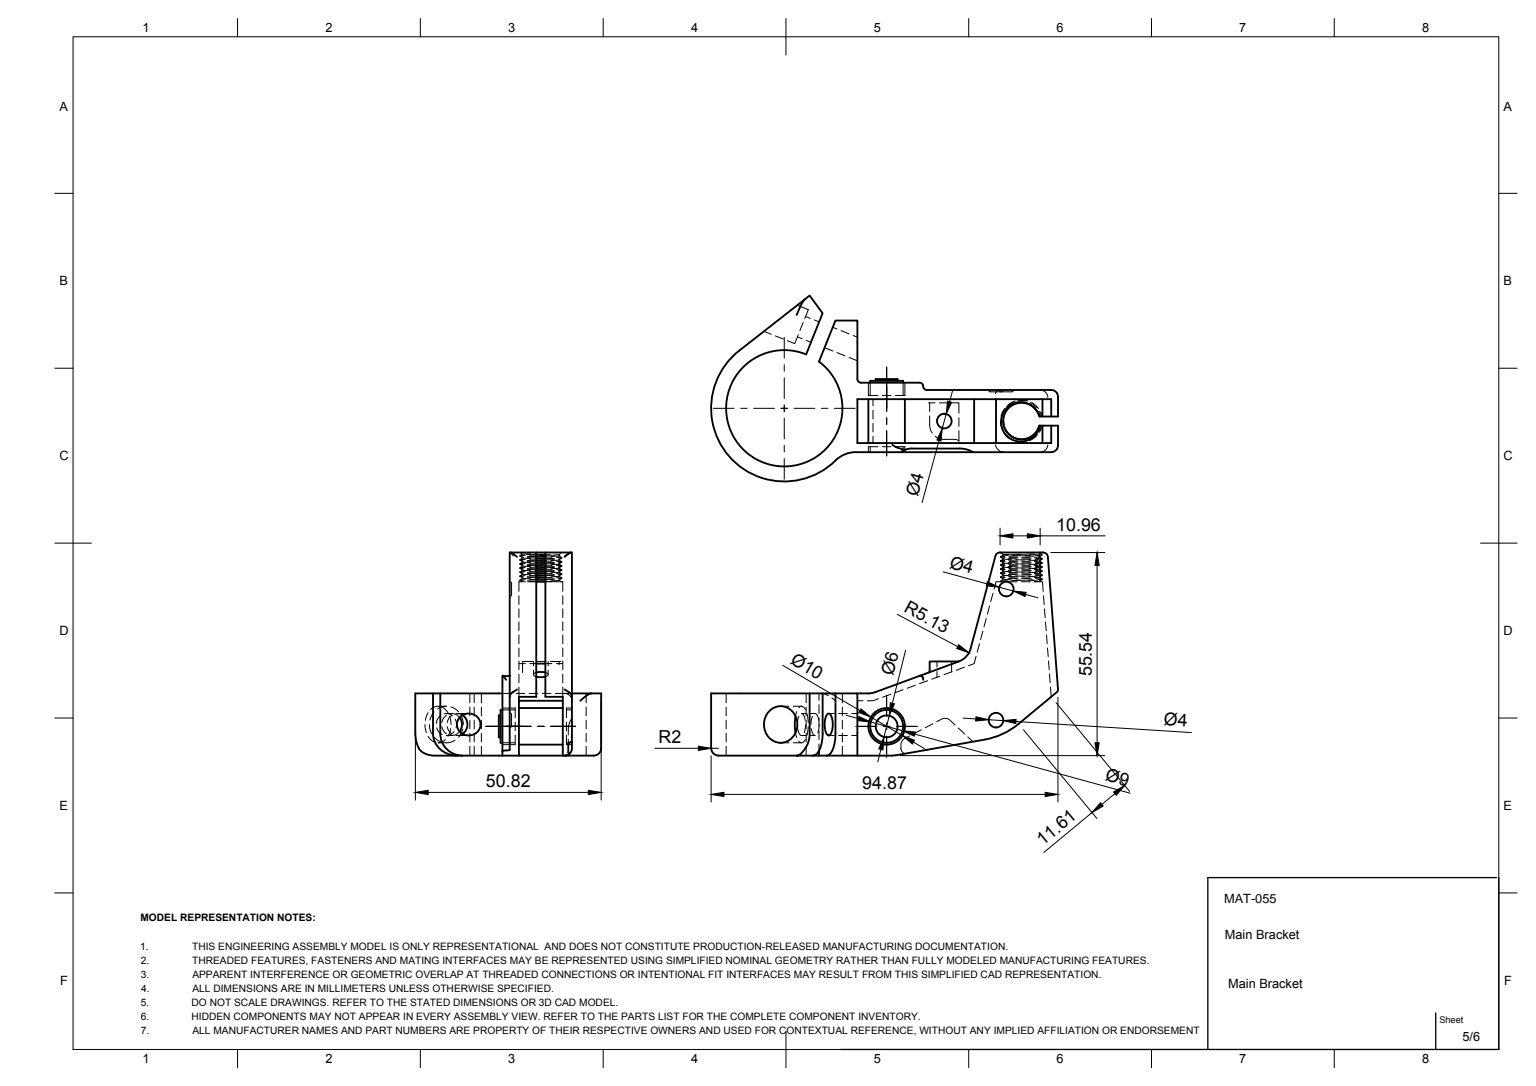
ISO-10303-21;
HEADER;
FILE_DESCRIPTION (('STEP AP214'),
    '1' );
FILE_NAME ('Main Bracket.step',
    '2026-10-30T09:41:00',
    ( '' ),
    ( '' ),
    'SwSTEP 2.0',
    'SolidWorks 2020',
    '' );
FILE_SCHEMA (( 'AUTOMOTIVE_DESIGN' ));
ENDSEC;

DATA;
#1=CARTESIAN_POINT ( 'NONE',  ( 110.9687390045248350, -9.868328341294098749, -11.32035403202665869 ) ) ;
#13=CARTESIAN_POINT ( 'NONE',  ( 69.69189222814998175, -41.76310523276723785, -24.39321520033831447 ) ) ;
#21=CARTESIAN_POINT ( 'NONE',  ( 106.2459265045248173, -7.250697342233347165, -19.15521520033831138 ) ) ;
#24=ORIENTED_EDGE ( 'NONE', *, *, #31128, .T. ) ;
#26=CYLINDRICAL_SURFACE ( 'NONE', #29939, 3.000000000000002665 ) ;
#41=CARTESIAN_POINT ( 'NONE',  ( 116.0834518517486771, -0.01906416985213849058, -12.14321520033831625 ) ) ;
#42=CARTESIAN_POINT ( 'NONE',  ( 106.5237390045248418, 0.8980012041604421569, -15.77991374673208469 ) ) ;
#43=CARTESIAN_POINT ( 'NONE',  ( 107.8433483795247838, -8.402594152722688392, -16.93181055722141792 ) ) ;
#44=CARTESIAN_POINT ( 'NONE',  ( 105.4819421295248247, 0.8980012041604618078, -13.39321520033831447 ) ) ;
#47=ORIENTED_EDGE ( 'NONE', *, *, #34668, .T. ) ;
#49=CARTESIAN_POINT ( 'NONE',  ( 111.3854577545248645, -7.250697342233347165, -7.631215200338321125 ) ) ;
#50=DIRECTION ( 'NONE',  ( 0.000000000000000000, 0.000000000000000000, -1.000000000000000000 ) ) ;
#55=CARTESIAN_POINT ( 'NONE',  ( 116.0388171295248014, -10.62599879583958540, -13.39321520033831447 ) ) ;
#56=CARTESIAN_POINT ( 'NONE',  ( 106.8710046295248759, -4.863998795839590272, -7.631215200338315796 ) ) ;
#57=ORIENTED_EDGE ( 'NONE', *, *, #39925, .T. ) ;
#62=CARTESIAN_POINT ( 'NONE',  ( 115.7610046295247912, -4.863998795839590272, -7.631215200338315796 ) ) ;
#63=CARTESIAN_POINT ( 'NONE',  ( 108.3295202545248657, 0.1403307496149616695, -11.32035403202665336 ) ) ;
#74=CARTESIAN_POINT ( 'NONE',  ( 112.6356140045247827, 0.1403307496149616695, -15.46607636864997204 ) ) ;
#85=CARTESIAN_POINT ( 'NONE',  ( 106.4542858795248179, -8.402594152722688392, -9.854619843455216355 ) ) ;
#88=AXIS2_PLACEMENT_3D ( 'NONE', #42203, #35787, #10965 ) ;
#91=CARTESIAN_POINT ( 'NONE',  ( 78.69189222814998175, -49.76310523276723785, -23.89321520033831803 ) ) ;
#92=ORIENTED_EDGE ( 'NONE', *, *, #23975, .F. ) ;
#96=CARTESIAN_POINT ( 'NONE',  ( 85.28386362106600416, -27.88924328735366132, -8.828750294274950505 ) ) ;
#98=EDGE_CURVE ( 'NONE', #12720, #5950, #1643, .T. ) ;
#100=ORIENTED_EDGE ( 'NONE', *, *, #14497, .T. ) ;
#103=CARTESIAN_POINT ( 'NONE',  ( 111.6632702545248605, -10.62599879583958717, -15.77991374673208469 ) ) ;
#108=CARTESIAN_POINT ( 'NONE',  ( 108.5378796295247810, -4.863998795839590272, -8.388885654883775800 ) ) ;
#109=DIRECTION ( 'NONE',  ( -1.000000000000000000, 0.000000000000000000, 0.000000000000000000 ) ) ;
#110=CARTESIAN_POINT ( 'NONE',  ( 109.2294422165998071, -3.102175910333654585, -18.18453611788106983 ) ) ;
#113=CARTESIAN_POINT ( 'NONE',  ( 107.0099108795247815, -8.938348069036489818, -9.318865927141430916 ) ) ;
#114=CARTESIAN_POINT ( 'NONE',  ( 115.2748327545248657, -6.936859964151250502, -8.388885654883777576 ) ) ;
#115=CARTESIAN_POINT ( 'NONE',  ( 111.3854577545248645, -7.250697342233347165, -7.631215200338321125 ) ) ;
#126=EDGE_CURVE ( 'NONE', #5046, #36034, #30866, .T. ) ;
#132=CARTESIAN_POINT ( 'NONE',  ( 114.7192077545248594, -7.250697342233347165, -7.631215200338321125 ) ) ;
#141=CARTESIAN_POINT ( 'NONE',  ( 111.1767004682428848, 0.5115630086001619059, -14.64321520033833757 ) ) ;
#142=CARTESIAN_POINT ( 'NONE',  ( 115.6915515045247531, -6.936859964151250502, -18.39754474579286025 ) ) ;
#148=ORIENTED_EDGE ( 'NONE', *, *, #1596, .T. ) ;
#155=CARTESIAN_POINT ( 'NONE',  ( 112.5661608795247872, -8.938348069036489818, -9.318865927141430916 ) ) ;
#158=CARTESIAN_POINT ( 'NONE',  ( 109.2294420414169451, -0.008529726858385754465, -11.21375788622608560 ) ) ;
#160=CARTESIAN_POINT ( 'NONE',  ( 107.0793640045248196, 0.1403307496149616695, -15.46607636864997204 ) ) ;
#164=CARTESIAN_POINT ( 'NONE',  ( 108.8851452545248151, 0.8980012041604421569, -11.00651665394454071 ) ) ;
#165=DIRECTION ( 'NONE',  ( -0.9970811988817434024, 0.07634843047859724008, 0.000000000000000000 ) ) ;
#174=CARTESIAN_POINT ( 'NONE',  ( 108.1906140045248037, 0.1403307496149616695, -15.46607636864997204 ) ) ;
#177=EDGE_LOOP ( 'NONE', ( #36537, #100, #20372, #6347 ) ) ;
#182=EDGE_LOOP ( 'NONE', ( #10317, #8710, #12538, #23742 ) ) ;
#183=CARTESIAN_POINT ( 'NONE',  ( 107.3571765045248299, -2.791137627527939813, -8.388885654883777576 ) ) ;
#202=CARTESIAN_POINT ( 'NONE',  ( 106.8015515045248378, -2.477300249445798297, -7.631215200338321125 ) ) ;
#212=EDGE_CURVE ( 'NONE', #32579, #21740, #16699, .T. ) ;
#213=CARTESIAN_POINT ( 'NONE',  ( 74.69189222814998175, -41.76310523276723785, -7.393215200338315363 ) ) ;
#217=CARTESIAN_POINT ( 'NONE',  ( 110.5520202545248054, 0.1403307496149616695, -11.32035403202665336 ) ) ;
#227=CYLINDRICAL_SURFACE ( 'NONE', #9190, 4.000000000000000000 ) ;
#229=ORIENTED_EDGE ( 'NONE', *, *, #20701, .T. ) ;
#231=CARTESIAN_POINT ( 'NONE',  ( 70.19189222814998175, -75.31442247550839397, -37.94335727672635983 ) ) ;
#235=ORIENTED_EDGE ( 'NONE', *, *, #33948, .T. ) ;
#236=ADVANCED_FACE ( 'NONE', ( #2543, #19428 ), #16245, .T. ) ;
#241=CARTESIAN_POINT ( 'NONE',  ( 77.77634386988368931, 3.254514819260763581, -19.39321520033831447 ) ) ;
#242=CARTESIAN_POINT ( 'NONE',  ( 110.1353015045248469, -2.477300249445798297, -7.631215200338321125 ) ) ;
#261=DIRECTION ( 'NONE',  ( 1.000000000000000000, 0.000000000000000000, 0.000000000000000000 ) ) ;
#262=CARTESIAN_POINT ( 'NONE',  ( 113.1217858795247935, -8.402594152722688392, -9.854619843455216355 ) ) ;
#264=CARTESIAN_POINT ( 'NONE',  ( 108.3989733795247759, -1.325403438956436419, -9.854619843455211026 ) ) ;
#265=CARTESIAN_POINT ( 'NONE',  ( 113.7468640045248236, 0.1403307496149616695, -15.46607636864997204 ) ) ;
#268=EDGE_LOOP ( 'NONE', ( #6034, #39667, #9832, #29930 ) ) ;
#270=CARTESIAN_POINT ( 'NONE',  ( 110.9687390045248350, 0.8980012041604421569, -15.77991374673208469 ) ) ;
#277=CARTESIAN_POINT ( 'NONE',  ( 115.2748327545248657, -2.477300249445798297, -19.15521520033831138 ) ) ;
#278=CARTESIAN_POINT ( 'NONE',  ( 114.7886608795247696, -1.325403438956436419, -16.93181055722141792 ) ) ;
#284=CARTESIAN_POINT ( 'NONE',  ( 113.3995983795247895, -0.7896495226426338832, -9.318865927141430916 ) ) ;
#285=CARTESIAN_POINT ( 'NONE',  ( 107.4960827545248350, -6.936859964151250502, -8.388885654883777576 ) ) ;
#289=ORIENTED_EDGE ( 'NONE', *, *, #44643, .F. ) ;
#295=EDGE_CURVE ( 'NONE', #33939, #11904, #44743, .T. ) ;
#296=CARTESIAN_POINT ( 'NONE',  ( 106.5931921295248372, 0.8980012041604618078, -13.39321520033831447 ) ) ;
#297=CARTESIAN_POINT ( 'NONE',  ( 110.9687390045248350, -9.868328341294098749, -11.32035403202665869 ) ) ;
#306=DIRECTION ( 'NONE',  ( 0.000000000000000000, 0.7876185884367599144, -0.6161630946014909904 ) ) ;
#307=CARTESIAN_POINT ( 'NONE',  ( 106.5931921295248372, -9.868328341294093420, -13.39321520033831447 ) ) ;
#316=LINE ( 'NONE', #14010, #39137 ) ;
#321=LINE ( 'NONE', #35409, #15967 ) ;
#322=CARTESIAN_POINT ( 'NONE',  ( 112.8439733795247832, -8.938348069036489818, -17.46756447353520159 ) ) ;
#327=CARTESIAN_POINT ( 'NONE',  ( 111.7327233795247849, -1.325403438956533675, -9.854619843455175499 ) ) ;
#328=CARTESIAN_POINT ( 'NONE',  ( 110.2047546295247855, -4.863998795839590272, -18.39754474579285315 ) ) ;
#331=CARTESIAN_POINT ( 'NONE',  ( 109.2294421564239713, -3.315832619059893460, -18.27430022661860676 ) ) ;
#333=CARTESIAN_POINT ( 'NONE',  ( 106.0375671295248310, -10.62599879583958540, -13.39321520033831447 ) ) ;
#334=CARTESIAN_POINT ( 'NONE',  ( 114.4413952545248350, -9.868328341294098749, -15.46607636864997204 ) ) ;
#335=CARTESIAN_POINT ( 'NONE',  ( 108.1906140045248463, -10.62599879583958717, -11.00651665394454604 ) ) ;
#336=CARTESIAN_POINT ( 'NONE',  ( 66.06194382436763135, -14.97931106434683635, -7.393215200338315363 ) ) ;
#338=CARTESIAN_POINT ( 'NONE',  ( 71.37572422742091760, -11.86958442233774313, -21.89321520033831447 ) ) ;
#341=EDGE_CURVE ( 'NONE', #2225, #6245, #14383, .T. ) ;
#351=EDGE_CURVE ( 'NONE', #29699, #30236, #16925, .T. ) ;
#353=CARTESIAN_POINT ( 'NONE',  ( 107.9128015045248219, -2.477300249445798297, -7.631215200338321125 ) ) ;
#354=B_SPLINE_CURVE_WITH_KNOTS ( 'NONE', 3,
 ( #21953, #36072, #29691, #15790, #25607, #25823, #22401, #36296, #1419, #40183 ),
 .UNSPECIFIED., .F., .F.,
 ( 4, 2, 2, 2, 4 ),
 ( 0.000000000000000000, 0.2500000000000000000, 0.5000000000000000000, 0.7500000000000000000, 1.000000000000000000 ),
 .UNSPECIFIED. ) ;
#356=FACE_OUTER_BOUND ( 'NONE', #44787, .T. ) ;
#360=CARTESIAN_POINT ( 'NONE',  ( 90.93679655599923706, -18.80572346544368756, -20.89321520033831447 ) ) ;
#363=CARTESIAN_POINT ( 'NONE',  ( 112.3324666496844912, 0.5600166689815611054, -12.14321520033829849 ) ) ;
#364=CARTESIAN_POINT ( 'NONE',  ( 114.4413952545248350, -9.868328341294098749, -15.46607636864997204 ) ) ;
#376=CARTESIAN_POINT ( 'NONE',  ( 116.3860827545247787, -6.936859964151250502, -8.388885654883777576 ) ) ;
#380=CARTESIAN_POINT ( 'NONE',  ( 114.3024890045248156, 0.8980012041604421569, -15.77991374673208469 ) ) ;
#386=CARTESIAN_POINT ( 'NONE',  ( 108.3295202545248657, 0.1403307496149616695, -11.32035403202665336 ) ) ;
#387=CARTESIAN_POINT ( 'NONE',  ( 117.1746850318387203, 1.411517391187495640, -21.51583517613059016 ) ) ;
#390=CARTESIAN_POINT ( 'NONE',  ( 112.4272546295247821, -4.863998795839590272, -7.631215200338315796 ) ) ;
#393=CARTESIAN_POINT ( 'NONE',  ( 117.2294421295247844, 1.035107641088057973, -21.89321520033831447 ) ) ;
#400=CARTESIAN_POINT ( 'NONE',  ( 106.7320983795247855, -8.402594152722688392, -16.93181055722141792 ) ) ;
#408=VERTEX_POINT ( 'NONE', #41764 ) ;
#409=CARTESIAN_POINT ( 'NONE',  ( 107.1488171295247867, 0.1403307496149613920, -13.39321520033831447 ) ) ;
#424=VERTEX_POINT ( 'NONE', #34228 ) ;
#426=CARTESIAN_POINT ( 'NONE',  ( 113.6079577545248043, -2.791137627527939813, -18.39754474579286025 ) ) ;
#428=DIRECTION ( 'NONE',  ( 8.673617379884029556E-16, 1.000000000000000000, 0.000000000000000000 ) ) ;
#438=CARTESIAN_POINT ( 'NONE',  ( 110.2742077545248094, -2.791137627527939813, -18.39754474579286025 ) ) ;
#449=CARTESIAN_POINT ( 'NONE',  ( 66.82415148905926117, -40.21211973637273474, -4.893215200338314474 ) ) ;
#450=CARTESIAN_POINT ( 'NONE',  ( 109.9649712410415816, 0.7607806665038616689, -12.14321520033831625 ) ) ;
#461=CARTESIAN_POINT ( 'NONE',  ( 108.8851452545248151, 0.8980012041604421569, -11.00651665394454071 ) ) ;
#465=AXIS2_PLACEMENT_3D ( 'NONE', #17179, #9891, #34693 ) ;
#466=CARTESIAN_POINT ( 'NONE',  ( 69.69189222814998175, -41.76310523276723785, -4.893215200338314474 ) ) ;
#484=CARTESIAN_POINT ( 'NONE',  ( 113.2606921295247702, -9.868328341294093420, -13.39321520033831447 ) ) ;
#485=CARTESIAN_POINT ( 'NONE',  ( 110.1353015045248469, -6.936859964151250502, -18.39754474579286025 ) ) ;
#486=CARTESIAN_POINT ( 'NONE',  ( 115.6915515045247531, -6.936859964151250502, -18.39754474579286025 ) ) ;
#492=CARTESIAN_POINT ( 'NONE',  ( 112.7745202545247878, -10.62599879583958717, -15.77991374673208469 ) ) ;
#499=CARTESIAN_POINT ( 'NONE',  ( 115.6915515045247531, -2.477300249445798297, -7.631215200338321125 ) ) ;
#500=CARTESIAN_POINT ( 'NONE',  ( 112.9134265045247645, -2.791137627527939813, -8.388885654883777576 ) ) ;
#506=CARTESIAN_POINT ( 'NONE',  ( 114.9970202545248412, -10.62599879583958717, -15.77991374673208469 ) ) ;
#507=CARTESIAN_POINT ( 'NONE',  ( 105.2041296295248287, -4.863998795839590272, -8.388885654883775800 ) ) ;
#520=CARTESIAN_POINT ( 'NONE',  ( 111.5938171295247940, 0.1403307496149613920, -13.39321520033831447 ) ) ;
#526=DIRECTION ( 'NONE',  ( 1.000000000000000000, 0.000000000000000000, 0.000000000000000000 ) ) ;
#527=EDGE_CURVE ( 'NONE', #24697, #26785, #16321, .T. ) ;
#529=VERTEX_POINT ( 'NONE', #27409 ) ;
#533=CARTESIAN_POINT ( 'NONE',  ( 112.4967077545247633, -7.250697342233347165, -7.631215200338321125 ) ) ;
#534=CIRCLE ( 'NONE', #35440, 3.000000000000002665 ) ;
#541=CARTESIAN_POINT ( 'NONE',  ( 115.4137390045248566, 0.8980012041604421569, -15.77991374673208469 ) ) ;
#542=CARTESIAN_POINT ( 'NONE',  ( 85.65290454163996969, -26.88367880166602220, -8.452090709015315895 ) ) ;
#548=CARTESIAN_POINT ( 'NONE',  ( 113.1912390045248031, 0.8980012041604421569, -15.77991374673208469 ) ) ;
#552=CIRCLE ( 'NONE', #2726, 2.000000000000001776 ) ;
#555=CARTESIAN_POINT ( 'NONE',  ( 110.3436608795247764, -1.325403438956436419, -16.93181055722141792 ) ) ;
#558=CARTESIAN_POINT ( 'NONE',  ( 109.2294414898113217, -8.099164058012600975, -17.65094077544404882 ) ) ;
#562=CARTESIAN_POINT ( 'NONE',  ( 111.2465515045248168, -2.477300249445798297, -7.631215200338321125 ) ) ;
#574=VERTEX_POINT ( 'NONE', #3001 ) ;
#579=CARTESIAN_POINT ( 'NONE',  ( 108.2600671295247992, -10.62599879583958540, -13.39321520033831447 ) ) ;
#582=CARTESIAN_POINT ( 'NONE',  ( 116.4555358795247884, -8.402594152722688392, -9.854619843455216355 ) ) ;
#588=CARTESIAN_POINT ( 'NONE',  ( 112.4290776191212871, 0.4261359969231631739, -12.14321520033833046 ) ) ;
#589=CARTESIAN_POINT ( 'NONE',  ( 114.8581140045248361, 0.1403307496149616695, -15.46607636864997204 ) ) ;
#598=ORIENTED_EDGE ( 'NONE', *, *, #44306, .T. ) ;
#601=CARTESIAN_POINT ( 'NONE',  ( 113.1912390045248031, -9.868328341294098749, -11.32035403202665869 ) ) ;
#605=CARTESIAN_POINT ( 'NONE',  ( 114.8581140045248361, -10.62599879583958717, -11.00651665394454604 ) ) ;
#609=CARTESIAN_POINT ( 'NONE',  ( 109.2293317483792805, -6.895714903177337263, -8.103635009265300226 ) ) ;
#611=CARTESIAN_POINT ( 'NONE',  ( 114.7192077545248594, -7.250697342233347165, -7.631215200338321125 ) ) ;
#612=CARTESIAN_POINT ( 'NONE',  ( 116.4741944465760213, 2.215541826465470709, -20.45829475731958169 ) ) ;
#615=CARTESIAN_POINT ( 'NONE',  ( 111.5243640045248412, -10.62599879583958717, -11.00651665394454604 ) ) ;
#625=CARTESIAN_POINT ( 'NONE',  ( 113.1217858795247935, -0.7896495226426338832, -17.46756447353520159 ) ) ;
#633=CARTESIAN_POINT ( 'NONE',  ( 116.1777233795247781, -8.938348069036489818, -17.46756447353520159 ) ) ;
#639=CARTESIAN_POINT ( 'NONE',  ( 143.3676850761856940, -63.77884951796256274, -31.62409037935697143 ) ) ;
#646=CARTESIAN_POINT ( 'NONE',  ( 111.6379010812576809, -0.01829820670803256055, -12.14321520033831625 ) ) ;
#648=ORIENTED_EDGE ( 'NONE', *, *, #42605, .T. ) ;
#650=CARTESIAN_POINT ( 'NONE',  ( 111.8716296295247901, -4.863998795839590272, -8.388885654883775800 ) ) ;
#654=CARTESIAN_POINT ( 'NONE',  ( 82.42994493343583429, -31.76310523276723430, -22.89321520033831803 ) ) ;
#656=ORIENTED_EDGE ( 'NONE', *, *, #15376, .T. ) ;
#658=VECTOR ( 'NONE', #32222, 1000.000000000000000 ) ;
#662=CARTESIAN_POINT ( 'NONE',  ( 112.7050671295247923, 0.1403307496149613920, -13.39321520033831447 ) ) ;
#666=DIRECTION ( 'NONE',  ( 0.000000000000000000, 0.000000000000000000, 1.000000000000000000 ) ) ;
#675=CARTESIAN_POINT ( 'NONE',  ( 114.9970202545248412, 0.1403307496149616695, -11.32035403202665336 ) ) ;
#678=ORIENTED_EDGE ( 'NONE', *, *, #1567, .T. ) ;
#686=AXIS2_PLACEMENT_3D ( 'NONE', #16548, #16776, #44363 ) ;
#699=ORIENTED_EDGE ( 'NONE', *, *, #22024, .F. ) ;
#700=CARTESIAN_POINT ( 'NONE',  ( 112.0109337908067886, 0.5115630086001619059, -12.14321520033831625 ) ) ;
#701=CARTESIAN_POINT ( 'NONE',  ( 115.9693640045247776, -10.62599879583958717, -11.00651665394454604 ) ) ;
#702=CARTESIAN_POINT ( 'NONE',  ( 114.3719421295247827, -9.868328341294093420, -13.39321520033831447 ) ) ;
#703=CARTESIAN_POINT ( 'NONE',  ( 110.4131140045248287, 0.1403307496149616695, -15.46607636864997204 ) ) ;
#704=CARTESIAN_POINT ( 'NONE',  ( 113.6079577545248043, -2.791137627527939813, -18.39754474579286025 ) ) ;
#707=EDGE_LOOP ( 'NONE', ( #22175, #39798, #28141, #15557 ) ) ;
#709=CARTESIAN_POINT ( 'NONE',  ( 109.2324108795247923, -8.938348069036489818, -9.318865927141430916 ) ) ;
#710=FACE_OUTER_BOUND ( 'NONE', #10794, .T. ) ;
#714=CARTESIAN_POINT ( 'NONE',  ( 115.3442858795247759, -0.7896495226426338832, -17.46756447353520159 ) ) ;
#715=CARTESIAN_POINT ( 'NONE',  ( 110.0658483795247804, -8.402594152722688392, -16.93181055722141792 ) ) ;
#721=CARTESIAN_POINT ( 'NONE',  ( 83.84865386347668448, -25.99489077589588604, -15.39321520033831625 ) ) ;
#727=AXIS2_PLACEMENT_3D ( 'NONE', #17094, #41489, #30986 ) ;
#733=CARTESIAN_POINT ( 'NONE',  ( 110.2047546295247855, -4.863998795839590272, -18.39754474579285315 ) ) ;
#740=ADVANCED_FACE ( 'NONE', ( #42651 ), #25772, .F. ) ;
#745=CARTESIAN_POINT ( 'NONE',  ( 112.4272546295247821, -4.863998795839590272, -7.631215200338315796 ) ) ;
#755=CARTESIAN_POINT ( 'NONE',  ( 116.5249890045247980, 0.8980012041604421569, -15.77991374673208469 ) ) ;
#758=TOROIDAL_SURFACE ( 'NONE', #8032, 1.500000000000000000, 0.5000000000000000000 ) ;
#760=DIRECTION ( 'NONE',  ( 1.000000000000000000, 0.000000000000000000, 0.000000000000000000 ) ) ;
#761=CARTESIAN_POINT ( 'NONE',  ( 111.7327233795247849, -8.938348069036489818, -17.46756447353520159 ) ) ;
#765=CARTESIAN_POINT ( 'NONE',  ( 71.37572422742091760, -11.86958442233774313, -21.39321520033831447 ) ) ;
#766=CARTESIAN_POINT ( 'NONE',  ( 106.3848327545248651, -6.936859964151250502, -8.388885654883777576 ) ) ;
#770=CARTESIAN_POINT ( 'NONE',  ( 109.2294595382483777, -2.917851662749194386, -18.10281666216439689 ) ) ;
#774=CARTESIAN_POINT ( 'NONE',  ( 114.1635827545248389, -6.936859964151250502, -8.388885654883777576 ) ) ;
#781=EDGE_LOOP ( 'NONE', ( #39157, #35315, #35728, #29011 ) ) ;
#794=CARTESIAN_POINT ( 'NONE',  ( 111.3854577545248645, -7.250697342233347165, -7.631215200338321125 ) ) ;
#801=CARTESIAN_POINT ( 'NONE',  ( 113.3301452545248083, -9.868328341294098749, -15.46607636864997204 ) ) ;
#805=CARTESIAN_POINT ( 'NONE',  ( 111.4567791257774729, 0.2334052082820642360, -12.14321520033830026 ) ) ;
#806=DIRECTION ( 'NONE',  ( 1.000000000000000000, 0.000000000000000000, 0.000000000000000000 ) ) ;
#807=CARTESIAN_POINT ( 'NONE',  ( 112.7050671295247923, 0.1403307496149613920, -13.39321520033831447 ) ) ;
#811=DIRECTION ( 'NONE',  ( 0.000000000000000000, 0.000000000000000000, 1.000000000000000000 ) ) ;
#816=VERTEX_POINT ( 'NONE', #43550 ) ;
#819=CARTESIAN_POINT ( 'NONE',  ( 114.0246765045248196, -2.791137627527939813, -8.388885654883777576 ) ) ;
#822=CARTESIAN_POINT ( 'NONE',  ( 85.43848064358274996, -28.59459646149706913, -9.352541679919285755 ) ) ;
#823=CARTESIAN_POINT ( 'NONE',  ( 113.3301452545248083, 0.8980012041604421569, -11.00651665394454071 ) ) ;
#828=CARTESIAN_POINT ( 'NONE',  ( 109.2293785907020407, -6.437107504569898886, -7.971344053030498422 ) ) ;
#830=CARTESIAN_POINT ( 'NONE',  ( 106.8710046295248759, -4.863998795839590272, -18.39754474579285315 ) ) ;
#832=CARTESIAN_POINT ( 'NONE',  ( 62.57015527438819191, -24.33598972801448923, -6.893215200338315363 ) ) ;
#835=CARTESIAN_POINT ( 'NONE',  ( 110.1353015045248469, -2.477300249445798297, -7.631215200338321125 ) ) ;
#845=CARTESIAN_POINT ( 'NONE',  ( 114.1635827545248389, -2.477300249445798297, -19.15521520033831138 ) ) ;
#862=CARTESIAN_POINT ( 'NONE',  ( 64.12124478315966769, -35.39759648474613840, -5.871463680831255694 ) ) ;
#875=CARTESIAN_POINT ( 'NONE',  ( 111.4549108795247747, -1.325403438956436419, -16.93181055722141792 ) ) ;
#878=CIRCLE ( 'NONE', #26376, 20.00000000000000355 ) ;
#879=CARTESIAN_POINT ( 'NONE',  ( 85.07488655036617331, -28.45866502056250980, -7.893215200338303816 ) ) ;
#886=CARTESIAN_POINT ( 'NONE',  ( 109.2294421295247844, -49.76310523276723785, -7.393215200338315363 ) ) ;
#887=CARTESIAN_POINT ( 'NONE',  ( 112.6356140045247827, 0.1403307496149616695, -15.46607636864997204 ) ) ;
#892=DIRECTION ( 'NONE',  ( 0.9659258262890689783, 0.2588190451025185190, 0.000000000000000000 ) ) ;
#899=CARTESIAN_POINT ( 'NONE',  ( 72.75524511225664526, -29.99489077589588959, -18.39321520033831803 ) ) ;
#901=EDGE_LOOP ( 'NONE', ( #39869, #4969 ) ) ;
#903=CARTESIAN_POINT ( 'NONE',  ( 116.3166296295247832, -4.863998795839590272, -8.388885654883775800 ) ) ;
#906=EDGE_LOOP ( 'NONE', ( #19691, #14880 ) ) ;
#921=PLANE ( 'NONE',  #20121 ) ;
#925=CARTESIAN_POINT ( 'NONE',  ( 116.7068493634037480, -7.245760568235874999, -17.91803073691438897 ) ) ;
#930=VERTEX_POINT ( 'NONE', #30764 ) ;
#931=CARTESIAN_POINT ( 'NONE',  ( 111.8277378519202756, 0.2518737723193609224, -12.14321520033831625 ) ) ;
#933=CARTESIAN_POINT ( 'NONE',  ( 112.9134265045247645, -2.791137627527939813, -8.388885654883777576 ) ) ;
#934=CARTESIAN_POINT ( 'NONE',  ( 114.0246765045248196, -2.791137627527939813, -8.388885654883777576 ) ) ;
#940=CARTESIAN_POINT ( 'NONE',  ( 107.7044421295247929, 0.8980012041604618078, -13.39321520033831447 ) ) ;
#942=CARTESIAN_POINT ( 'NONE',  ( 69.69189222814998175, -41.76310523276723785, -4.893215200338314474 ) ) ;
#943=CARTESIAN_POINT ( 'NONE',  ( 109.2294421295247560, 0.08637466845215115152, -14.75790253999268131 ) ) ;
#947=CARTESIAN_POINT ( 'NONE',  ( 116.4555358795247884, -0.7896495226426338832, -17.46756447353520159 ) ) ;
#948=CARTESIAN_POINT ( 'NONE',  ( 113.8163171295247764, 0.1403307496149613920, -13.39321520033831447 ) ) ;
#959=EDGE_LOOP ( 'NONE', ( #4440, #25894, #33864, #38580, #39938 ) ) ;
#967=CARTESIAN_POINT ( 'NONE',  ( 115.2748327545248657, -2.477300249445798297, -19.15521520033831138 ) ) ;
#970=VERTEX_POINT ( 'NONE', #23714 ) ;
#980=CARTESIAN_POINT ( 'NONE',  ( 111.9410827545248708, -2.477300249445798297, -19.15521520033831138 ) ) ;
#981=CIRCLE ( 'NONE', #8996, 1.500000000000001332 ) ;
#988=CARTESIAN_POINT ( 'NONE',  ( 115.9693640045247776, -10.62599879583958717, -11.00651665394454604 ) ) ;
#990=CARTESIAN_POINT ( 'NONE',  ( 117.1500671295247713, 0.1403307496149613920, -13.39321520033831447 ) ) ;
#991=FACE_OUTER_BOUND ( 'NONE', #6590, .T. ) ;
#996=CARTESIAN_POINT ( 'NONE',  ( 113.5385046295247804, -4.863998795839590272, -7.631215200338315796 ) ) ;
#1001=CARTESIAN_POINT ( 'NONE',  ( 90.93679655599923706, -18.80572346544368756, -4.893215200338314474 ) ) ;
#1004=CARTESIAN_POINT ( 'NONE',  ( 109.2294436890326779, -7.171314547180734245, -18.16325295140885387 ) ) ;
#1007=CARTESIAN_POINT ( 'NONE',  ( 115.6915515045247531, -6.936859964151250502, -18.39754474579286025 ) ) ;
#1008=CARTESIAN_POINT ( 'NONE',  ( 113.8857702545248003, 0.1403307496149616695, -11.32035403202665336 ) ) ;
#1014=ORIENTED_EDGE ( 'NONE', *, *, #2177, .F. ) ;
#1023=CARTESIAN_POINT ( 'NONE',  ( 110.6909265045248247, -7.250697342233347165, -19.15521520033831138 ) ) ;
#1025=CARTESIAN_POINT ( 'NONE',  ( 116.6447457829843870, 0.6362173239733635022, -14.64321520033831447 ) ) ;
#1026=EDGE_CURVE ( 'NONE', #25605, #31523, #7613, .T. ) ;
#1027=CARTESIAN_POINT ( 'NONE',  ( 113.5385046295247804, -4.863998795839590272, -18.39754474579285315 ) ) ;
#1033=CARTESIAN_POINT ( 'NONE',  ( 108.8156921295247912, -9.868328341294093420, -13.39321520033831447 ) ) ;
#1045=CARTESIAN_POINT ( 'NONE',  ( 116.5249890045247980, -9.868328341294098749, -11.32035403202665869 ) ) ;
#1049=CARTESIAN_POINT ( 'NONE',  ( 85.01908738548678457, -29.61018707541026629, -10.68033442898624941 ) ) ;
#1050=CARTESIAN_POINT ( 'NONE',  ( 107.9128015045248219, -2.477300249445798297, -7.631215200338321125 ) ) ;
#1054=CARTESIAN_POINT ( 'NONE',  ( 109.2294962932281095, -5.361490969279928187, -7.816834419629333119 ) ) ;
#1056=CARTESIAN_POINT ( 'NONE',  ( 106.1070202545248407, 0.1403307496149616695, -11.32035403202665336 ) ) ;
#1057=ADVANCED_FACE ( 'NONE', ( #37605 ), #20955, .T. ) ;
#1058=CARTESIAN_POINT ( 'NONE',  ( 116.8894182543351405, 1.911972990205162981, -21.02721497854282973 ) ) ;
#1059=CARTESIAN_POINT ( 'NONE',  ( 83.41361896732357195, -32.98529496753769052, -22.17982263453885494 ) ) ;
#1062=CARTESIAN_POINT ( 'NONE',  ( 110.9687390045248350, 0.8980012041604421569, -15.77991374673208469 ) ) ;
#1074=AXIS2_PLACEMENT_3D ( 'NONE', #18198, #11365, #39169 ) ;
#1075=CARTESIAN_POINT ( 'NONE',  ( 113.6079577545248043, -7.250697342233347165, -7.631215200338321125 ) ) ;
#1082=ORIENTED_EDGE ( 'NONE', *, *, #17680, .F. ) ;
#1088=CARTESIAN_POINT ( 'NONE',  ( 64.98570645825515157, -35.85007757536534001, -5.722960826911935861 ) ) ;
#1090=LINE ( 'NONE', #639, #17142 ) ;
#1092=AXIS2_PLACEMENT_3D ( 'NONE', #41329, #44293, #41546 ) ;
#1099=VECTOR ( 'NONE', #43138, 1000.000000000000114 ) ;
#1103=CARTESIAN_POINT ( 'NONE',  ( 115.4137390045248566, -9.868328341294098749, -11.32035403202665869 ) ) ;
#1104=CARTESIAN_POINT ( 'NONE',  ( 86.84453910206313765, -17.83168818462593919, -7.393215200338315363 ) ) ;
#1107=CARTESIAN_POINT ( 'NONE',  ( 117.1500671295247713, 0.1403307496149613920, -13.39321520033831447 ) ) ;
#1114=CARTESIAN_POINT ( 'NONE',  ( 106.8710046295248759, -4.863998795839590272, -18.39754474579285315 ) ) ;
#1115=ORIENTED_EDGE ( 'NONE', *, *, #34492, .T. ) ;
#1117=DIRECTION ( 'NONE',  ( -0.3445294493088594256, -0.9387755102040817867, 2.988316619407199162E-16 ) ) ;
#1124=VERTEX_POINT ( 'NONE', #38050 ) ;
#1130=EDGE_LOOP ( 'NONE', ( #25260, #4271, #38542, #14867, #38250, #1878, #17115, #2078 ) ) ;
#1131=CARTESIAN_POINT ( 'NONE',  ( 61.69084222814998242, 7.836001204160461420, -12.14321520033831625 ) ) ;
#1133=AXIS2_PLACEMENT_3D ( 'NONE', #30931, #41654, #44854 ) ;
#1140=CARTESIAN_POINT ( 'NONE',  ( 79.13619734047924226, 4.894407596166499452, -20.89842468304581047 ) ) ;
#1148=CARTESIAN_POINT ( 'NONE',  ( 116.6385761563547447, -9.481945103229687533, -15.42247872983044665 ) ) ;
#1154=CARTESIAN_POINT ( 'NONE',  ( 114.5066521944298756, 0.6269505268395592079, -12.14321520033831625 ) ) ;
#1155=CARTESIAN_POINT ( 'NONE',  ( 116.1777233795247781, -8.938348069036489818, -17.46756447353520159 ) ) ;
#1157=CARTESIAN_POINT ( 'NONE',  ( 115.0664733795247798, -1.325403438956436419, -9.854619843455211026 ) ) ;
#1158=CARTESIAN_POINT ( 'NONE',  ( 114.4413952545248350, -9.868328341294098749, -15.46607636864997204 ) ) ;
#1163=CARTESIAN_POINT ( 'NONE',  ( 107.0099108795247815, -8.938348069036489818, -9.318865927141430916 ) ) ;
#1171=CARTESIAN_POINT ( 'NONE',  ( 111.3854577545248645, -7.250697342233347165, -7.631215200338321125 ) ) ;
#1172=CARTESIAN_POINT ( 'NONE',  ( 110.2047546295247855, -4.863998795839590272, -18.39754474579285315 ) ) ;
#1185=B_SPLINE_CURVE_WITH_KNOTS ( 'NONE', 3,
 ( #39404, #4514, #28248, #24600 ),
 .UNSPECIFIED., .F., .F.,
 ( 4, 4 ),
 ( 0.005279168639414119624, 0.005761668442105720260 ),
 .UNSPECIFIED. ) ;
#1193=CARTESIAN_POINT ( 'NONE',  ( 114.7192077545248594, -7.250697342233347165, -7.631215200338321125 ) ) ;
#1196=ORIENTED_EDGE ( 'NONE', *, *, #31166, .F. ) ;
#1204=CARTESIAN_POINT ( 'NONE',  ( 62.03132163408040611, -65.45885774859658568, -44.53126419185489482 ) ) ;
#1205=CARTESIAN_POINT ( 'NONE',  ( 111.3854577545248645, -7.250697342233347165, -7.631215200338321125 ) ) ;
#1206=( BOUNDED_CURVE ( )  B_SPLINE_CURVE ( 3, ( #13133, #12913, #34310, #37964 ),
 .UNSPECIFIED., .F., .T. ) 
 B_SPLINE_CURVE_WITH_KNOTS ( ( 4, 4 ),
 ( 3.141592653589795336, 4.712388980384689674 ),
 .UNSPECIFIED. ) 
 CURVE ( )  GEOMETRIC_REPRESENTATION_ITEM ( )  RATIONAL_B_SPLINE_CURVE ( ( 1.000000000000000000, 0.8047378541243649375, 0.8047378541243649375, 1.000000000000000000 ) ) 
 REPRESENTATION_ITEM ( '' )  );
#1215=CARTESIAN_POINT ( 'NONE',  ( 114.7886608795247696, -8.938348069036489818, -9.318865927141430916 ) ) ;
#1218=ORIENTED_EDGE ( 'NONE', *, *, #5520, .T. ) ;
#1221=CARTESIAN_POINT ( 'NONE',  ( 106.3848327545248651, -2.477300249445798297, -19.15521520033831138 ) ) ;
#1225=CARTESIAN_POINT ( 'NONE',  ( 116.6426534889645552, -11.85006152547368430, -6.385399117676209713 ) ) ;
#1226=CARTESIAN_POINT ( 'NONE',  ( 107.4960827545248350, -6.936859964151250502, -8.388885654883777576 ) ) ;
#1229=CARTESIAN_POINT ( 'NONE',  ( 115.5212212410415873, 0.7607806665037644134, -12.14321520033829493 ) ) ;
#1230=CARTESIAN_POINT ( 'NONE',  ( 109.2294382629313958, -10.31656828667767734, -14.31165057277949870 ) ) ;
#1233=CARTESIAN_POINT ( 'NONE',  ( 114.2330358795247776, -8.402594152722688392, -9.854619843455216355 ) ) ;
#1234=CARTESIAN_POINT ( 'NONE',  ( 113.5385046295247804, -4.863998795839590272, -18.39754474579285315 ) ) ;
#1237=DIRECTION ( 'NONE',  ( 0.000000000000000000, 0.000000000000000000, 1.000000000000000000 ) ) ;
#1240=ORIENTED_EDGE ( 'NONE', *, *, #25111, .F. ) ;
#1251=DIRECTION ( 'NONE',  ( 0.2588190451025126904, -0.9659258262890705327, 0.000000000000000000 ) ) ;
#1253=CARTESIAN_POINT ( 'NONE',  ( 114.9970202545248412, 0.1403307496149616695, -11.32035403202665336 ) ) ;
#1258=DIRECTION ( 'NONE',  ( 0.000000000000000000, 0.000000000000000000, 1.000000000000000000 ) ) ;
#1260=CARTESIAN_POINT ( 'NONE',  ( 111.6632702545248605, 0.1403307496149616695, -11.32035403202665336 ) ) ;
#1272=CARTESIAN_POINT ( 'NONE',  ( 112.6356140045247827, 0.1403307496149616695, -15.46607636864997204 ) ) ;
#1276=CARTESIAN_POINT ( 'NONE',  ( 85.90654841308125356, -27.46059110997621033, -8.671423226218806235 ) ) ;
#1277=CARTESIAN_POINT ( 'NONE',  ( 109.5796765045248122, -7.250697342233347165, -19.15521520033831138 ) ) ;
#1284=CARTESIAN_POINT ( 'NONE',  ( 114.3024890045248156, 0.8980012041604421569, -15.77991374673208469 ) ) ;
#1286=CARTESIAN_POINT ( 'NONE',  ( 82.57348731610973402, -31.56754274340543986, -22.29195438618578606 ) ) ;
#1289=CARTESIAN_POINT ( 'NONE',  ( 105.6208483795248299, -0.7896495226426338832, -9.318865927141430916 ) ) ;
#1299=CARTESIAN_POINT ( 'NONE',  ( 113.3301452545248083, 0.8980012041604421569, -11.00651665394454071 ) ) ;
#1301=CARTESIAN_POINT ( 'NONE',  ( 116.7898211891027671, -3.191637679206685618, -18.31208751218940733 ) ) ;
#1322=DIRECTION ( 'NONE',  ( 0.000000000000000000, 0.000000000000000000, -1.000000000000000000 ) ) ;
#1324=ORIENTED_EDGE ( 'NONE', *, *, #3945, .T. ) ;
#1326=CARTESIAN_POINT ( 'NONE',  ( 114.9970202545248412, 0.1403307496149616695, -11.32035403202665336 ) ) ;
#1327=DIRECTION ( 'NONE',  ( 0.000000000000000000, -0.3713878862591642460, 0.9284778069183722282 ) ) ;
#1333=DIRECTION ( 'NONE',  ( 1.000000000000000000, 0.000000000000000000, 0.000000000000000000 ) ) ;
#1336=CARTESIAN_POINT ( 'NONE',  ( 107.0099108795247815, -1.325403438956436419, -16.93181055722141792 ) ) ;
#1337=EDGE_CURVE ( 'NONE', #35799, #17886, #22886, .T. ) ;
#1338=ORIENTED_EDGE ( 'NONE', *, *, #7480, .F. ) ;
#1350=CARTESIAN_POINT ( 'NONE',  ( 114.7192077545248594, -2.791137627527939813, -18.39754474579286025 ) ) ;
#1354=DIRECTION ( 'NONE',  ( -3.317300593186674996E-33, 1.195183497228115774E-16, 1.000000000000000000 ) ) ;
#1357=CARTESIAN_POINT ( 'NONE',  ( 111.0381921295247878, -9.868328341294093420, -13.39321520033836599 ) ) ;
#1361=CYLINDRICAL_SURFACE ( 'NONE', #27421, 5.000000000000004441 ) ;
#1362=CARTESIAN_POINT ( 'NONE',  ( 64.61935771200890599, -37.86087448816891765, -4.893215200338314474 ) ) ;
#1366=EDGE_CURVE ( 'NONE', #32579, #11479, #1090, .T. ) ;
#1377=CARTESIAN_POINT ( 'NONE',  ( 114.9275671295247889, -10.62599879583958540, -13.39321520033831447 ) ) ;
#1378=CARTESIAN_POINT ( 'NONE',  ( 112.0105358795248804, -8.402594152722688392, -9.854619843455216355 ) ) ;
#1379=CARTESIAN_POINT ( 'NONE',  ( 109.7185827545247889, -6.936859964151250502, -8.388885654883777576 ) ) ;
#1384=CARTESIAN_POINT ( 'NONE',  ( 108.8851452545248151, 0.8980012041604421569, -11.00651665394454071 ) ) ;
#1391=CARTESIAN_POINT ( 'NONE',  ( 109.2324108795247923, -8.938348069036489818, -9.318865927141430916 ) ) ;
#1392=CARTESIAN_POINT ( 'NONE',  ( 112.5661608795247872, -1.325403438956436419, -16.93181055722141792 ) ) ;
#1403=CARTESIAN_POINT ( 'NONE',  ( 113.5823964071292806, 0.2518737723193609224, -14.64321520033831447 ) ) ;
#1409=CARTESIAN_POINT ( 'NONE',  ( 106.5931921295248372, -9.868328341294093420, -13.39321520033831447 ) ) ;
#1419=CARTESIAN_POINT ( 'NONE',  ( 71.50489436060276205, -24.57757939319463958, -4.893215200338314474 ) ) ;
#1420=CARTESIAN_POINT ( 'NONE',  ( 112.3578015045248861, -2.477300249445798297, -7.631215200338321125 ) ) ;
#1424=ADVANCED_FACE ( 'NONE', ( #42377 ), #25497, .T. ) ;
#1430=CARTESIAN_POINT ( 'NONE',  ( 111.5243640045248412, -10.62599879583958717, -11.00651665394454604 ) ) ;
#1431=CARTESIAN_POINT ( 'NONE',  ( 116.2471765045247594, -2.791137627527939813, -8.388885654883777576 ) ) ;
#1432=CARTESIAN_POINT ( 'NONE',  ( 115.5526452545247622, 0.8980012041604421569, -11.00651665394454071 ) ) ;
#1438=CARTESIAN_POINT ( 'NONE',  ( 105.9681140045248355, -10.62599879583958717, -11.00651665394454604 ) ) ;
#1442=CARTESIAN_POINT ( 'NONE',  ( 117.1639140680481148, -11.17155048450423571, -5.478470727163857745 ) ) ;
#1443=CARTESIAN_POINT ( 'NONE',  ( 107.0793640045248196, 0.1403307496149616695, -15.46607636864997204 ) ) ;
#1445=CARTESIAN_POINT ( 'NONE',  ( 115.6915515045247531, -2.477300249445798297, -7.631215200338321125 ) ) ;
#1449=CARTESIAN_POINT ( 'NONE',  ( 113.3995983795247895, -8.402594152722688392, -16.93181055722141792 ) ) ;
#1450=CARTESIAN_POINT ( 'NONE',  ( 105.6208483795248299, -0.7896495226426338832, -9.318865927141430916 ) ) ;
#1456=ORIENTED_EDGE ( 'NONE', *, *, #21137, .F. ) ;
#1461=ORIENTED_EDGE ( 'NONE', *, *, #33249, .T. ) ;
#1466=DIRECTION ( 'NONE',  ( 0.000000000000000000, 0.5905882410490338463, 0.8069730661766898461 ) ) ;
#1468=CARTESIAN_POINT ( 'NONE',  ( 114.9275671295247889, 0.1403307496149613920, -13.39321520033831447 ) ) ;
#1476=DIRECTION ( 'NONE',  ( 0.000000000000000000, 1.000000000000000000, 0.000000000000000000 ) ) ;
#1477=B_SPLINE_CURVE_WITH_KNOTS ( 'NONE', 3,
 ( #15560, #4843, #19211, #1859, #4618, #1638, #18762, #32652, #8949, #33090, #22850, #11923, #36741, #18539, #8718, #8274, #32430, #1204, #15118, #32869, #39954, #39730, #29465, #43380, #26051, #8499, #42936, #11697, #22177, #5064, #18979, #36522, #5295, #14589, #10732, #25081, #39436, #14818, #38973 ),
 .UNSPECIFIED., .F., .F.,
 ( 4, 2, 2, 2, 1, 1, 1, 2, 2, 2, 2, 1, 1, 1, 2, 2, 2, 2, 1, 1, 1, 2, 2, 4 ),
 ( 0.000000000000000000, 0.1250000000001450784, 0.1875000000002177425, 0.2187500000002557954, 0.2343750000002725598, 0.2421875000002784162, 0.2460937500002818301, 0.2480468750002813305, 0.2500000000002808309, 0.3750000000002225997, 0.4375000000001940115, 0.4687500000001821321, 0.4843750000001779132, 0.4921875000001740275, 0.4960937500001719735, 0.5000000000001699751, 0.6250000000001478817, 0.6875000000001361133, 0.7187500000001322276, 0.7343750000001287859, 0.7421875000001285638, 0.7460937500001243450, 0.7500000000001200151, 1.000000000000000000 ),
 .UNSPECIFIED. ) ;
#1478=CARTESIAN_POINT ( 'NONE',  ( 116.1808983795247769, -1.328464889906837199, -9.857681294405580275 ) ) ;
#1479=CARTESIAN_POINT ( 'NONE',  ( 109.9269421295247753, -9.868328341294093420, -13.39321520033831447 ) ) ;
#1481=CARTESIAN_POINT ( 'NONE',  ( 92.26512299712632625, -23.76310523276723785, -4.893215200338314474 ) ) ;
#1489=CARTESIAN_POINT ( 'NONE',  ( 108.1211608795247798, -1.325403438956436419, -16.93181055722141792 ) ) ;
#1494=CARTESIAN_POINT ( 'NONE',  ( 110.2742077545248094, -7.250697342233347165, -7.631215200338321125 ) ) ;
#1502=CARTESIAN_POINT ( 'NONE',  ( 106.1764733795248219, -1.325403438956436419, -9.854619843455211026 ) ) ;
#1504=CARTESIAN_POINT ( 'NONE',  ( 83.65649369947882974, -32.32350872240788675, -21.29440707590126536 ) ) ;
#1507=CARTESIAN_POINT ( 'NONE',  ( 108.2600671295247992, -10.62599879583958540, -13.39321520033831447 ) ) ;
#1518=CARTESIAN_POINT ( 'NONE',  ( 110.8298327545248299, -2.477300249445798297, -19.15521520033831138 ) ) ;
#1520=CARTESIAN_POINT ( 'NONE',  ( 111.0001630180080809, 0.7607806665038616689, -14.64321520033831447 ) ) ;
#1525=ORIENTED_EDGE ( 'NONE', *, *, #11406, .T. ) ;
#1531=CARTESIAN_POINT ( 'NONE',  ( 64.01282776924008999, -34.86145050234441811, -5.893215200338315363 ) ) ;
#1539=CIRCLE ( 'NONE', #5799, 2.000000000000000000 ) ;
#1542=CARTESIAN_POINT ( 'NONE',  ( 113.8857702545248003, 0.1403307496149616695, -11.32035403202665336 ) ) ;
#1546=CARTESIAN_POINT ( 'NONE',  ( 106.4542858795248179, -8.402594152722688392, -9.854619843455216355 ) ) ;
#1547=CARTESIAN_POINT ( 'NONE',  ( 111.3160046295247838, -4.863998795839590272, -18.39754474579285315 ) ) ;
#1556=DIRECTION ( 'NONE',  ( 0.000000000000000000, 0.000000000000000000, -1.000000000000000000 ) ) ;
#1557=CARTESIAN_POINT ( 'NONE',  ( 109.3713171295247832, 0.1403307496149613920, -13.39321520033831447 ) ) ;
#1564=CARTESIAN_POINT ( 'NONE',  ( 143.3676850761856940, -60.26310523276723785, -29.64311716074571379 ) ) ;
#1565=DIRECTION ( 'NONE',  ( 0.000000000000000000, 0.000000000000000000, -1.000000000000000000 ) ) ;
#1567=EDGE_CURVE ( 'NONE', #31450, #27343, #1756, .T. ) ;
#1568=CARTESIAN_POINT ( 'NONE',  ( 114.9275671295247889, 0.1403307496149613920, -13.39321520033831447 ) ) ;
#1569=AXIS2_PLACEMENT_3D ( 'NONE', #40150, #39699, #32835 ) ;
#1572=EDGE_LOOP ( 'NONE', ( #5834, #26562, #648, #6802 ) ) ;
#1575=CARTESIAN_POINT ( 'NONE',  ( 111.2465515045248168, -6.936859964151197211, -18.39754474579287447 ) ) ;
#1579=CARTESIAN_POINT ( 'NONE',  ( 109.5102233795247884, -1.325403438956533675, -9.854619843455186157 ) ) ;
#1595=CARTESIAN_POINT ( 'NONE',  ( 114.8811338361194743, 0.1075849324168598464, -12.14321520033831625 ) ) ;
#1596=EDGE_CURVE ( 'NONE', #42526, #38298, #5731, .T. ) ;
#1597=CARTESIAN_POINT ( 'NONE',  ( 116.2471765045247594, -7.250697342233347165, -19.15521520033831138 ) ) ;
#1598=CARTESIAN_POINT ( 'NONE',  ( 111.8716296295247901, -4.863998795839590272, -8.388885654883775800 ) ) ;
#1599=CARTESIAN_POINT ( 'NONE',  ( 109.3713171295247832, 0.1403307496149613920, -13.39321520033831447 ) ) ;
#1602=EDGE_LOOP ( 'NONE', ( #39178, #37336, #34760, #27849 ) ) ;
#1603=CARTESIAN_POINT ( 'NONE',  ( 107.7738952545248310, 0.8980012041604421569, -11.00651665394454071 ) ) ;
#1604=CARTESIAN_POINT ( 'NONE',  ( 61.69189222814998175, -48.76310523276723785, -24.89321520033831447 ) ) ;
#1609=CARTESIAN_POINT ( 'NONE',  ( 109.9963952545248134, 0.8980012041604421569, -11.00651665394454071 ) ) ;
#1615=B_SPLINE_CURVE_WITH_KNOTS ( 'NONE', 3,
 ( #6118, #2233, #19574, #12520, #5882, #30067, #33917, #30287, #20036, #2688, #44433, #23227, #9093, #16849, #34149, #30741, #13427, #40328, #33691, #33453, #22994, #43979, #12744, #26645, #9319, #2463, #16386, #17866, #39285, #31982, #25162, #24929, #3721, #38374, #28808 ),
 .UNSPECIFIED., .F., .F.,
 ( 4, 2, 2, 1, 1, 1, 2, 2, 2, 2, 1, 1, 2, 2, 2, 2, 1, 1, 2, 2, 4 ),
 ( 0.000000000000000000, 0.1250000000003427814, 0.1875000000005233869, 0.2187500000006241119, 0.2343750000006737666, 0.2421875000006920020, 0.2460937500006886713, 0.2500000000006853407, 0.3750000000005874745, 0.4375000000005401235, 0.4687500000005156431, 0.4843750000005034306, 0.4921875000004973244, 0.5000000000004911627, 0.6250000000004246603, 0.6875000000003913536, 0.7187500000003758105, 0.7343750000003669287, 0.7421875000003596012, 0.7500000000003522738, 1.000000000000000000 ),
 .UNSPECIFIED. ) ;
#1621=EDGE_CURVE ( 'NONE', #43791, #29714, #44805, .T. ) ;
#1629=CARTESIAN_POINT ( 'NONE',  ( 106.2459265045248173, -2.791137627527939813, -8.388885654883777576 ) ) ;
#1631=ORIENTED_EDGE ( 'NONE', *, *, #31239, .F. ) ;
#1638=CARTESIAN_POINT ( 'NONE',  ( 61.77599217838784540, -65.91878806257270185, -43.48361792650258906 ) ) ;
#1639=CARTESIAN_POINT ( 'NONE',  ( 107.6349890045248401, 0.8980012041604421569, -15.77991374673208469 ) ) ;
#1643=( BOUNDED_CURVE ( )  B_SPLINE_CURVE ( 3, ( #8948, #12374, #30373, #12603 ),
 .UNSPECIFIED., .F., .F. ) 
 B_SPLINE_CURVE_WITH_KNOTS ( ( 4, 4 ),
 ( 4.329840622631089708, 4.712388980384689674 ),
 .UNSPECIFIED. ) 
 CURVE ( )  GEOMETRIC_REPRESENTATION_ITEM ( )  RATIONAL_B_SPLINE_CURVE ( ( 1.000000000000000000, 0.9878418653401740412, 0.9878418653401740412, 1.000000000000000000 ) ) 
 REPRESENTATION_ITEM ( '' )  );
#1645=DIRECTION ( 'NONE',  ( 0.000000000000000000, -0.7876185884367603585, 0.6161630946014903243 ) ) ;
#1650=EDGE_CURVE ( 'NONE', #26421, #38311, #22043, .T. ) ;
#1652=CARTESIAN_POINT ( 'NONE',  ( 111.1076452545248259, 0.8980012041604421569, -11.00651665394454071 ) ) ;
#1654=CARTESIAN_POINT ( 'NONE',  ( 116.6638952545248031, -9.868328341294098749, -15.46607636864997204 ) ) ;
#1655=CARTESIAN_POINT ( 'NONE',  ( 110.1353015045248469, -2.477300249445798297, -7.631215200338321125 ) ) ;
#1660=CARTESIAN_POINT ( 'NONE',  ( 107.4266296295248821, -4.863998795839590272, -19.15521520033831493 ) ) ;
#1664=CARTESIAN_POINT ( 'NONE',  ( 117.1731602005347384, -11.14203525093994251, -5.453018689005371122 ) ) ;
#1668=CARTESIAN_POINT ( 'NONE',  ( 109.2294421294243136, -10.06703191844256651, -15.14667944815581535 ) ) ;
#1670=CARTESIAN_POINT ( 'NONE',  ( 113.2606921295247702, -9.868328341294093420, -13.39321520033831447 ) ) ;
#1671=CARTESIAN_POINT ( 'NONE',  ( 115.6220983795247861, -8.402594152722688392, -16.93181055722141792 ) ) ;
#1673=CYLINDRICAL_SURFACE ( 'NONE', #5179, 20.00000000000000000 ) ;
#1674=CARTESIAN_POINT ( 'NONE',  ( 70.92411738817702371, -25.94128094577593657, -5.473262044462485321 ) ) ;
#1678=EDGE_CURVE ( 'NONE', #24866, #22218, #24105, .T. ) ;
#1686=VECTOR ( 'NONE', #20269, 999.9999999999998863 ) ;
#1691=CARTESIAN_POINT ( 'NONE',  ( 106.3848327545248651, -2.477300249445798297, -19.15521520033831138 ) ) ;
#1694=CARTESIAN_POINT ( 'NONE',  ( 115.6220983795247861, -8.402594152722688392, -16.93181055722141792 ) ) ;
#1696=PLANE ( 'NONE',  #28500 ) ;
#1697=CARTESIAN_POINT ( 'NONE',  ( 83.82415148905927538, -48.76310523276723785, -24.89321520033831447 ) ) ;
#1702=CARTESIAN_POINT ( 'NONE',  ( 116.1114452545248525, 0.1360012041604422017, -11.32214738847284075 ) ) ;
#1703=CARTESIAN_POINT ( 'NONE',  ( 111.7327233795247849, -1.325403438956436419, -9.854619843455211026 ) ) ;
#1713=CARTESIAN_POINT ( 'NONE',  ( 111.5938171295247940, 0.1403307496149613920, -13.39321520033831447 ) ) ;
#1715=EDGE_CURVE ( 'NONE', #25696, #41400, #24357, .T. ) ;
#1719=CARTESIAN_POINT ( 'NONE',  ( 108.1211608795247798, -8.938348069036489818, -9.318865927141430916 ) ) ;
#1723=CARTESIAN_POINT ( 'NONE',  ( 63.69189222814998175, -50.16718729050181480, 3.106784799661685526 ) ) ;
#1724=CARTESIAN_POINT ( 'NONE',  ( 109.9963952545248134, 0.8980012041604421569, -11.00651665394454071 ) ) ;
#1725=DIRECTION ( 'NONE',  ( 0.000000000000000000, 0.3713878862591642460, -0.9284778069183722282 ) ) ;
#1726=CARTESIAN_POINT ( 'NONE',  ( 83.87098973808613778, -31.73904887874523340, -22.52550971913698419 ) ) ;
#1729=CARTESIAN_POINT ( 'NONE',  ( 108.1211608795247798, -8.938348069036489818, -9.318865927141430916 ) ) ;
#1742=CARTESIAN_POINT ( 'NONE',  ( 107.2182702545248105, -10.62599879583958717, -15.77991374673208469 ) ) ;
#1744=CARTESIAN_POINT ( 'NONE',  ( 83.46705746533213244, -32.83968548964498524, -23.89321520033831803 ) ) ;
#1746=ORIENTED_EDGE ( 'NONE', *, *, #39630, .T. ) ;
#1753=CARTESIAN_POINT ( 'NONE',  ( 83.86216108596053687, -30.76310523276723785, -22.89321520033831803 ) ) ;
#1756=LINE ( 'NONE', #19547, #36017 ) ;
#1765=CARTESIAN_POINT ( 'NONE',  ( 113.7468640045248236, 0.1403307496149616695, -15.46607636864997204 ) ) ;
#1769=CARTESIAN_POINT ( 'NONE',  ( 106.3153796295248412, -4.863998795839590272, -8.388885654883775800 ) ) ;
#1770=CARTESIAN_POINT ( 'NONE',  ( 111.3854577545248645, -2.791137627527939813, -18.39754474579286025 ) ) ;
#1782=CARTESIAN_POINT ( 'NONE',  ( 109.1629577545248395, -2.791137627527939813, -18.39754474579286025 ) ) ;
#1792=CARTESIAN_POINT ( 'NONE',  ( 111.7327233795247849, -1.325403438956436419, -9.854619843455211026 ) ) ;
#1798=FACE_BOUND ( 'NONE', #15754, .T. ) ;
#1801=VERTEX_POINT ( 'NONE', #20460 ) ;
#1807=AXIS2_PLACEMENT_3D ( 'NONE', #35738, #10915, #29133 ) ;
#1809=LINE ( 'NONE', #19599, #44500 ) ;
#1813=CARTESIAN_POINT ( 'NONE',  ( 116.6540404065295178, -9.155876812127887732, -16.09229352560785031 ) ) ;
#1819=CARTESIAN_POINT ( 'NONE',  ( 114.4583197905468808, 0.6938714319018670640, -12.14321520033833579 ) ) ;
#1820=CARTESIAN_POINT ( 'NONE',  ( 109.9963952545248134, 0.8980012041604421569, -11.00651665394454071 ) ) ;
#1821=CARTESIAN_POINT ( 'NONE',  ( 111.0381921295247878, -9.868328341294093420, -13.39321520033831447 ) ) ;
#1822=CARTESIAN_POINT ( 'NONE',  ( 110.7603796295247918, -4.863998795839590272, -8.388885654883775800 ) ) ;
#1825=ORIENTED_EDGE ( 'NONE', *, *, #24490, .T. ) ;
#1831=CARTESIAN_POINT ( 'NONE',  ( 108.7462390045248242, 0.8980012041604421569, -15.77991374673208469 ) ) ;
#1847=ORIENTED_EDGE ( 'NONE', *, *, #42590, .F. ) ;
#1851=CARTESIAN_POINT ( 'NONE',  ( 115.2053796295247849, -4.863998795839590272, -19.15521520033831493 ) ) ;
#1859=CARTESIAN_POINT ( 'NONE',  ( 61.74332929926398350, -66.01496853250924346, -43.25593076250496694 ) ) ;
#1868=EDGE_CURVE ( 'NONE', #4322, #970, #41663, .T. ) ;
#1870=ORIENTED_EDGE ( 'NONE', *, *, #31960, .F. ) ;
#1872=DIRECTION ( 'NONE',  ( 0.000000000000000000, 0.8069730661766899571, -0.5905882410490339574 ) ) ;
#1873=CARTESIAN_POINT ( 'NONE',  ( 110.6909265045248247, -7.250697342233347165, -19.15521520033831138 ) ) ;
#1875=CARTESIAN_POINT ( 'NONE',  ( 110.8298327545248299, -2.477300249445798297, -19.15521520033831138 ) ) ;
#1876=VECTOR ( 'NONE', #43079, 1000.000000000000000 ) ;
#1878=ORIENTED_EDGE ( 'NONE', *, *, #1567, .F. ) ;
#1881=CARTESIAN_POINT ( 'NONE',  ( 106.1070202545248407, -10.62599879583958717, -15.77991374673208469 ) ) ;
#1886=ORIENTED_EDGE ( 'NONE', *, *, #7632, .F. ) ;
#1887=DIRECTION ( 'NONE',  ( -1.000000000000000000, 0.000000000000000000, 0.000000000000000000 ) ) ;
#1888=CARTESIAN_POINT ( 'NONE',  ( 109.2294421359564467, -10.14375206540927365, -14.94852355942958155 ) ) ;
#1891=CARTESIAN_POINT ( 'NONE',  ( 114.3024890045248156, -9.868328341294098749, -11.32035403202665869 ) ) ;
#1892=CARTESIAN_POINT ( 'NONE',  ( 112.4272546295247821, -4.863998795839590272, -18.39754474579285315 ) ) ;
#1894=DIRECTION ( 'NONE',  ( 0.000000000000000000, 0.000000000000000000, -1.000000000000000000 ) ) ;
#1895=CARTESIAN_POINT ( 'NONE',  ( 69.79878637322866552, -26.09957013199193554, -5.786566508650874852 ) ) ;
#1904=ORIENTED_EDGE ( 'NONE', *, *, #32554, .T. ) ;
#1906=ADVANCED_FACE ( 'NONE', ( #2890, #17472 ), #31369, .T. ) ;
#1907=AXIS2_PLACEMENT_3D ( 'NONE', #5450, #8440, #15500 ) ;
#1913=CARTESIAN_POINT ( 'NONE',  ( 106.4542858795248179, -0.7896495226426338832, -17.46756447353520159 ) ) ;
#1916=CARTESIAN_POINT ( 'NONE',  ( 108.8851452545248151, -9.868328341294098749, -15.46607636864997204 ) ) ;
#1924=EDGE_CURVE ( 'NONE', #12824, #19575, #42844, .T. ) ;
#1927=CARTESIAN_POINT ( 'NONE',  ( 116.6670702545247593, -9.863998795839588496, -15.46428301220378998 ) ) ;
#1928=CARTESIAN_POINT ( 'NONE',  ( 108.3989733795247759, -1.325403438956436419, -9.854619843455211026 ) ) ;
#1931=AXIS2_PLACEMENT_3D ( 'NONE', #40032, #8352, #15192 ) ;
#1934=CARTESIAN_POINT ( 'NONE',  ( 69.87572422742091760, -11.86958442233774313, -21.39321520033831447 ) ) ;
#1938=CARTESIAN_POINT ( 'NONE',  ( 61.69084222814998242, -0.02276961308034231024, -12.14321520033831625 ) ) ;
#1940=CARTESIAN_POINT ( 'NONE',  ( 111.8021765045248372, -2.791137627527939813, -8.388885654883777576 ) ) ;
#1945=CARTESIAN_POINT ( 'NONE',  ( 106.5931921295248372, 0.8980012041604618078, -13.39321520033831447 ) ) ;
#1948=LINE ( 'NONE', #39813, #37916 ) ;
#1949=CARTESIAN_POINT ( 'NONE',  ( 111.8716296295247901, -4.863998795839590272, -19.15521520033831493 ) ) ;
#1951=CARTESIAN_POINT ( 'NONE',  ( 116.3860827545247787, -2.477300249445798297, -19.15521520033831138 ) ) ;
#1957=ORIENTED_EDGE ( 'NONE', *, *, #33681, .T. ) ;
#1958=CARTESIAN_POINT ( 'NONE',  ( 72.75524511225664526, -25.99489077589583630, -8.393215200338314474 ) ) ;
#1967=VECTOR ( 'NONE', #8831, 1000.000000000000000 ) ;
#1968=CARTESIAN_POINT ( 'NONE',  ( 107.3571765045248299, -7.250697342233347165, -19.15521520033831138 ) ) ;
#1970=CARTESIAN_POINT ( 'NONE',  ( 110.9481121053769073, 0.3967854368539851517, -16.28112951403850062 ) ) ;
#1979=CARTESIAN_POINT ( 'NONE',  ( 109.2294421295247844, 0.8460904216231607267, -12.14321520033831625 ) ) ;
#1995=CARTESIAN_POINT ( 'NONE',  ( 115.6915515045247531, -6.936859964151250502, -18.39754474579286025 ) ) ;
#1999=CARTESIAN_POINT ( 'NONE',  ( 113.0523327545247838, -2.477300249445798297, -19.15521520033831138 ) ) ;
#2000=CARTESIAN_POINT ( 'NONE',  ( 111.0381921295247878, -9.868328341294093420, -13.39321520033831447 ) ) ;
#2004=CARTESIAN_POINT ( 'NONE',  ( 112.9134265045247645, -2.791137627527939813, -8.388885654883777576 ) ) ;
#2005=EDGE_LOOP ( 'NONE', ( #20661, #33610, #40801, #10397 ) ) ;
#2012=CARTESIAN_POINT ( 'NONE',  ( 106.9404577545248145, -2.791137627527939813, -18.39754474579286025 ) ) ;
#2018=FACE_OUTER_BOUND ( 'NONE', #39725, .T. ) ;
#2019=LINE ( 'NONE', #5439, #1876 ) ;
#2021=CARTESIAN_POINT ( 'NONE',  ( 111.9410827545248708, -6.936859964151250502, -8.388885654883777576 ) ) ;
#2027=LINE ( 'NONE', #29855, #19846 ) ;
#2029=ORIENTED_EDGE ( 'NONE', *, *, #27260, .F. ) ;
#2050=CARTESIAN_POINT ( 'NONE',  ( 113.7468640045248236, -10.62599879583958717, -11.00651665394454604 ) ) ;
#2051=CARTESIAN_POINT ( 'NONE',  ( 108.8156921295247912, -9.868328341294093420, -13.39321520033831447 ) ) ;
#2052=CARTESIAN_POINT ( 'NONE',  ( 107.1488171295248861, 0.1403307496149613920, -13.39321520033831447 ) ) ;
#2053=VECTOR ( 'NONE', #39873, 1000.000000000000000 ) ;
#2058=DIRECTION ( 'NONE',  ( 1.000000000000000000, 0.000000000000000000, 0.000000000000000000 ) ) ;
#2062=CARTESIAN_POINT ( 'NONE',  ( 108.2600671295247992, -10.62599879583958540, -13.39321520033831447 ) ) ;
#2063=DIRECTION ( 'NONE',  ( -1.000000000000000000, 0.000000000000000000, 0.000000000000000000 ) ) ;
#2064=ORIENTED_EDGE ( 'NONE', *, *, #36464, .F. ) ;
#2078=ORIENTED_EDGE ( 'NONE', *, *, #35027, .T. ) ;
#2081=CARTESIAN_POINT ( 'NONE',  ( 112.4967077545247633, -7.250697342233347165, -7.631215200338321125 ) ) ;
#2088=ORIENTED_EDGE ( 'NONE', *, *, #12602, .T. ) ;
#2090=DIRECTION ( 'NONE',  ( 0.000000000000000000, 0.000000000000000000, 1.000000000000000000 ) ) ;
#2099=CARTESIAN_POINT ( 'NONE',  ( 114.6497546295247929, -4.863998795839590272, -7.631215200338315796 ) ) ;
#2100=CARTESIAN_POINT ( 'NONE',  ( 114.5803015045248117, -6.936859964151250502, -18.39754474579286025 ) ) ;
#2101=CARTESIAN_POINT ( 'NONE',  ( 111.9410827545248708, -2.477300249445798297, -19.15521520033831138 ) ) ;
#2106=CARTESIAN_POINT ( 'NONE',  ( 106.9404577545248145, -7.250697342233347165, -7.631215200338321125 ) ) ;
#2110=CARTESIAN_POINT ( 'NONE',  ( 116.9195933520218489, -11.60549135878080129, -5.961931887625801174 ) ) ;
#2111=EDGE_LOOP ( 'NONE', ( #24890, #26882, #38289, #33119 ) ) ;
#2113=CARTESIAN_POINT ( 'NONE',  ( 109.2294398899149570, -10.40495872603004912, -13.78690482381271920 ) ) ;
#2115=CARTESIAN_POINT ( 'NONE',  ( 112.7050671295247923, 0.1403307496149613920, -13.39321520033831447 ) ) ;
#2116=CARTESIAN_POINT ( 'NONE',  ( 111.5243640045248412, 0.1403307496149616695, -15.46607636864997204 ) ) ;
#2120=CARTESIAN_POINT ( 'NONE',  ( 69.72146619215227759, -25.52849560314718858, -5.786566508650934360 ) ) ;
#2134=CARTESIAN_POINT ( 'NONE',  ( 108.3989733795248753, -8.938348069036489818, -17.46756447353520159 ) ) ;
#2137=CARTESIAN_POINT ( 'NONE',  ( 107.9822546295247889, -4.863998795839590272, -18.39754474579285315 ) ) ;
#2155=CARTESIAN_POINT ( 'NONE',  ( 110.1534981608379837, 0.3867979994853637526, -14.64321520033831447 ) ) ;
#2157=CARTESIAN_POINT ( 'NONE',  ( 111.7327233795247849, -1.325403438956436419, -9.854619843455211026 ) ) ;
#2163=CARTESIAN_POINT ( 'NONE',  ( 115.0664733795247798, -1.325403438956436419, -9.854619843455211026 ) ) ;
#2167=CARTESIAN_POINT ( 'NONE',  ( 111.4549108795247747, -8.938348069036489818, -9.318865927141430916 ) ) ;
#2169=CARTESIAN_POINT ( 'NONE',  ( 112.7745202545247878, -10.62599879583958717, -15.77991374673208469 ) ) ;
#2172=CARTESIAN_POINT ( 'NONE',  ( 106.1764733795248219, -8.938348069036489818, -17.46756447353520159 ) ) ;
#2176=CARTESIAN_POINT ( 'NONE',  ( 70.36267391504962632, -5.685877709920933221, -4.893215200338314474 ) ) ;
#2177=EDGE_CURVE ( 'NONE', #18453, #20631, #29303, .T. ) ;
#2189=CARTESIAN_POINT ( 'NONE',  ( 110.1353015045248469, -2.477300249445798297, -7.631215200338321125 ) ) ;
#2192=CARTESIAN_POINT ( 'NONE',  ( 116.7994817539454147, -2.735128593956382748, -18.16285249951504355 ) ) ;
#2201=CARTESIAN_POINT ( 'NONE',  ( 114.0923066399283812, 0.4261359969231631739, -14.64321520033831447 ) ) ;
#2202=CARTESIAN_POINT ( 'NONE',  ( 108.2600671295247992, 0.1403307496149613920, -13.39321520033831447 ) ) ;
#2203=CARTESIAN_POINT ( 'NONE',  ( 109.4177504229301690, 0.1075849324168598464, -14.64321520033834645 ) ) ;
#2204=CARTESIAN_POINT ( 'NONE',  ( 70.19189222814998175, -41.58126682492877535, -29.83537093841426469 ) ) ;
#2213=CARTESIAN_POINT ( 'NONE',  ( 113.5385046295247804, -4.863998795839590272, -18.39754474579285315 ) ) ;
#2217=CARTESIAN_POINT ( 'NONE',  ( 116.1777233795247781, -8.938348069036489818, -17.46756447353520159 ) ) ;
#2218=CARTESIAN_POINT ( 'NONE',  ( 107.7044421295247929, -9.868328341294093420, -13.39321520033831447 ) ) ;
#2219=CARTESIAN_POINT ( 'NONE',  ( 83.19148113855052884, -31.91406586441351934, -23.42170072420262628 ) ) ;
#2223=CARTESIAN_POINT ( 'NONE',  ( 61.69189222814998175, -61.90644496644519990, -36.30514255143466329 ) ) ;
#2224=CARTESIAN_POINT ( 'NONE',  ( 113.1217858795247935, -8.402594152722688392, -9.854619843455216355 ) ) ;
#2225=VERTEX_POINT ( 'NONE', #26563 ) ;
#2227=CARTESIAN_POINT ( 'NONE',  ( 109.2296046993104710, -0.1282053629079296375, -15.30017343217149950 ) ) ;
#2233=CARTESIAN_POINT ( 'NONE',  ( 116.3474387856597758, -11.99696240085007837, -20.96724589306712261 ) ) ;
#2234=EDGE_LOOP ( 'NONE', ( #6707, #17676, #1870, #18909 ) ) ;
#2238=SURFACE_STYLE_USAGE ( .BOTH. , #19579 ) ;
#2242=ADVANCED_FACE ( 'NONE', ( #11984 ), #22304, .T. ) ;
#2243=CARTESIAN_POINT ( 'NONE',  ( 113.1912390045248031, -9.868328341294098749, -11.32035403202665869 ) ) ;
#2244=TOROIDAL_SURFACE ( 'NONE', #34311, 10.00000000000000000, 2.000000000000000000 ) ;
#2247=ORIENTED_EDGE ( 'NONE', *, *, #38111, .T. ) ;
#2253=ORIENTED_EDGE ( 'NONE', *, *, #38111, .F. ) ;
#2258=AXIS2_PLACEMENT_3D ( 'NONE', #28724, #666, #4760 ) ;
#2273=CARTESIAN_POINT ( 'NONE',  ( 110.6214733795247867, -8.938348069036489818, -17.46756447353520159 ) ) ;
#2274=CARTESIAN_POINT ( 'NONE',  ( 108.4684265045248424, -2.791137627527939813, -8.388885654883777576 ) ) ;
#2275=CARTESIAN_POINT ( 'NONE',  ( 110.5520202545248054, 0.1403307496149616695, -11.32035403202665336 ) ) ;
#2276=CIRCLE ( 'NONE', #16889, 0.5000000000000004441 ) ;
#2277=CARTESIAN_POINT ( 'NONE',  ( 64.01282776924008999, -34.86145050234443943, -5.893215200338315363 ) ) ;
#2281=CARTESIAN_POINT ( 'NONE',  ( 109.2294611991032554, -8.247533281633225855, -8.767455091437543757 ) ) ;
#2284=CARTESIAN_POINT ( 'NONE',  ( 105.6903015045248253, -6.936859964151250502, -18.39754474579286025 ) ) ;
#2287=CARTESIAN_POINT ( 'NONE',  ( 107.2182702545248105, -10.62599879583958717, -15.77991374673208469 ) ) ;
#2288=CARTESIAN_POINT ( 'NONE',  ( 116.5944421295247793, -4.863998795839590272, -13.39321520033831447 ) ) ;
#2290=CARTESIAN_POINT ( 'NONE',  ( 111.0001630180080809, 0.7607806665038616689, -14.64321520033831447 ) ) ;
#2307=CARTESIAN_POINT ( 'NONE',  ( 112.2188952545247531, 0.8980012041604421569, -11.00651665394454071 ) ) ;
#2329=CARTESIAN_POINT ( 'NONE',  ( 113.6774108795247997, -8.938348069036489818, -9.318865927141430916 ) ) ;
#2330=CARTESIAN_POINT ( 'NONE',  ( 113.9552233795247815, -1.325403438956436419, -9.854619843455211026 ) ) ;
#2331=CARTESIAN_POINT ( 'NONE',  ( 111.7327233795247849, -8.938348069036489818, -17.46756447353520159 ) ) ;
#2339=CYLINDRICAL_SURFACE ( 'NONE', #11824, 5.000000000000000000 ) ;
#2347=CARTESIAN_POINT ( 'NONE',  ( 106.9404577545248145, -2.791137627527939813, -18.39754474579286025 ) ) ;
#2348=CARTESIAN_POINT ( 'NONE',  ( 110.7603796295247918, -4.863998795839590272, -8.388885654883775800 ) ) ;
#2350=CARTESIAN_POINT ( 'NONE',  ( 69.97727075072853609, -25.42500284328563964, -5.723131632646515143 ) ) ;
#2358=EDGE_CURVE ( 'NONE', #37481, #40668, #44581, .T. ) ;
#2367=DIRECTION ( 'NONE',  ( 0.000000000000000000, 0.000000000000000000, 1.000000000000000000 ) ) ;
#2368=ORIENTED_EDGE ( 'NONE', *, *, #32345, .F. ) ;
#2370=CARTESIAN_POINT ( 'NONE',  ( 109.4407702545248355, 0.1403307496149616695, -11.32035403202665336 ) ) ;
#2371=AXIS2_PLACEMENT_3D ( 'NONE', #41951, #5989, #2570 ) ;
#2372=DIRECTION ( 'NONE',  ( -1.000000000000000000, 0.000000000000000000, 0.000000000000000000 ) ) ;
#2377=CARTESIAN_POINT ( 'NONE',  ( 116.8754296295248025, -4.863998795839590272, -18.39321520033831803 ) ) ;
#2378=MECHANICAL_DESIGN_GEOMETRIC_PRESENTATION_REPRESENTATION('',(#19877),#43182);
#2382=CARTESIAN_POINT ( 'NONE',  ( 61.69189222814998175, -60.36723518915388809, -40.15320052877397217 ) ) ;
#2384=CARTESIAN_POINT ( 'NONE',  ( 69.87842214007035579, -26.26439233367433346, -5.755590708596306726 ) ) ;
#2390=CARTESIAN_POINT ( 'NONE',  ( 111.3160046295247838, -4.863998795839590272, -18.39754474579285315 ) ) ;
#2394=CARTESIAN_POINT ( 'NONE',  ( 114.1635827545248389, -6.936859964151250502, -8.388885654883777576 ) ) ;
#2398=CARTESIAN_POINT ( 'NONE',  ( 109.3713171295247832, -10.62599879583958540, -13.39321520033831447 ) ) ;
#2400=CARTESIAN_POINT ( 'NONE',  ( 112.7050671295247923, -10.62599879583958540, -13.39321520033831447 ) ) ;
#2403=CARTESIAN_POINT ( 'NONE',  ( 115.3442858795247759, -0.7896495226426338832, -17.46756447353520159 ) ) ;
#2408=CIRCLE ( 'NONE', #38821, 20.00000000000000355 ) ;
#2414=ORIENTED_EDGE ( 'NONE', *, *, #17247, .F. ) ;
#2417=ADVANCED_FACE ( 'NONE', ( #37252 ), #6264, .F. ) ;
#2418=CARTESIAN_POINT ( 'NONE',  ( 107.7044421295247929, 0.8980012041604618078, -13.39321520033831447 ) ) ;
#2419=AXIS2_PLACEMENT_3D ( 'NONE', #34160, #31634, #16861 ) ;
#2430=LINE ( 'NONE', #16817, #23110 ) ;
#2431=CARTESIAN_POINT ( 'NONE',  ( 107.2877233795247776, -1.325403438956436419, -9.854619843455211026 ) ) ;
#2433=AXIS2_PLACEMENT_3D ( 'NONE', #12240, #12014, #36382 ) ;
#2444=CARTESIAN_POINT ( 'NONE',  ( 115.1359265045248605, -2.791137627527939813, -8.388885654883777576 ) ) ;
#2450=CARTESIAN_POINT ( 'NONE',  ( 114.2330358795247776, -0.7896495226426338832, -17.46756447353520159 ) ) ;
#2451=CARTESIAN_POINT ( 'NONE',  ( 110.2047546295247855, -4.863998795839590272, -18.39754474579285315 ) ) ;
#2454=CARTESIAN_POINT ( 'NONE',  ( 66.82415148905926117, -40.21211973637273474, -4.893215200338314474 ) ) ;
#2455=CARTESIAN_POINT ( 'NONE',  ( 114.5803015045248117, -6.936859964151250502, -18.39754474579286025 ) ) ;
#2457=CARTESIAN_POINT ( 'NONE',  ( 109.2294786918755278, -0.01490074043973391681, -15.03572518876057806 ) ) ;
#2461=ORIENTED_EDGE ( 'NONE', *, *, #33475, .F. ) ;
#2462=DIRECTION ( 'NONE',  ( 1.000000000000000000, 0.000000000000000000, 0.000000000000000000 ) ) ;
#2463=CARTESIAN_POINT ( 'NONE',  ( 117.0819916265821661, -11.36549209999471266, -21.70826808144084907 ) ) ;
#2471=VECTOR ( 'NONE', #41331, 1000.000000000000000 ) ;
#2473=CARTESIAN_POINT ( 'NONE',  ( 112.3578015045248861, -6.936859964151250502, -18.39754474579286025 ) ) ;
#2484=CARTESIAN_POINT ( 'NONE',  ( 115.9294421295247872, 1.035107641088057973, -4.893215200338314474 ) ) ;
#2501=EDGE_LOOP ( 'NONE', ( #40934, #44267, #8046, #3100, #36010, #17499 ) ) ;
#2503=CARTESIAN_POINT ( 'NONE',  ( 112.2883483795247770, -0.7896495226426338832, -9.318865927141430916 ) ) ;
#2505=CARTESIAN_POINT ( 'NONE',  ( 106.3848327545248651, -6.936859964151250502, -8.388885654883777576 ) ) ;
#2508=EDGE_LOOP ( 'NONE', ( #30104, #14540, #30555, #36508, #31890 ) ) ;
#2510=LINE ( 'NONE', #19852, #8131 ) ;
#2511=EDGE_CURVE ( 'NONE', #32422, #8854, #20847, .T. ) ;
#2515=CARTESIAN_POINT ( 'NONE',  ( 107.5655358795247736, -0.7896495226426338832, -17.46756447353520159 ) ) ;
#2527=VECTOR ( 'NONE', #45030, 1000.000000000000000 ) ;
#2531=VERTEX_POINT ( 'NONE', #37723 ) ;
#2534=VECTOR ( 'NONE', #27301, 1000.000000000000000 ) ;
#2535=CARTESIAN_POINT ( 'NONE',  ( 113.2606921295247702, 0.8980012041604618078, -13.39321520033831447 ) ) ;
#2543=FACE_BOUND ( 'NONE', #6617, .T. ) ;
#2545=CARTESIAN_POINT ( 'NONE',  ( 107.7044421295247929, 0.8980012041604618078, -13.39321520033831447 ) ) ;
#2551=EDGE_LOOP ( 'NONE', ( #41096, #23934, #17870, #2088, #22809, #24035, #12080, #11391, #41619, #30442, #23287, #13989, #19282, #24260, #14132, #38624, #4393, #15346, #42865 ) ) ;
#2556=CARTESIAN_POINT ( 'NONE',  ( 110.4825671295247815, -10.62599879583958540, -13.39321520033831447 ) ) ;
#2557=CARTESIAN_POINT ( 'NONE',  ( 115.4831921295247952, -9.868328341294093420, -13.39321520033831447 ) ) ;
#2558=CARTESIAN_POINT ( 'NONE',  ( 111.3854577545248645, -7.250697342233347165, -7.631215200338321125 ) ) ;
#2570=DIRECTION ( 'NONE',  ( -1.000000000000000000, 0.000000000000000000, 0.000000000000000000 ) ) ;
#2576=CARTESIAN_POINT ( 'NONE',  ( 107.7044421295247929, -9.868328341294093420, -13.39321520033831447 ) ) ;
#2577=CARTESIAN_POINT ( 'NONE',  ( 110.2047546295247855, -4.863998795839590272, -18.39754474579285315 ) ) ;
#2579=CARTESIAN_POINT ( 'NONE',  ( 70.05034961234838420, -25.59043224118723714, -5.724109476187135392 ) ) ;
#2589=( BOUNDED_SURFACE ( )  B_SPLINE_SURFACE ( 1, 2, ( 
 ( #32387, #25114, #36255, #4572, #18040, #1597, #1155, #31935, #15291, #701, #18719, #11880, #15072, #39236, #8000, #39010, #28761, #14621, #28984, #28538, #18268, #21689, #11210, #32163, #1377, #36029, #42444, #29200, #43110, #39691, #25559, #5022, #18938, #32826, #29424, #24883, #15747, #26011, #33495, #2730, #16656, #2050, #44254, #37147, #40367, #29649, #33276, #15974, #5922, #33046, #19844, #43793, #9355, #5248, #30106, #29877, #33732, #44022, #9584, #19166, #40141, #9131, #2503, #23034, #16430, #36922, #37386, #30326, #13010, #12558, #43338, #26909, #19387, #40829, #40597, #23500, #6158, #5692, #20077, #33962, #19611, #26464, #12107, #39915, #43563, #36699, #2273, #16203, #12783, #8905, #8677, #26686, #22580, #12332, #23265, #1820, #36481, #26232, #22803, #5467, #37618, #38061, #6839, #23728, #41942, #24169, #28035, #24387, #41507, #10705, #38273, #10049, #7054, #20965, #16886, #34837, #3185, #20745, #44703, #24608, #34624, #41061, #21183, #10262, #27138, #3622, #9818, #17542, #31435, #3410, #44926, #13685, #13464, #17110, #6392, #17327, #2959, #23953, #27366, #30778, #41287, #202, #27806, #37834, #14118, #38491, #7266, #6612, #35060, #27594, #20299, #20524, #31000, #34404, #13236, #31217, #3841, #30550, #45143, #44471, #34185 ),
 ( #13900, #41721, #10485, #25058, #17761, #4061, #25734, #31885, #11152, #1103, #35975, #4524, #14342, #15020, #14565, #1326, #38719, #15238, #39414, #35288, #28484, #35519, #11378, #18447, #31658, #28256, #11827, #42388, #28708, #8177, #14794, #22087, #25284, #39641, #42165, #426, #42615, #24828, #8405, #28931, #42838, #25509, #11599, #7944, #22309, #4746, #18666, #4291, #36205, #32559, #38951, #29147, #43060, #10926, #7490, #39180, #21407, #17985, #21855, #7718, #650, #21631, #18210, #32108, #35751, #32336, #875, #1770, #1547, #12509, #23214, #5194, #2000, #8629, #5867, #32773, #22749, #26405, #12056, #40315, #9079, #43285, #16371, #43739, #2451, #43965, #15926, #30274, #12729, #29598, #26632, #40545, #36425, #9306, #36650, #22982, #19112, #44199, #36871, #15468, #40770, #29823, #29374, #37093, #25957, #19790, #33673, #5641, #19340, #33225, #32996, #5423, #39864, #19562, #22529, #43515, #15696, #12284, #26180, #12961, #2218, #40088, #26857, #9528, #23444, #8849, #4972, #33439, #16148, #30052, #18882, #9762, #20020, #27541, #41892, #10653, #41232, #38225, #31169, #34355, #23673, #27315, #9992, #45090, #27087, #13846, #37784, #3359, #44418, #24119, #23901, #27761, #38013, #3574, #13184, #2673, #41676, #17058, #10434, #16833, #16605 ) ),
 .UNSPECIFIED., .F., .F., .T. ) 
 B_SPLINE_SURFACE_WITH_KNOTS ( ( 2, 2 ),
 ( 3, 2, 2, 2, 2, 2, 2, 2, 2, 2, 2, 2, 2, 2, 2, 2, 2, 2, 2, 2, 2, 2, 2, 2, 2, 2, 2, 2, 2, 2, 2, 2, 2, 2, 2, 2, 2, 2, 2, 2, 2, 2, 2, 2, 2, 2, 2, 2, 2, 2, 2, 2, 2, 2, 2, 2, 2, 2, 2, 2, 2, 2, 2, 2, 2, 2, 2, 2, 2, 2, 2, 2, 2, 2, 2, 2, 2, 2, 2, 2, 3 ),
 ( 0.000000000000000000, 1.000000000000000000 ),
 ( 0.000000000000000000, 0.01250000000000000069, 0.02500000000000000139, 0.03749999999999999861, 0.05000000000000000278, 0.06250000000000000000, 0.07499999999999999722, 0.08749999999999999445, 0.1000000000000000056, 0.1125000000000000028, 0.1250000000000000000, 0.1375000000000000111, 0.1499999999999999944, 0.1625000000000000056, 0.1749999999999999889, 0.1875000000000000000, 0.2000000000000000111, 0.2124999999999999944, 0.2250000000000000056, 0.2374999999999999889, 0.2500000000000000000, 0.2625000000000000111, 0.2750000000000000222, 0.2874999999999999778, 0.2999999999999999889, 0.3125000000000000000, 0.3250000000000000111, 0.3375000000000000222, 0.3499999999999999778, 0.3624999999999999889, 0.3750000000000000000, 0.3875000000000000111, 0.4000000000000000222, 0.4124999999999999778, 0.4249999999999999889, 0.4375000000000000000, 0.4500000000000000111, 0.4625000000000000222, 0.4749999999999999778, 0.4874999999999999889, 0.5000000000000000000, 0.5124999999999999556, 0.5250000000000000222, 0.5374999999999999778, 0.5500000000000000444, 0.5625000000000000000, 0.5749999999999999556, 0.5875000000000000222, 0.5999999999999999778, 0.6125000000000000444, 0.6250000000000000000, 0.6374999999999999556, 0.6500000000000000222, 0.6624999999999999778, 0.6750000000000000444, 0.6875000000000000000, 0.6999999999999999556, 0.7125000000000000222, 0.7249999999999999778, 0.7375000000000000444, 0.7500000000000000000, 0.7624999999999999556, 0.7750000000000000222, 0.7874999999999999778, 0.8000000000000000444, 0.8125000000000000000, 0.8249999999999999556, 0.8375000000000000222, 0.8499999999999999778, 0.8625000000000000444, 0.8750000000000000000, 0.8874999999999999556, 0.9000000000000000222, 0.9124999999999999778, 0.9250000000000000444, 0.9375000000000000000, 0.9499999999999999556, 0.9625000000000000222, 0.9749999999999999778, 0.9875000000000000444, 1.000000000000000000 ),
 .UNSPECIFIED. ) 
 GEOMETRIC_REPRESENTATION_ITEM ( )  RATIONAL_B_SPLINE_SURFACE ( (
 ( 1.000000000000000000, 0.9238795325112869605, 1.000000000000000000, 0.9238795325112869605, 1.000000000000000000, 0.9238795325112869605, 1.000000000000000000, 0.9238795325112869605, 1.000000000000000000, 0.9238795325112869605, 1.000000000000000000, 0.9238795325112869605, 1.000000000000000000, 0.9238795325112869605, 1.000000000000000000, 0.9238795325112869605, 1.000000000000000000, 0.9238795325112869605, 1.000000000000000000, 0.9238795325112869605, 1.000000000000000000, 0.9238795325112869605, 1.000000000000000000, 0.9238795325112869605, 1.000000000000000000, 0.9238795325112869605, 1.000000000000000000, 0.9238795325112869605, 1.000000000000000000, 0.9238795325112869605, 1.000000000000000000, 0.9238795325112869605, 1.000000000000000000, 0.9238795325112869605, 1.000000000000000000, 0.9238795325112869605, 1.000000000000000000, 0.9238795325112869605, 1.000000000000000000, 0.9238795325112869605, 1.000000000000000000, 0.9238795325112869605, 1.000000000000000000, 0.9238795325112869605, 1.000000000000000000, 0.9238795325112869605, 1.000000000000000000, 0.9238795325112869605, 1.000000000000000000, 0.9238795325112869605, 1.000000000000000000, 0.9238795325112869605, 1.000000000000000000, 0.9238795325112869605, 1.000000000000000000, 0.9238795325112869605, 1.000000000000000000, 0.9238795325112869605, 1.000000000000000000, 0.9238795325112869605, 1.000000000000000000, 0.9238795325112869605, 1.000000000000000000, 0.9238795325112869605, 1.000000000000000000, 0.9238795325112869605, 1.000000000000000000, 0.9238795325112869605, 1.000000000000000000, 0.9238795325112869605, 1.000000000000000000, 0.9238795325112869605, 1.000000000000000000, 0.9238795325112869605, 1.000000000000000000, 0.9238795325112869605, 1.000000000000000000, 0.9238795325112869605, 1.000000000000000000, 0.9238795325112869605, 1.000000000000000000, 0.9238795325112869605, 1.000000000000000000, 0.9238795325112869605, 1.000000000000000000, 0.9238795325112869605, 1.000000000000000000, 0.9238795325112869605, 1.000000000000000000, 0.9238795325112869605, 1.000000000000000000, 0.9238795325112869605, 1.000000000000000000, 0.9238795325112869605, 1.000000000000000000, 0.9238795325112869605, 1.000000000000000000, 0.9238795325112869605, 1.000000000000000000, 0.9238795325112869605, 1.000000000000000000, 0.9238795325112869605, 1.000000000000000000, 0.9238795325112869605, 1.000000000000000000, 0.9238795325112869605, 1.000000000000000000, 0.9238795325112869605, 1.000000000000000000, 0.9238795325112869605, 1.000000000000000000, 0.9238795325112869605, 1.000000000000000000, 0.9238795325112869605, 1.000000000000000000, 0.9238795325112869605, 1.000000000000000000, 0.9238795325112869605, 1.000000000000000000, 0.9238795325112869605, 1.000000000000000000, 0.9238795325112869605, 1.000000000000000000, 0.9238795325112869605, 1.000000000000000000, 0.9238795325112869605, 1.000000000000000000, 0.9238795325112869605, 1.000000000000000000, 0.9238795325112869605, 1.000000000000000000, 0.9238795325112869605, 1.000000000000000000, 0.9238795325112869605, 1.000000000000000000, 0.9238795325112869605, 1.000000000000000000, 0.9238795325112869605, 1.000000000000000000, 0.9238795325112869605, 1.000000000000000000, 0.9238795325112869605, 1.000000000000000000, 0.9238795325112869605, 1.000000000000000000, 0.9238795325112869605, 1.000000000000000000, 0.9238795325112869605, 1.000000000000000000, 0.9238795325112869605, 1.000000000000000000, 0.9238795325112869605, 1.000000000000000000, 0.9238795325112869605, 1.000000000000000000, 0.9238795325112869605, 1.000000000000000000, 0.9238795325112869605, 1.000000000000000000, 0.9238795325112869605, 1.000000000000000000),
 ( 1.000000000000000000, 0.9238795325112869605, 1.000000000000000000, 0.9238795325112869605, 1.000000000000000000, 0.9238795325112869605, 1.000000000000000000, 0.9238795325112869605, 1.000000000000000000, 0.9238795325112869605, 1.000000000000000000, 0.9238795325112869605, 1.000000000000000000, 0.9238795325112869605, 1.000000000000000000, 0.9238795325112869605, 1.000000000000000000, 0.9238795325112869605, 1.000000000000000000, 0.9238795325112869605, 1.000000000000000000, 0.9238795325112869605, 1.000000000000000000, 0.9238795325112869605, 1.000000000000000000, 0.9238795325112869605, 1.000000000000000000, 0.9238795325112869605, 1.000000000000000000, 0.9238795325112869605, 1.000000000000000000, 0.9238795325112869605, 1.000000000000000000, 0.9238795325112869605, 1.000000000000000000, 0.9238795325112869605, 1.000000000000000000, 0.9238795325112869605, 1.000000000000000000, 0.9238795325112869605, 1.000000000000000000, 0.9238795325112869605, 1.000000000000000000, 0.9238795325112869605, 1.000000000000000000, 0.9238795325112869605, 1.000000000000000000, 0.9238795325112869605, 1.000000000000000000, 0.9238795325112869605, 1.000000000000000000, 0.9238795325112869605, 1.000000000000000000, 0.9238795325112869605, 1.000000000000000000, 0.9238795325112869605, 1.000000000000000000, 0.9238795325112869605, 1.000000000000000000, 0.9238795325112869605, 1.000000000000000000, 0.9238795325112869605, 1.000000000000000000, 0.9238795325112869605, 1.000000000000000000, 0.9238795325112869605, 1.000000000000000000, 0.9238795325112869605, 1.000000000000000000, 0.9238795325112869605, 1.000000000000000000, 0.9238795325112869605, 1.000000000000000000, 0.9238795325112869605, 1.000000000000000000, 0.9238795325112869605, 1.000000000000000000, 0.9238795325112869605, 1.000000000000000000, 0.9238795325112869605, 1.000000000000000000, 0.9238795325112869605, 1.000000000000000000, 0.9238795325112869605, 1.000000000000000000, 0.9238795325112869605, 1.000000000000000000, 0.9238795325112869605, 1.000000000000000000, 0.9238795325112869605, 1.000000000000000000, 0.9238795325112869605, 1.000000000000000000, 0.9238795325112869605, 1.000000000000000000, 0.9238795325112869605, 1.000000000000000000, 0.9238795325112869605, 1.000000000000000000, 0.9238795325112869605, 1.000000000000000000, 0.9238795325112869605, 1.000000000000000000, 0.9238795325112869605, 1.000000000000000000, 0.9238795325112869605, 1.000000000000000000, 0.9238795325112869605, 1.000000000000000000, 0.9238795325112869605, 1.000000000000000000, 0.9238795325112869605, 1.000000000000000000, 0.9238795325112869605, 1.000000000000000000, 0.9238795325112869605, 1.000000000000000000, 0.9238795325112869605, 1.000000000000000000, 0.9238795325112869605, 1.000000000000000000, 0.9238795325112869605, 1.000000000000000000, 0.9238795325112869605, 1.000000000000000000, 0.9238795325112869605, 1.000000000000000000, 0.9238795325112869605, 1.000000000000000000, 0.9238795325112869605, 1.000000000000000000, 0.9238795325112869605, 1.000000000000000000, 0.9238795325112869605, 1.000000000000000000, 0.9238795325112869605, 1.000000000000000000, 0.9238795325112869605, 1.000000000000000000, 0.9238795325112869605, 1.000000000000000000, 0.9238795325112869605, 1.000000000000000000, 0.9238795325112869605, 1.000000000000000000, 0.9238795325112869605, 1.000000000000000000, 0.9238795325112869605, 1.000000000000000000, 0.9238795325112869605, 1.000000000000000000, 0.9238795325112869605, 1.000000000000000000, 0.9238795325112869605, 1.000000000000000000, 0.9238795325112869605, 1.000000000000000000, 0.9238795325112869605, 1.000000000000000000, 0.9238795325112869605, 1.000000000000000000) ) ) 
 REPRESENTATION_ITEM ( '' )  SURFACE ( )  );
#2599=CARTESIAN_POINT ( 'NONE',  ( 107.4960827545248350, -6.936859964151250502, -8.388885654883777576 ) ) ;
#2600=CARTESIAN_POINT ( 'NONE',  ( 115.8999108795247821, -1.325403438956436419, -16.93181055722138595 ) ) ;
#2610=CARTESIAN_POINT ( 'NONE',  ( 70.27122018245525226, -26.36473080579375861, -5.633705330403472544 ) ) ;
#2612=EDGE_CURVE ( 'NONE', #7036, #28148, #18318, .T. ) ;
#2617=CARTESIAN_POINT ( 'NONE',  ( 114.5803015045248117, -2.477300249445798297, -7.631215200338321125 ) ) ;
#2621=CARTESIAN_POINT ( 'NONE',  ( 113.8163171295247764, 0.1403307496149613920, -13.39321520033831447 ) ) ;
#2625=CARTESIAN_POINT ( 'NONE',  ( 111.3160046295247838, -4.863998795839590272, -7.631215200338315796 ) ) ;
#2626=CARTESIAN_POINT ( 'NONE',  ( 117.2294421295247844, -10.76310523276723785, -5.182735500338556456 ) ) ;
#2627=CARTESIAN_POINT ( 'NONE',  ( 112.4967077545247633, -7.250697342233347165, -7.631215200338321125 ) ) ;
#2630=CARTESIAN_POINT ( 'NONE',  ( 115.3931121053768436, 0.3967854368539331933, -16.28112951403852549 ) ) ;
#2644=CARTESIAN_POINT ( 'NONE',  ( 110.8298327545248299, -6.936859964151250502, -8.388885654883777576 ) ) ;
#2646=CARTESIAN_POINT ( 'NONE',  ( 116.8546682094391400, -0.5381813604855363309, -16.38644560622362434 ) ) ;
#2647=CARTESIAN_POINT ( 'NONE',  ( 66.19909219943727408, -62.82237896425675672, -47.71602681600973739 ) ) ;
#2654=CARTESIAN_POINT ( 'NONE',  ( 117.0590115223097030, 1.678907146655578053, -5.492932798708517694 ) ) ;
#2655=CARTESIAN_POINT ( 'NONE',  ( 114.0440301496069821, 0.3591747506842615789, -14.64321520033831447 ) ) ;
#2656=CARTESIAN_POINT ( 'NONE',  ( 109.1629577545248395, -2.791137627527939813, -18.39754474579286025 ) ) ;
#2657=CARTESIAN_POINT ( 'NONE',  ( 111.2647481608379820, 0.3867979994853637526, -14.64321520033833757 ) ) ;
#2660=LINE ( 'NONE', #10200, #44967 ) ;
#2672=CARTESIAN_POINT ( 'NONE',  ( 112.4272546295247821, -4.863998795839590272, -7.631215200338315796 ) ) ;
#2673=CARTESIAN_POINT ( 'NONE',  ( 105.2735827545248810, -6.936859964151250502, -8.388885654883777576 ) ) ;
#2674=CARTESIAN_POINT ( 'NONE',  ( 115.9693640045247776, -10.62599879583958717, -11.00651665394454604 ) ) ;
#2677=CARTESIAN_POINT ( 'NONE',  ( 112.9389878519202739, 0.2518737723193609224, -12.14321520033831625 ) ) ;
#2679=CARTESIAN_POINT ( 'NONE',  ( 114.5108483795247878, -8.402594152722688392, -16.93181055722141792 ) ) ;
#2688=CARTESIAN_POINT ( 'NONE',  ( 116.6091619947073070, -11.87124904611273735, -21.21647875974084840 ) ) ;
#2694=FILL_AREA_STYLE ('',( #16392 ) ) ;
#2695=LINE ( 'NONE', #16855, #1686 ) ;
#2699=CARTESIAN_POINT ( 'NONE',  ( 109.9963952545248134, -9.868328341294098749, -15.46607636864997204 ) ) ;
#2726=AXIS2_PLACEMENT_3D ( 'NONE', #41402, #17220, #20195 ) ;
#2730=CARTESIAN_POINT ( 'NONE',  ( 113.8857702545248003, -10.62599879583958717, -15.77991374673208469 ) ) ;
#2732=CARTESIAN_POINT ( 'NONE',  ( 106.1764733795248219, -1.325403438956436419, -9.854619843455211026 ) ) ;
#2733=LINE ( 'NONE', #16658, #34177 ) ;
#2734=CARTESIAN_POINT ( 'NONE',  ( 109.5102233795247884, -8.938348069036441856, -17.46756447353520869 ) ) ;
#2743=CARTESIAN_POINT ( 'NONE',  ( 106.2459265045248173, -7.250697342233347165, -19.15521520033831138 ) ) ;
#2767=CARTESIAN_POINT ( 'NONE',  ( 114.0246765045248196, -7.250697342233347165, -19.15521520033831138 ) ) ;
#2769=ORIENTED_EDGE ( 'NONE', *, *, #28952, .T. ) ;
#2788=CARTESIAN_POINT ( 'NONE',  ( 109.3713171295247832, -10.62599879583958540, -13.39321520033831447 ) ) ;
#2789=CARTESIAN_POINT ( 'NONE',  ( 115.1359265045248605, -2.791137627527939813, -8.388885654883777576 ) ) ;
#2790=CARTESIAN_POINT ( 'NONE',  ( 108.1211608795247798, -8.938348069036489818, -9.318865927141430916 ) ) ;
#2793=ORIENTED_EDGE ( 'NONE', *, *, #28718, .T. ) ;
#2798=B_SPLINE_CURVE_WITH_KNOTS ( 'NONE', 3,
 ( #31205, #41491, #37603, #20285, #17095, #6595, #34169, #23938, #30987, #20512, #38048, #6826, #13670, #27578, #23249, #37131, #5907, #21840, #4508, #32322, #21168, #42597, #11360, #41708, #17971, #25269, #41928, #39166 ),
 .UNSPECIFIED., .F., .F.,
 ( 4, 2, 2, 1, 1, 1, 1, 1, 2, 2, 2, 1, 1, 1, 1, 1, 2, 2, 4 ),
 ( 0.000000000000000000, 0.2499999999998344657, 0.3749999999997541411, 0.4374999999997165046, 0.4687499999996964650, 0.4843749999996863620, 0.4921874999996825317, 0.4960937499996794786, 0.4980468749996780353, 0.4999999999996767031, 0.6249999999994826361, 0.6874999999993886002, 0.7187499999993398614, 0.7343749999993155475, 0.7421874999993045563, 0.7460937499993005595, 0.7480468749993014477, 0.7499999999993022248, 1.000000000000000000 ),
 .UNSPECIFIED. ) ;
#2807=CARTESIAN_POINT ( 'NONE',  ( 107.3571765045248299, -2.791137627527939813, -8.388885654883777576 ) ) ;
#2808=CARTESIAN_POINT ( 'NONE',  ( 113.4690515045247992, -6.936859964151250502, -18.39754474579286025 ) ) ;
#2813=ADVANCED_FACE ( 'NONE', ( #31081 ), #38144, .T. ) ;
#2824=CYLINDRICAL_SURFACE ( 'NONE', #38413, 15.90000000000000036 ) ;
#2829=CARTESIAN_POINT ( 'NONE',  ( 109.7880358795247986, -8.402594152722688392, -9.854619843455216355 ) ) ;
#2830=CARTESIAN_POINT ( 'NONE',  ( 114.9716510812576757, -0.01829820670803256055, -12.14321520033831625 ) ) ;
#2840=CARTESIAN_POINT ( 'NONE',  ( 114.2334337908067710, 0.5115630086001619059, -12.14321520033831625 ) ) ;
#2847=CARTESIAN_POINT ( 'NONE',  ( 107.2182702545248105, 0.1403307496149616695, -11.32035403202665336 ) ) ;
#2851=CARTESIAN_POINT ( 'NONE',  ( 114.7886608795247696, -1.325403438956436419, -16.93181055722141792 ) ) ;
#2855=CARTESIAN_POINT ( 'NONE',  ( 87.44708369096657918, -25.99489077589588604, -13.39321520033831447 ) ) ;
#2857=CARTESIAN_POINT ( 'NONE',  ( 112.3578015045248861, -2.477300249445798297, -7.631215200338321125 ) ) ;
#2861=( BOUNDED_CURVE ( )  B_SPLINE_CURVE ( 3, ( #30022, #33413, #2647, #9281 ),
 .UNSPECIFIED., .F., .T. ) 
 B_SPLINE_CURVE_WITH_KNOTS ( ( 4, 4 ),
 ( 2.411864997362825225, 3.141592653589795336 ),
 .UNSPECIFIED. ) 
 CURVE ( )  GEOMETRIC_REPRESENTATION_ITEM ( )  RATIONAL_B_SPLINE_CURVE ( ( 1.000000000000000000, 0.9561149059751439250, 0.9561149059751439250, 1.000000000000000000 ) ) 
 REPRESENTATION_ITEM ( '' )  );
#2865=VERTEX_POINT ( 'NONE', #13544 ) ;
#2875=CARTESIAN_POINT ( 'NONE',  ( 112.4272546295247821, -4.863998795839590272, -18.39754474579285315 ) ) ;
#2876=EDGE_CURVE ( 'NONE', #13043, #17886, #27453, .T. ) ;
#2880=CARTESIAN_POINT ( 'NONE',  ( 112.4272546295247821, -4.863998795839590272, -7.631215200338315796 ) ) ;
#2881=ORIENTED_EDGE ( 'NONE', *, *, #1026, .T. ) ;
#2884=CARTESIAN_POINT ( 'NONE',  ( 112.9327801496069696, 0.3591747506842615789, -14.64321520033830026 ) ) ;
#2886=DIRECTION ( 'NONE',  ( -8.728168432587710164E-16, -1.000000000000000000, 0.000000000000000000 ) ) ;
#2888=CARTESIAN_POINT ( 'NONE',  ( 113.7722331777918896, -0.01829820670813664396, -14.64321520033831447 ) ) ;
#2889=CARTESIAN_POINT ( 'NONE',  ( 105.8986608795248401, -1.325403438956436419, -16.93181055722141792 ) ) ;
#2890=FACE_BOUND ( 'NONE', #40393, .T. ) ;
#2893=DIRECTION ( 'NONE',  ( 0.000000000000000000, 0.000000000000000000, 1.000000000000000000 ) ) ;
#2900=CARTESIAN_POINT ( 'NONE',  ( 62.57015527438819191, -24.33598972801448923, -4.893215200338314474 ) ) ;
#2903=CARTESIAN_POINT ( 'NONE',  ( 109.7185827545247889, -2.477300249445798297, -19.15521520033831138 ) ) ;
#2904=CARTESIAN_POINT ( 'NONE',  ( 61.85703706989207973, -38.82652229419164769, -6.037231199156998684 ) ) ;
#2905=FACE_OUTER_BOUND ( 'NONE', #38733, .T. ) ;
#2909=CARTESIAN_POINT ( 'NONE',  ( 115.2053796295247849, -4.863998795839590272, -8.388885654883775800 ) ) ;
#2918=CARTESIAN_POINT ( 'NONE',  ( 105.3430358795248338, -8.402594152722688392, -9.854619843455216355 ) ) ;
#2919=ORIENTED_EDGE ( 'NONE', *, *, #17248, .F. ) ;
#2924=PRESENTATION_STYLE_ASSIGNMENT (( #2238 ) ) ;
#2929=CARTESIAN_POINT ( 'NONE',  ( 106.1070202545248407, 0.1403307496149616695, -11.32035403202665336 ) ) ;
#2937=ORIENTED_EDGE ( 'NONE', *, *, #31128, .F. ) ;
#2939=AXIS2_PLACEMENT_3D ( 'NONE', #32208, #7594, #14897 ) ;
#2947=CIRCLE ( 'NONE', #23364, 5.000000000000004441 ) ;
#2948=DIRECTION ( 'NONE',  ( 0.000000000000000000, 1.000000000000000000, 0.000000000000000000 ) ) ;
#2959=CARTESIAN_POINT ( 'NONE',  ( 107.1488171295247867, -10.62599879583958540, -13.39321520033831447 ) ) ;
#2960=CARTESIAN_POINT ( 'NONE',  ( 106.6626452545248611, -9.868328341294098749, -15.46607636864997204 ) ) ;
#2961=CARTESIAN_POINT ( 'NONE',  ( 106.8710046295248759, -4.863998795839590272, -18.39754474579285315 ) ) ;
#2970=CARTESIAN_POINT ( 'NONE',  ( 106.6626452545248611, 0.8980012041604421569, -11.00651665394454071 ) ) ;
#2972=ORIENTED_EDGE ( 'NONE', *, *, #25320, .F. ) ;
#2982=EDGE_LOOP ( 'NONE', ( #44977, #36661, #11961, #42449 ) ) ;
#2983=CARTESIAN_POINT ( 'NONE',  ( 116.5945156689966922, -9.863253977036384512, -13.30267646073255250 ) ) ;
#2992=CARTESIAN_POINT ( 'NONE',  ( 111.8716296295247901, -4.863998795839590272, -19.15521520033831493 ) ) ;
#2995=ORIENTED_EDGE ( 'NONE', *, *, #8638, .T. ) ;
#3001=CARTESIAN_POINT ( 'NONE',  ( 70.36267391504962632, -5.685877709920933221, -21.89321520033831447 ) ) ;
#3015=CARTESIAN_POINT ( 'NONE',  ( 106.8015515045248378, -2.477300249445798297, -7.631215200338321125 ) ) ;
#3017=CARTESIAN_POINT ( 'NONE',  ( 114.0941296295247867, -4.863998795839590272, -8.388885654883775800 ) ) ;
#3018=CARTESIAN_POINT ( 'NONE',  ( 107.2182702545248105, -10.62599879583958717, -15.77991374673208469 ) ) ;
#3025=DIRECTION ( 'NONE',  ( 1.000000000000000000, 0.000000000000000000, 0.000000000000000000 ) ) ;
#3033=CARTESIAN_POINT ( 'NONE',  ( 107.4266296295248821, -4.863998795839590272, -19.15521520033831493 ) ) ;
#3038=CARTESIAN_POINT ( 'NONE',  ( 109.7880358795247986, -8.402594152722688392, -9.854619843455216355 ) ) ;
#3039=CARTESIAN_POINT ( 'NONE',  ( 107.9128015045248219, -6.936859964151250502, -18.39754474579286025 ) ) ;
#3047=DIRECTION ( 'NONE',  ( 0.000000000000000000, 0.000000000000000000, -1.000000000000000000 ) ) ;
#3049=DIRECTION ( 'NONE',  ( -1.000000000000000000, 0.000000000000000000, 0.000000000000000000 ) ) ;
#3058=EDGE_CURVE ( 'NONE', #13698, #24351, #14650, .T. ) ;
#3059=CARTESIAN_POINT ( 'NONE',  ( 115.2053796295247849, -4.863998795839590272, -19.15521520033831493 ) ) ;
#3065=EDGE_LOOP ( 'NONE', ( #38219, #3508, #17725 ) ) ;
#3066=CARTESIAN_POINT ( 'NONE',  ( 116.1082702545247827, 0.1403307496149616695, -11.32035403202665336 ) ) ;
#3067=CARTESIAN_POINT ( 'NONE',  ( 116.4114176093651878, 0.5600166689815611054, -14.64321520033831447 ) ) ;
#3068=CARTESIAN_POINT ( 'NONE',  ( 112.3578015045248719, -2.477300249445798297, -7.631215200338321125 ) ) ;
#3070=CARTESIAN_POINT ( 'NONE',  ( 66.38809756183205479, -36.79083284667497367, -4.893215200338314474 ) ) ;
#3073=EDGE_LOOP ( 'NONE', ( #19466, #6837, #32313, #23665 ) ) ;
#3076=CARTESIAN_POINT ( 'NONE',  ( 115.4831921295247952, 0.8980012041604618078, -13.39321520033831447 ) ) ;
#3081=CARTESIAN_POINT ( 'NONE',  ( 115.7610046295247912, -4.863998795839590272, -18.39754474579285315 ) ) ;
#3085=CARTESIAN_POINT ( 'NONE',  ( 107.8433483795247838, -0.7896495226426338832, -9.318865927141430916 ) ) ;
#3087=CARTESIAN_POINT ( 'NONE',  ( 112.8439733795247832, -8.938348069036489818, -17.46756447353520159 ) ) ;
#3090=DIRECTION ( 'NONE',  ( 0.000000000000000000, 0.000000000000000000, 1.000000000000000000 ) ) ;
#3094=ORIENTED_EDGE ( 'NONE', *, *, #6249, .F. ) ;
#3100=ORIENTED_EDGE ( 'NONE', *, *, #43789, .T. ) ;
#3106=CARTESIAN_POINT ( 'NONE',  ( 116.8417075039013184, -0.9679852802911167453, -16.90817056666675811 ) ) ;
#3107=CARTESIAN_POINT ( 'NONE',  ( 114.3719421295247827, 0.8980012041604618078, -13.39321520033831447 ) ) ;
#3109=PRODUCT_DEFINITION_FORMATION_WITH_SPECIFIED_SOURCE ( 'ANY', '', #10664, .NOT_KNOWN. ) ;
#3111=CARTESIAN_POINT ( 'NONE',  ( 113.0776676093651929, 0.5600166689815611054, -14.64321520033833579 ) ) ;
#3112=CARTESIAN_POINT ( 'NONE',  ( 117.0111608795247946, -1.325403438956436419, -16.93181055722141792 ) ) ;
#3113=AXIS2_PLACEMENT_3D ( 'NONE', #37307, #23420, #36848 ) ;
#3117=CARTESIAN_POINT ( 'NONE',  ( 107.9128015045248219, -6.936859964151250502, -18.39754474579286025 ) ) ;
#3119=CARTESIAN_POINT ( 'NONE',  ( 111.5023434012278898, 0.04929351793716424401, -14.64321520033831447 ) ) ;
#3131=( BOUNDED_SURFACE ( )  B_SPLINE_SURFACE ( 1, 2, ( 
 ( #17394, #34902, #947, #31282, #17832, #31949, #31729, #10553, #55, #35591, #28774, #3913, #14411, #499, #18058, #31505, #42682, #28553, #714, #277, #13969, #25356, #10997, #21922, #27881, #14187, #42233, #3691, #21477, #21253, #14635, #24898, #38791, #39250, #21029, #28106, #7563, #35132, #35362, #14865, #41795, #4137, #7795, #38342, #42458, #11223, #8015, #10775, #25129, #7119, #17613, #39024, #21704, #24671, #4361, #7334, #18281, #38558, #4587, #32400, #43124, #29890, #11893, #29435, #22150, #25575, #23049, #25795, #8243, #5263, #5036, #12120, #15530, #36493, #29214, #1171, #15986, #43350, #8917, #26022, #43575, #39704, #28997, #12345, #18950, #9143, #11667, #39479, #18510, #15086, #36042, #33287, #42905, #32841, #19179, #1609, #4811, #18732, #22818, #43806, #36268, #39928, #8688, #33058, #15306, #12573, #1391, #32625, #22593, #8469, #22372, #26243, #40155, #1831, #15761, #29662, #26477, #36710, #5479, #19400, #2062, #40382, #33507, #20312, #33745, #20535, #12797, #34415, #13475, #9367, #2515, #9596, #30563, #37631, #5706, #2287, #31009, #10275, #6622, #17120, #16441, #34196, #23963, #2970, #10060, #3196, #44482, #44939, #27377, #2743, #26920, #41300, #37848, #23276, #30342, #13249, #16667, #27151, #44265, #27604, #16216 ),
 ( #16898, #23512, #41073, #44034, #9830, #23740, #30120, #13696, #6404, #41518, #30791, #44715, #36935, #19623, #13022, #26698, #40609, #37158, #5934, #37399, #19857, #40841, #6169, #20089, #33975, #14807, #3853, #20757, #28495, #3422, #17998, #25070, #31669, #38286, #32119, #14130, #28720, #34636, #14355, #41733, #17553, #7065, #24398, #20976, #31896, #21417, #10497, #42401, #662, #887, #10937, #38962, #4073, #31229, #34849, #24619, #3635, #6850, #28268, #42626, #24180, #17776, #28046, #38072, #13910, #31447, #41954, #10719, #14578, #27821, #11165, #38502, #35302, #1, #24840, #7279, #7731, #38731, #35531, #217, #21195, #35072, #21642, #438, #4303, #42177, #17339, #7502, #18225, #36217, #18458, #33238, #8640, #22540, #19124, #39874, #1557, #5433, #43525, #1782, #43070, #15937, #33007, #32570, #29609, #7957, #15480, #28942, #4757, #25521, #11610, #39424, #5205, #36437, #42851, #12293, #15707, #19351, #43298, #26193, #40100, #32348, #8189, #11838, #22098, #39191, #29385, #29836, #11388, #4982, #1336, #2012, #1114, #35986, #15251, #29157, #8859, #15031, #22761, #25746, #36660, #18678, #12067, #39652, #25299, #25969, #21868, #8415, #22320, #18894, #35763, #32786, #4534, #12975, #2918, #26419, #43755, #26870, #36884, #44664, #16619 ) ),
 .UNSPECIFIED., .F., .F., .F. ) 
 B_SPLINE_SURFACE_WITH_KNOTS ( ( 2, 2 ),
 ( 3, 2, 2, 2, 2, 2, 2, 2, 2, 2, 2, 2, 2, 2, 2, 2, 2, 2, 2, 2, 2, 2, 2, 2, 2, 2, 2, 2, 2, 2, 2, 2, 2, 2, 2, 2, 2, 2, 2, 2, 2, 2, 2, 2, 2, 2, 2, 2, 2, 2, 2, 2, 2, 2, 2, 2, 2, 2, 2, 2, 2, 2, 2, 2, 2, 2, 2, 2, 2, 2, 2, 2, 2, 2, 2, 2, 2, 2, 2, 2, 3 ),
 ( 0.000000000000000000, 1.000000000000000000 ),
 ( 0.000000000000000000, 0.01250000000000000069, 0.02500000000000000139, 0.03749999999999999861, 0.05000000000000000278, 0.06250000000000000000, 0.07499999999999999722, 0.08749999999999999445, 0.1000000000000000056, 0.1125000000000000028, 0.1250000000000000000, 0.1375000000000000111, 0.1499999999999999944, 0.1625000000000000056, 0.1749999999999999889, 0.1875000000000000000, 0.2000000000000000111, 0.2124999999999999944, 0.2250000000000000056, 0.2374999999999999889, 0.2500000000000000000, 0.2625000000000000111, 0.2750000000000000222, 0.2874999999999999778, 0.2999999999999999889, 0.3125000000000000000, 0.3250000000000000111, 0.3375000000000000222, 0.3499999999999999778, 0.3624999999999999889, 0.3750000000000000000, 0.3875000000000000111, 0.4000000000000000222, 0.4124999999999999778, 0.4249999999999999889, 0.4375000000000000000, 0.4500000000000000111, 0.4625000000000000222, 0.4749999999999999778, 0.4874999999999999889, 0.5000000000000000000, 0.5124999999999999556, 0.5250000000000000222, 0.5374999999999999778, 0.5500000000000000444, 0.5625000000000000000, 0.5749999999999999556, 0.5875000000000000222, 0.5999999999999999778, 0.6125000000000000444, 0.6250000000000000000, 0.6374999999999999556, 0.6500000000000000222, 0.6624999999999999778, 0.6750000000000000444, 0.6875000000000000000, 0.6999999999999999556, 0.7125000000000000222, 0.7249999999999999778, 0.7375000000000000444, 0.7500000000000000000, 0.7624999999999999556, 0.7750000000000000222, 0.7874999999999999778, 0.8000000000000000444, 0.8125000000000000000, 0.8249999999999999556, 0.8375000000000000222, 0.8499999999999999778, 0.8625000000000000444, 0.8750000000000000000, 0.8874999999999999556, 0.9000000000000000222, 0.9124999999999999778, 0.9250000000000000444, 0.9375000000000000000, 0.9499999999999999556, 0.9625000000000000222, 0.9749999999999999778, 0.9875000000000000444, 1.000000000000000000 ),
 .UNSPECIFIED. ) 
 GEOMETRIC_REPRESENTATION_ITEM ( )  RATIONAL_B_SPLINE_SURFACE ( (
 ( 1.000000000000000000, 0.9238795325112869605, 1.000000000000000000, 0.9238795325112869605, 1.000000000000000000, 0.9238795325112869605, 1.000000000000000000, 0.9238795325112869605, 1.000000000000000000, 0.9238795325112869605, 1.000000000000000000, 0.9238795325112869605, 1.000000000000000000, 0.9238795325112869605, 1.000000000000000000, 0.9238795325112869605, 1.000000000000000000, 0.9238795325112869605, 1.000000000000000000, 0.9238795325112869605, 1.000000000000000000, 0.9238795325112869605, 1.000000000000000000, 0.9238795325112869605, 1.000000000000000000, 0.9238795325112869605, 1.000000000000000000, 0.9238795325112869605, 1.000000000000000000, 0.9238795325112869605, 1.000000000000000000, 0.9238795325112869605, 1.000000000000000000, 0.9238795325112869605, 1.000000000000000000, 0.9238795325112869605, 1.000000000000000000, 0.9238795325112869605, 1.000000000000000000, 0.9238795325112869605, 1.000000000000000000, 0.9238795325112869605, 1.000000000000000000, 0.9238795325112869605, 1.000000000000000000, 0.9238795325112869605, 1.000000000000000000, 0.9238795325112869605, 1.000000000000000000, 0.9238795325112869605, 1.000000000000000000, 0.9238795325112869605, 1.000000000000000000, 0.9238795325112869605, 1.000000000000000000, 0.9238795325112869605, 1.000000000000000000, 0.9238795325112869605, 1.000000000000000000, 0.9238795325112869605, 1.000000000000000000, 0.9238795325112869605, 1.000000000000000000, 0.9238795325112869605, 1.000000000000000000, 0.9238795325112869605, 1.000000000000000000, 0.9238795325112869605, 1.000000000000000000, 0.9238795325112869605, 1.000000000000000000, 0.9238795325112869605, 1.000000000000000000, 0.9238795325112869605, 1.000000000000000000, 0.9238795325112869605, 1.000000000000000000, 0.9238795325112869605, 1.000000000000000000, 0.9238795325112869605, 1.000000000000000000, 0.9238795325112869605, 1.000000000000000000, 0.9238795325112869605, 1.000000000000000000, 0.9238795325112869605, 1.000000000000000000, 0.9238795325112869605, 1.000000000000000000, 0.9238795325112869605, 1.000000000000000000, 0.9238795325112869605, 1.000000000000000000, 0.9238795325112869605, 1.000000000000000000, 0.9238795325112869605, 1.000000000000000000, 0.9238795325112869605, 1.000000000000000000, 0.9238795325112869605, 1.000000000000000000, 0.9238795325112869605, 1.000000000000000000, 0.9238795325112869605, 1.000000000000000000, 0.9238795325112869605, 1.000000000000000000, 0.9238795325112869605, 1.000000000000000000, 0.9238795325112869605, 1.000000000000000000, 0.9238795325112869605, 1.000000000000000000, 0.9238795325112869605, 1.000000000000000000, 0.9238795325112869605, 1.000000000000000000, 0.9238795325112869605, 1.000000000000000000, 0.9238795325112869605, 1.000000000000000000, 0.9238795325112869605, 1.000000000000000000, 0.9238795325112869605, 1.000000000000000000, 0.9238795325112869605, 1.000000000000000000, 0.9238795325112869605, 1.000000000000000000, 0.9238795325112869605, 1.000000000000000000, 0.9238795325112869605, 1.000000000000000000, 0.9238795325112869605, 1.000000000000000000, 0.9238795325112869605, 1.000000000000000000, 0.9238795325112869605, 1.000000000000000000, 0.9238795325112869605, 1.000000000000000000, 0.9238795325112869605, 1.000000000000000000, 0.9238795325112869605, 1.000000000000000000, 0.9238795325112869605, 1.000000000000000000, 0.9238795325112869605, 1.000000000000000000, 0.9238795325112869605, 1.000000000000000000, 0.9238795325112869605, 1.000000000000000000, 0.9238795325112869605, 1.000000000000000000, 0.9238795325112869605, 1.000000000000000000, 0.9238795325112869605, 1.000000000000000000, 0.9238795325112869605, 1.000000000000000000),
 ( 1.000000000000000000, 0.9238795325112869605, 1.000000000000000000, 0.9238795325112869605, 1.000000000000000000, 0.9238795325112869605, 1.000000000000000000, 0.9238795325112869605, 1.000000000000000000, 0.9238795325112869605, 1.000000000000000000, 0.9238795325112869605, 1.000000000000000000, 0.9238795325112869605, 1.000000000000000000, 0.9238795325112869605, 1.000000000000000000, 0.9238795325112869605, 1.000000000000000000, 0.9238795325112869605, 1.000000000000000000, 0.9238795325112869605, 1.000000000000000000, 0.9238795325112869605, 1.000000000000000000, 0.9238795325112869605, 1.000000000000000000, 0.9238795325112869605, 1.000000000000000000, 0.9238795325112869605, 1.000000000000000000, 0.9238795325112869605, 1.000000000000000000, 0.9238795325112869605, 1.000000000000000000, 0.9238795325112869605, 1.000000000000000000, 0.9238795325112869605, 1.000000000000000000, 0.9238795325112869605, 1.000000000000000000, 0.9238795325112869605, 1.000000000000000000, 0.9238795325112869605, 1.000000000000000000, 0.9238795325112869605, 1.000000000000000000, 0.9238795325112869605, 1.000000000000000000, 0.9238795325112869605, 1.000000000000000000, 0.9238795325112869605, 1.000000000000000000, 0.9238795325112869605, 1.000000000000000000, 0.9238795325112869605, 1.000000000000000000, 0.9238795325112869605, 1.000000000000000000, 0.9238795325112869605, 1.000000000000000000, 0.9238795325112869605, 1.000000000000000000, 0.9238795325112869605, 1.000000000000000000, 0.9238795325112869605, 1.000000000000000000, 0.9238795325112869605, 1.000000000000000000, 0.9238795325112869605, 1.000000000000000000, 0.9238795325112869605, 1.000000000000000000, 0.9238795325112869605, 1.000000000000000000, 0.9238795325112869605, 1.000000000000000000, 0.9238795325112869605, 1.000000000000000000, 0.9238795325112869605, 1.000000000000000000, 0.9238795325112869605, 1.000000000000000000, 0.9238795325112869605, 1.000000000000000000, 0.9238795325112869605, 1.000000000000000000, 0.9238795325112869605, 1.000000000000000000, 0.9238795325112869605, 1.000000000000000000, 0.9238795325112869605, 1.000000000000000000, 0.9238795325112869605, 1.000000000000000000, 0.9238795325112869605, 1.000000000000000000, 0.9238795325112869605, 1.000000000000000000, 0.9238795325112869605, 1.000000000000000000, 0.9238795325112869605, 1.000000000000000000, 0.9238795325112869605, 1.000000000000000000, 0.9238795325112869605, 1.000000000000000000, 0.9238795325112869605, 1.000000000000000000, 0.9238795325112869605, 1.000000000000000000, 0.9238795325112869605, 1.000000000000000000, 0.9238795325112869605, 1.000000000000000000, 0.9238795325112869605, 1.000000000000000000, 0.9238795325112869605, 1.000000000000000000, 0.9238795325112869605, 1.000000000000000000, 0.9238795325112869605, 1.000000000000000000, 0.9238795325112869605, 1.000000000000000000, 0.9238795325112869605, 1.000000000000000000, 0.9238795325112869605, 1.000000000000000000, 0.9238795325112869605, 1.000000000000000000, 0.9238795325112869605, 1.000000000000000000, 0.9238795325112869605, 1.000000000000000000, 0.9238795325112869605, 1.000000000000000000, 0.9238795325112869605, 1.000000000000000000, 0.9238795325112869605, 1.000000000000000000, 0.9238795325112869605, 1.000000000000000000, 0.9238795325112869605, 1.000000000000000000, 0.9238795325112869605, 1.000000000000000000, 0.9238795325112869605, 1.000000000000000000, 0.9238795325112869605, 1.000000000000000000, 0.9238795325112869605, 1.000000000000000000, 0.9238795325112869605, 1.000000000000000000, 0.9238795325112869605, 1.000000000000000000, 0.9238795325112869605, 1.000000000000000000, 0.9238795325112869605, 1.000000000000000000) ) ) 
 REPRESENTATION_ITEM ( '' )  SURFACE ( )  );
#3132=CONICAL_SURFACE ( 'NONE', #14782, 5.000000000000000888, 0.7853981633974419507 ) ;
#3134=CARTESIAN_POINT ( 'NONE',  ( 112.2188952545247531, 0.8980012041604421569, -11.00651665394454071 ) ) ;
#3136=CARTESIAN_POINT ( 'NONE',  ( 82.85213572415328542, -31.80476018815861394, -23.17883450557113179 ) ) ;
#3138=AXIS2_PLACEMENT_3D ( 'NONE', #23330, #40897, #13907 ) ;
#3143=CARTESIAN_POINT ( 'NONE',  ( 109.3018640045248304, 0.1403307496149616695, -15.46607636864997204 ) ) ;
#3157=CARTESIAN_POINT ( 'NONE',  ( 84.86020291624612355, -29.99489077589588959, -18.39321520033831803 ) ) ;
#3160=CARTESIAN_POINT ( 'NONE',  ( 108.2600671295247992, 0.1403307496149613920, -13.39321520033831447 ) ) ;
#3162=DIRECTION ( 'NONE',  ( 1.000000000000000000, 0.000000000000000000, 0.000000000000000000 ) ) ;
#3177=CARTESIAN_POINT ( 'NONE',  ( 64.01282776924008999, -34.86145050234443943, -5.893215200338315363 ) ) ;
#3185=CARTESIAN_POINT ( 'NONE',  ( 108.5378796295247810, -4.863998795839590272, -19.15521520033831493 ) ) ;
#3186=CARTESIAN_POINT ( 'NONE',  ( 107.0793640045248196, 0.1403307496149616695, -15.46607636864997204 ) ) ;
#3187=CARTESIAN_POINT ( 'NONE',  ( 106.1070202545248407, 0.1403307496149616695, -11.32035403202665336 ) ) ;
#3191=VERTEX_POINT ( 'NONE', #22162 ) ;
#3194=DIRECTION ( 'NONE',  ( 0.000000000000000000, 0.000000000000000000, 1.000000000000000000 ) ) ;
#3196=CARTESIAN_POINT ( 'NONE',  ( 106.5237390045248418, 0.8980012041604421569, -15.77991374673208469 ) ) ;
#3203=CARTESIAN_POINT ( 'NONE',  ( 74.69189222814998175, -41.76310523276723785, -19.39321520033831447 ) ) ;
#3216=CARTESIAN_POINT ( 'NONE',  ( 108.8156921295247912, 0.8980012041604618078, -13.39321520033831447 ) ) ;
#3223=CARTESIAN_POINT ( 'NONE',  ( 69.69189222814998175, -41.76310523276723785, -4.893215200338314474 ) ) ;
#3227=B_SPLINE_CURVE_WITH_KNOTS ( 'NONE', 3,
 ( #27995, #28664, #21362, #24568, #387, #22038, #35245, #41900, #7224, #42568, #32293, #14973, #39370, #11330, #4700, #1058, #11559, #25466, #10885, #4022, #42349, #8137, #21138, #35014, #3794, #17944, #17720, #612, #31618, #14300, #25010, #40035, #22931, #19517, #19739 ),
 .UNSPECIFIED., .F., .F.,
 ( 4, 2, 2, 1, 1, 2, 2, 2, 2, 1, 1, 2, 2, 2, 2, 1, 1, 1, 2, 2, 4 ),
 ( 0.000000000000000000, 0.1250000000001383060, 0.1875000000002075840, 0.2187500000002391698, 0.2343750000002570721, 0.2421875000002660372, 0.2500000000002749467, 0.3750000000004191647, 0.4375000000004898859, 0.4687500000005253020, 0.4843750000005431211, 0.4921875000005542233, 0.5000000000005653256, 0.6250000000006362688, 0.6875000000006702416, 0.7187500000006900036, 0.7343750000006985523, 0.7421875000007027712, 0.7460937500007075451, 0.7500000000007122081, 1.000000000000000000 ),
 .UNSPECIFIED. ) ;
#3237=CARTESIAN_POINT ( 'NONE',  ( 109.2324108795247923, -8.938348069036489818, -9.318865927141430916 ) ) ;
#3238=CARTESIAN_POINT ( 'NONE',  ( 107.0099108795247815, -1.325403438956436419, -16.93181055722141792 ) ) ;
#3239=CARTESIAN_POINT ( 'NONE',  ( 108.3989733795248753, -8.938348069036489818, -17.46756447353520159 ) ) ;
#3244=CARTESIAN_POINT ( 'NONE',  ( 112.2188952545247531, 0.8980012041604421569, -11.00651665394454071 ) ) ;
#3245=CARTESIAN_POINT ( 'NONE',  ( 117.2294421295247844, -10.76310523276723785, -5.182735500338556456 ) ) ;
#3247=CARTESIAN_POINT ( 'NONE',  ( 61.69189222814998175, -49.76310523276723785, -19.39321520033831447 ) ) ;
#3251=CARTESIAN_POINT ( 'NONE',  ( 107.2182702545248105, -10.62599879583958717, -15.77991374673208469 ) ) ;
#3257=CARTESIAN_POINT ( 'NONE',  ( 107.0793640045248196, 0.1403307496149616695, -15.46607636864997204 ) ) ;
#3258=CARTESIAN_POINT ( 'NONE',  ( 105.2735827545248810, -6.936859964151250502, -8.388885654883777576 ) ) ;
#3267=ORIENTED_EDGE ( 'NONE', *, *, #28125, .T. ) ;
#3272=EDGE_CURVE ( 'NONE', #34550, #30411, #21035, .T. ) ;
#3273=DIRECTION ( 'NONE',  ( 0.000000000000000000, 0.000000000000000000, 1.000000000000000000 ) ) ;
#3274=EDGE_CURVE ( 'NONE', #22330, #24697, #37528, .T. ) ;
#3281=CARTESIAN_POINT ( 'NONE',  ( 107.1488171295247867, 0.1403307496149613920, -13.39321520033831447 ) ) ;
#3282=CARTESIAN_POINT ( 'NONE',  ( 115.2748327545248657, -6.936859964151250502, -8.388885654883788234 ) ) ;
#3292=CARTESIAN_POINT ( 'NONE',  ( 65.66749702063913219, -36.20550398600038022, -5.467054258871666406 ) ) ;
#3298=CARTESIAN_POINT ( 'NONE',  ( 106.5931921295248372, -9.868328341294093420, -13.39321520033831447 ) ) ;
#3302=CARTESIAN_POINT ( 'NONE',  ( 108.7462390045248242, -9.868328341294098749, -11.32035403202665869 ) ) ;
#3304=CARTESIAN_POINT ( 'NONE',  ( 111.8716296295247901, -4.863998795839590272, -19.15521520033831493 ) ) ;
#3307=CARTESIAN_POINT ( 'NONE',  ( 107.7738952545248310, 0.8980012041604421569, -11.00651665394454071 ) ) ;
#3309=CARTESIAN_POINT ( 'NONE',  ( 109.9963952545248134, 0.8980012041604421569, -11.00651665394454071 ) ) ;
#3312=CARTESIAN_POINT ( 'NONE',  ( 111.7308551332721862, 0.2334052082820642360, -14.64321520033831447 ) ) ;
#3317=EDGE_CURVE ( 'NONE', #37700, #3191, #21724, .T. ) ;
#3330=B_SPLINE_CURVE_WITH_KNOTS ( 'NONE', 3,
 ( #18846, #19072, #30009, #39377, #8364, #12016, #43020, #29559, #29336, #26141 ),
 .UNSPECIFIED., .F., .F.,
 ( 4, 3, 3, 4 ),
 ( 0.000000000000000000, 0.0002476487219222790075, 0.0004952974148303519383, 0.0009534114850261680291 ),
 .UNSPECIFIED. ) ;
#3331=CARTESIAN_POINT ( 'NONE',  ( 113.3301452545248083, 0.8980012041604421569, -11.00651665394454071 ) ) ;
#3335=EDGE_CURVE ( 'NONE', #40778, #1801, #44847, .T. ) ;
#3336=PLANE ( 'NONE',  #14796 ) ;
#3337=CARTESIAN_POINT ( 'NONE',  ( 113.2226630180080775, 0.7607806665038616689, -14.64321520033831447 ) ) ;
#3338=PLANE ( 'NONE',  #32780 ) ;
#3344=CARTESIAN_POINT ( 'NONE',  ( 114.7192077545248594, -2.791137627527939813, -18.39754474579286025 ) ) ;
#3349=CARTESIAN_POINT ( 'NONE',  ( 70.19189222814998175, -42.69543048370626792, -27.04993751765913501 ) ) ;
#3358=CARTESIAN_POINT ( 'NONE',  ( 111.0381921295247878, 0.8980012041604618078, -13.39321520033831447 ) ) ;
#3359=CARTESIAN_POINT ( 'NONE',  ( 105.8292077545248446, -2.791137627527939813, -18.39754474579286025 ) ) ;
#3360=CARTESIAN_POINT ( 'NONE',  ( 114.0246765045248196, -7.250697342233347165, -19.15521520033831138 ) ) ;
#3365=CARTESIAN_POINT ( 'NONE',  ( 108.8156921295247912, -9.868328341294093420, -13.39321520033831447 ) ) ;
#3371=ORIENTED_EDGE ( 'NONE', *, *, #3945, .F. ) ;
#3372=CARTESIAN_POINT ( 'NONE',  ( 113.3995983795247895, -0.7896495226426338832, -9.318865927141425587 ) ) ;
#3377=TOROIDAL_SURFACE ( 'NONE', #6271, 7.132259260909269649, 2.000000000000000000 ) ;
#3383=CARTESIAN_POINT ( 'NONE',  ( 107.2877233795247776, -1.325403438956436419, -9.854619843455211026 ) ) ;
#3392=CARTESIAN_POINT ( 'NONE',  ( 115.2748327545248657, -2.477300249445798297, -19.15521520033831138 ) ) ;
#3398=( BOUNDED_CURVE ( )  B_SPLINE_CURVE ( 2, ( #23731, #5697, #37622, #16433, #27143, #23038, #2734, #5926, #20303, #30553, #27369, #36925, #40600 ),
 .UNSPECIFIED., .F., .F. ) 
 B_SPLINE_CURVE_WITH_KNOTS ( ( 3, 2, 2, 2, 2, 2, 3 ),
 ( 0.6035091206787219775, 0.6125000000000000444, 0.6250000000000000000, 0.6374999999999999556, 0.6500000000000000222, 0.6624999999999999778, 0.6627876305315190120 ),
 .UNSPECIFIED. ) 
 CURVE ( )  GEOMETRIC_REPRESENTATION_ITEM ( )  RATIONAL_B_SPLINE_CURVE ( ( 0.9692594319298230010, 0.9452488050343769155, 1.000000000000000000, 0.9238795325112869605, 1.000000000000000000, 0.9238795325112869605, 1.000000000000000000, 0.9238795325112869605, 1.000000000000000000, 0.9238795325112869605, 1.000000000000000000, 0.9982484343581399244, 0.9965774773173300405 ) ) 
 REPRESENTATION_ITEM ( '' )  );
#3402=DIRECTION ( 'NONE',  ( 0.000000000000000000, 0.000000000000000000, -1.000000000000000000 ) ) ;
#3410=CARTESIAN_POINT ( 'NONE',  ( 107.6349890045248401, 0.8980012041604421569, -15.77991374673208469 ) ) ;
#3412=CARTESIAN_POINT ( 'NONE',  ( 106.5931921295248372, -9.868328341294093420, -13.39321520033831447 ) ) ;
#3413=CARTESIAN_POINT ( 'NONE',  ( 105.7597546295248350, -4.863998795839590272, -18.39754474579285315 ) ) ;
#3419=CYLINDRICAL_SURFACE ( 'NONE', #3138, 3.000000000000001332 ) ;
#3422=CARTESIAN_POINT ( 'NONE',  ( 114.0246765045248196, -2.791137627527939813, -8.388885654883777576 ) ) ;
#3425=CYLINDRICAL_SURFACE ( 'NONE', #13603, 15.90000000000000036 ) ;
#3442=CARTESIAN_POINT ( 'NONE',  ( 108.4684265045247997, -7.250697342233347165, -19.15521520033831138 ) ) ;
#3445=VERTEX_POINT ( 'NONE', #20228 ) ;
#3448=EDGE_CURVE ( 'NONE', #30411, #21756, #39528, .T. ) ;
#3449=FACE_OUTER_BOUND ( 'NONE', #19455, .T. ) ;
#3450=CARTESIAN_POINT ( 'NONE',  ( 74.19189222814998175, -41.76310523276723785, -24.39321520033831447 ) ) ;
#3461=ORIENTED_EDGE ( 'NONE', *, *, #25980, .F. ) ;
#3462=DIRECTION ( 'NONE',  ( 0.000000000000000000, 0.000000000000000000, 1.000000000000000000 ) ) ;
#3463=CARTESIAN_POINT ( 'NONE',  ( 107.0793640045248196, -10.62599879583958717, -11.00651665394454604 ) ) ;
#3464=CARTESIAN_POINT ( 'NONE',  ( 110.2742077545248094, -2.791137627527939813, -18.39754474579286025 ) ) ;
#3465=CARTESIAN_POINT ( 'NONE',  ( 108.8851452545248151, 0.8980012041604421569, -11.00651665394454071 ) ) ;
#3472=CARTESIAN_POINT ( 'NONE',  ( 112.0105358795247810, -0.7896495226426338832, -17.46756447353520159 ) ) ;
#3476=DIRECTION ( 'NONE',  ( 0.000000000000000000, -0.3713878862591641905, 0.9284778069183722282 ) ) ;
#3479=CARTESIAN_POINT ( 'NONE',  ( 106.4542858795248179, -0.7896495226426338832, -17.46756447353520159 ) ) ;
#3484=CARTESIAN_POINT ( 'NONE',  ( 115.9693640045247776, -10.62599879583958717, -11.00651665394454604 ) ) ;
#3485=CARTESIAN_POINT ( 'NONE',  ( 108.2600671295247992, 0.1403307496149613920, -13.39321520033831447 ) ) ;
#3498=CARTESIAN_POINT ( 'NONE',  ( 109.2294421295247844, 0.1210096558822565393, -14.64321520034217805 ) ) ;
#3503=CARTESIAN_POINT ( 'NONE',  ( 115.7610046295247912, -4.863998795839590272, -7.631215200338315796 ) ) ;
#3504=CARTESIAN_POINT ( 'NONE',  ( 115.6915515045247531, -6.936859964151197211, -18.39754474579287447 ) ) ;
#3507=LINE ( 'NONE', #91, #10477 ) ;
#3508=ORIENTED_EDGE ( 'NONE', *, *, #40922, .T. ) ;
#3512=CARTESIAN_POINT ( 'NONE',  ( 84.51109360120413783, -29.99489077589588959, -12.39321520033831625 ) ) ;
#3517=CARTESIAN_POINT ( 'NONE',  ( 74.19189222814998175, -41.76310523276723785, -20.39321520033831447 ) ) ;
#3518=CARTESIAN_POINT ( 'NONE',  ( 115.3442858795247759, -0.7896495226426338832, -17.46756447353520159 ) ) ;
#3523=CARTESIAN_POINT ( 'NONE',  ( 109.9963952545248134, -9.868328341294098749, -15.46607636864997204 ) ) ;
#3524=CARTESIAN_POINT ( 'NONE',  ( 111.3854577545248503, -7.250697342233347165, -7.631215200338321125 ) ) ;
#3525=CARTESIAN_POINT ( 'NONE',  ( 109.2295012951870348, -4.728831740048331511, -18.57600240304503103 ) ) ;
#3527=CARTESIAN_POINT ( 'NONE',  ( 107.9128015045248219, -2.477300249445798297, -7.631215200338321125 ) ) ;
#3530=CARTESIAN_POINT ( 'NONE',  ( 108.7462390045248242, 0.8980012041604421569, -15.77991374673208469 ) ) ;
#3535=EDGE_CURVE ( 'NONE', #22322, #2225, #31363, .T. ) ;
#3537=ORIENTED_EDGE ( 'NONE', *, *, #23345, .F. ) ;
#3546=CARTESIAN_POINT ( 'NONE',  ( 115.0664733795247798, -8.938348069036489818, -17.46756447353520159 ) ) ;
#3547=EDGE_LOOP ( 'NONE', ( #18988, #39471, #22113, #36114 ) ) ;
#3560=CARTESIAN_POINT ( 'NONE',  ( 113.3995983795247895, -8.402594152722688392, -16.93181055722141792 ) ) ;
#3567=ORIENTED_EDGE ( 'NONE', *, *, #17796, .T. ) ;
#3570=CARTESIAN_POINT ( 'NONE',  ( 76.69189222814998175, -55.76602098829192755, -2.607500914624014232 ) ) ;
#3574=CARTESIAN_POINT ( 'NONE',  ( 105.4124890045248293, -9.868328341294098749, -11.32035403202665869 ) ) ;
#3575=CARTESIAN_POINT ( 'NONE',  ( 113.0523327545247838, -2.477300249445798297, -19.15521520033831138 ) ) ;
#3578=CARTESIAN_POINT ( 'NONE',  ( 109.2294421680114596, -0.2361213814094521024, -10.76286691213928748 ) ) ;
#3579=CARTESIAN_POINT ( 'NONE',  ( 107.1488171295247867, 0.1403307496149613920, -13.39321520033831447 ) ) ;
#3580=B_SPLINE_CURVE_WITH_KNOTS ( 'NONE', 3,
 ( #38872, #32031, #14718, #28629, #32257, #1025, #14943 ),
 .UNSPECIFIED., .F., .F.,
 ( 4, 3, 4 ),
 ( 0.0003705783391767355139, 0.0004952974148303549741, 0.0009534114850261810395 ),
 .UNSPECIFIED. ) ;
#3582=CARTESIAN_POINT ( 'NONE',  ( 109.2292940338004286, -1.048241503082447457, -16.67292528126275641 ) ) ;
#3585=CARTESIAN_POINT ( 'NONE',  ( 109.1629577545248395, -7.250697342233347165, -7.631215200338321125 ) ) ;
#3587=ADVANCED_FACE ( 'NONE', ( #25434 ), #22003, .F. ) ;
#3596=CARTESIAN_POINT ( 'NONE',  ( 108.3295202545248657, 0.1403307496149616695, -11.32035403202665336 ) ) ;
#3598=DIRECTION ( 'NONE',  ( 0.000000000000000000, -1.000000000000000000, 0.000000000000000000 ) ) ;
#3603=VERTEX_POINT ( 'NONE', #35443 ) ;
#3604=CARTESIAN_POINT ( 'NONE',  ( 113.8857702545248003, -10.62599879583958717, -15.77991374673208469 ) ) ;
#3607=CARTESIAN_POINT ( 'NONE',  ( 116.0861162244890892, -0.02276961308034231024, -12.14321520033833934 ) ) ;
#3622=CARTESIAN_POINT ( 'NONE',  ( 107.9128015045248219, -2.477300249445798297, -7.631215200338321125 ) ) ;
#3626=FACE_OUTER_BOUND ( 'NONE', #182, .T. ) ;
#3629=VECTOR ( 'NONE', #43163, 1000.000000000000000 ) ;
#3630=CARTESIAN_POINT ( 'NONE',  ( 116.0286950891469786, 2.331313199634366118, -14.64321520033831447 ) ) ;
#3635=CARTESIAN_POINT ( 'NONE',  ( 112.1494421295248003, -9.868328341294093420, -13.39321520033831447 ) ) ;
#3642=CARTESIAN_POINT ( 'NONE',  ( 61.69189222814998175, -66.48243304680813992, -42.55772070205831170 ) ) ;
#3643=CARTESIAN_POINT ( 'NONE',  ( 68.68839935636917460, -25.95913848132418522, -5.893215200338315363 ) ) ;
#3646=EDGE_CURVE ( 'NONE', #44662, #3847, #3580, .T. ) ;
#3656=CARTESIAN_POINT ( 'NONE',  ( 106.0375671295248310, -10.62599879583958540, -13.39321520033831447 ) ) ;
#3673=CARTESIAN_POINT ( 'NONE',  ( 71.36400868967236022, -24.42718413923373788, -4.893215200338314474 ) ) ;
#3678=CARTESIAN_POINT ( 'NONE',  ( 116.0388171295248014, 0.1403307496149613920, -13.39321520033831447 ) ) ;
#3679=CARTESIAN_POINT ( 'NONE',  ( 109.3713171295247832, 0.1403307496149613920, -13.39321520033831447 ) ) ;
#3680=CARTESIAN_POINT ( 'NONE',  ( 112.5661608795247872, -1.325403438956436419, -16.93181055722141792 ) ) ;
#3685=CARTESIAN_POINT ( 'NONE',  ( 111.0381921295247878, 0.8980012041604618078, -13.39321520033831447 ) ) ;
#3686=CARTESIAN_POINT ( 'NONE',  ( 66.82415148905926117, -40.21211973637273474, -4.893215200338314474 ) ) ;
#3691=CARTESIAN_POINT ( 'NONE',  ( 114.7192077545248594, -7.250697342233347165, -7.631215200338321125 ) ) ;
#3692=CARTESIAN_POINT ( 'NONE',  ( 115.0664733795247798, -1.325403438956436419, -9.854619843455211026 ) ) ;
#3693=VERTEX_POINT ( 'NONE', #40469 ) ;
#3699=CARTESIAN_POINT ( 'NONE',  ( 115.0664733795247798, -8.938348069036489818, -17.46756447353520159 ) ) ;
#3700=CARTESIAN_POINT ( 'NONE',  ( 105.7597546295248350, -4.863998795839590272, -18.39754474579285315 ) ) ;
#3708=ORIENTED_EDGE ( 'NONE', *, *, #34863, .F. ) ;
#3710=CARTESIAN_POINT ( 'NONE',  ( 112.2883483795247770, -8.402594152722688392, -16.93181055722141792 ) ) ;
#3720=CARTESIAN_POINT ( 'NONE',  ( 106.3153796295248412, -4.863998795839590272, -8.388885654883775800 ) ) ;
#3721=CARTESIAN_POINT ( 'NONE',  ( 117.2014317992446024, -11.08072105495146076, -21.84774360349757316 ) ) ;
#3734=CARTESIAN_POINT ( 'NONE',  ( 109.4154010812577837, -0.01829820670803256055, -12.14321520033831625 ) ) ;
#3735=CARTESIAN_POINT ( 'NONE',  ( 113.2606921295247702, 0.8980012041604618078, -13.39321520033831447 ) ) ;
#3740=CARTESIAN_POINT ( 'NONE',  ( 112.0799890045248475, -9.868328341294098749, -11.32035403202665869 ) ) ;
#3741=CARTESIAN_POINT ( 'NONE',  ( 111.7327233795247849, -8.938348069036441856, -17.46756447353520869 ) ) ;
#3742=CARTESIAN_POINT ( 'NONE',  ( 109.2294312348150527, -3.835661836656289569, -18.43199761928219971 ) ) ;
#3745=EDGE_CURVE ( 'NONE', #6998, #44941, #30200, .T. ) ;
#3746=CARTESIAN_POINT ( 'NONE',  ( 106.2459265045248173, -7.250697342233347165, -19.15521520033831138 ) ) ;
#3747=CARTESIAN_POINT ( 'NONE',  ( 114.5108483795247878, -8.402594152722688392, -16.93181055722141792 ) ) ;
#3748=CARTESIAN_POINT ( 'NONE',  ( 111.5938171295247940, -10.62599879583958540, -13.39321520033831447 ) ) ;
#3757=DIRECTION ( 'NONE',  ( 0.000000000000000000, 1.000000000000000000, 0.000000000000000000 ) ) ;
#3764=CARTESIAN_POINT ( 'NONE',  ( 107.9822546295247889, -4.863998795839590272, -7.631215200338315796 ) ) ;
#3766=CARTESIAN_POINT ( 'NONE',  ( 143.3676850761856940, -50.16718729050181480, 3.106784799661685526 ) ) ;
#3767=CARTESIAN_POINT ( 'NONE',  ( 116.9417077545247992, -2.791137627527939813, -18.39754474579286025 ) ) ;
#3769=CARTESIAN_POINT ( 'NONE',  ( 86.50830818076254047, -21.65036132658698520, -20.89321520033831447 ) ) ;
#3773=CARTESIAN_POINT ( 'NONE',  ( 114.9970202545248412, 0.1403307496149616695, -11.32035403202665336 ) ) ;
#3783=CARTESIAN_POINT ( 'NONE',  ( 115.8304577545247582, -2.791137627527939813, -18.39754474579286025 ) ) ;
#3786=CARTESIAN_POINT ( 'NONE',  ( 85.35287308025479547, -28.80162431559100611, -9.543249340220466337 ) ) ;
#3787=CARTESIAN_POINT ( 'NONE',  ( 111.3854577545248645, -7.250697342233347165, -7.631215200338321125 ) ) ;
#3790=CARTESIAN_POINT ( 'NONE',  ( 115.5334957829843887, 0.6362173239733635022, -14.64321520033831447 ) ) ;
#3793=CARTESIAN_POINT ( 'NONE',  ( 108.6767858795247861, -8.402594152722688392, -9.854619843455216355 ) ) ;
#3794=CARTESIAN_POINT ( 'NONE',  ( 116.5840207075926145, 2.158964875678295314, -20.60257148143831074 ) ) ;
#3797=CARTESIAN_POINT ( 'NONE',  ( 111.9410827545248708, -2.477300249445798297, -19.15521520033831138 ) ) ;
#3800=LINE ( 'NONE', #393, #22498 ) ;
#3801=VECTOR ( 'NONE', #33295, 1000.000000000000000 ) ;
#3811=CARTESIAN_POINT ( 'NONE',  ( 109.0935046295247872, -4.863998795839590272, -18.39754474579285315 ) ) ;
#3820=CARTESIAN_POINT ( 'NONE',  ( 115.4137390045248566, 0.8980012041604421569, -15.77991374673208469 ) ) ;
#3824=ADVANCED_FACE ( 'NONE', ( #39562 ), #15612, .F. ) ;
#3837=CARTESIAN_POINT ( 'NONE',  ( 87.44708369096657918, -21.99489077589588604, -6.893215200338315363 ) ) ;
#3841=CARTESIAN_POINT ( 'NONE',  ( 105.7597546295248350, -4.863998795839590272, -7.631215200338315796 ) ) ;
#3844=FACE_OUTER_BOUND ( 'NONE', #11522, .T. ) ;
#3847=VERTEX_POINT ( 'NONE', #37482 ) ;
#3850=CYLINDRICAL_SURFACE ( 'NONE', #2371, 20.00000000000000355 ) ;
#3853=CARTESIAN_POINT ( 'NONE',  ( 114.2330358795247776, -8.402594152722688392, -9.854619843455216355 ) ) ;
#3865=FACE_OUTER_BOUND ( 'NONE', #18802, .T. ) ;
#3877=CARTESIAN_POINT ( 'NONE',  ( 106.3848327545248651, -2.477300249445798297, -19.15521520033831138 ) ) ;
#3889=CARTESIAN_POINT ( 'NONE',  ( 78.69189222814998175, -46.76310523276723785, -4.893215200338314474 ) ) ;
#3899=CARTESIAN_POINT ( 'NONE',  ( 115.6915515045247531, -6.936859964151250502, -18.39754474579286025 ) ) ;
#3901=CARTESIAN_POINT ( 'NONE',  ( 108.7462390045248242, -9.868328341294098749, -11.32035403202665869 ) ) ;
#3902=CARTESIAN_POINT ( 'NONE',  ( 113.1217858795247935, -8.402594152722688392, -9.854619843455216355 ) ) ;
#3905=ORIENTED_EDGE ( 'NONE', *, *, #20391, .T. ) ;
#3907=CARTESIAN_POINT ( 'NONE',  ( 113.1912390045248031, 0.8980012041604421569, -15.77991374673208469 ) ) ;
#3913=CARTESIAN_POINT ( 'NONE',  ( 115.8304577545247582, -7.250697342233347165, -7.631215200338321125 ) ) ;
#3914=CARTESIAN_POINT ( 'NONE',  ( 114.3719421295247827, -9.868328341294093420, -13.39321520033831447 ) ) ;
#3917=DIRECTION ( 'NONE',  ( 0.000000000000000000, 0.000000000000000000, -1.000000000000000000 ) ) ;
#3920=CARTESIAN_POINT ( 'NONE',  ( 114.7886608795247696, -8.938348069036489818, -9.318865927141430916 ) ) ;
#3921=CARTESIAN_POINT ( 'NONE',  ( 106.3848327545248651, -6.936859964151250502, -8.388885654883777576 ) ) ;
#3925=ORIENTED_EDGE ( 'NONE', *, *, #21962, .F. ) ;
#3934=CARTESIAN_POINT ( 'NONE',  ( 109.9269421295247753, -9.868328341294093420, -13.39321520033831447 ) ) ;
#3942=CARTESIAN_POINT ( 'NONE',  ( 116.4555358795247884, -0.7896495226426338832, -17.46756447353520159 ) ) ;
#3945=EDGE_CURVE ( 'NONE', #40078, #35613, #9915, .T. ) ;
#3952=CARTESIAN_POINT ( 'NONE',  ( 86.29547825138352835, -26.51858395224443754, -8.393215200338314474 ) ) ;
#3953=CARTESIAN_POINT ( 'NONE',  ( 115.9693640045247776, -10.62599879583958717, -11.00651665394454604 ) ) ;
#3957=CARTESIAN_POINT ( 'NONE',  ( 109.7003860982116805, 0.3867979994853637526, -12.14321520033828072 ) ) ;
#3958=CARTESIAN_POINT ( 'NONE',  ( 109.5796765045248122, -7.250697342233347165, -19.15521520033831138 ) ) ;
#3963=CARTESIAN_POINT ( 'NONE',  ( 111.8716296295247901, -4.863998795839638234, -8.388885654883775800 ) ) ;
#3964=CARTESIAN_POINT ( 'NONE',  ( 111.3160046295247838, -4.863998795839590272, -18.39754474579285315 ) ) ;
#3967=CARTESIAN_POINT ( 'NONE',  ( 109.2294391953206798, -4.004300405888451486, -18.47138478117985372 ) ) ;
#3970=FACE_OUTER_BOUND ( 'NONE', #24951, .T. ) ;
#3971=CARTESIAN_POINT ( 'NONE',  ( 108.9545983795247821, -0.7896495226426338832, -9.318865927141430916 ) ) ;
#3987=CARTESIAN_POINT ( 'NONE',  ( 111.2465515045248168, -2.477300249445798297, -7.631215200338321125 ) ) ;
#3991=CARTESIAN_POINT ( 'NONE',  ( 116.5249890045247980, -9.868328341294098749, -11.32035403202665869 ) ) ;
#3994=DIRECTION ( 'NONE',  ( -0.3445294493088599252, -0.9387755102040817867, 0.000000000000000000 ) ) ;
#3998=CARTESIAN_POINT ( 'NONE',  ( 116.4555358795247884, -8.402594152722688392, -9.854619843455216355 ) ) ;
#4007=ORIENTED_EDGE ( 'NONE', *, *, #45112, .T. ) ;
#4010=CARTESIAN_POINT ( 'NONE',  ( 113.7468640045248236, 0.1403307496149616695, -15.46607636864997204 ) ) ;
#4013=CARTESIAN_POINT ( 'NONE',  ( 85.18868397526492231, -29.19971465527826737, -9.984222205337539791 ) ) ;
#4014=CARTESIAN_POINT ( 'NONE',  ( 111.2465515045248168, -2.477300249445798297, -7.631215200338321125 ) ) ;
#4018=CARTESIAN_POINT ( 'NONE',  ( 115.6217004682427785, 0.5115630086001619059, -14.64321520033831447 ) ) ;
#4021=CARTESIAN_POINT ( 'NONE',  ( 110.6909265045248247, -2.791137627527939813, -8.388885654883777576 ) ) ;
#4022=CARTESIAN_POINT ( 'NONE',  ( 116.8216831185638398, 1.980589080847753092, -20.92910018805106276 ) ) ;
#4025=CARTESIAN_POINT ( 'NONE',  ( 111.6632702545248605, -10.62599879583958717, -15.77991374673208469 ) ) ;
#4035=CARTESIAN_POINT ( 'NONE',  ( 113.8857702545248003, -10.62599879583958717, -15.77991374673208469 ) ) ;
#4040=( BOUNDED_CURVE ( )  B_SPLINE_CURVE ( 3, ( #38249, #20941, #10681, #14990 ),
 .UNSPECIFIED., .F., .T. ) 
 B_SPLINE_CURVE_WITH_KNOTS ( ( 4, 4 ),
 ( 4.712388980384689674, 7.853981633974479237 ),
 .UNSPECIFIED. ) 
 CURVE ( )  GEOMETRIC_REPRESENTATION_ITEM ( )  RATIONAL_B_SPLINE_CURVE ( ( 1.000000000000000000, 0.3333333333333335369, 0.3333333333333335369, 1.000000000000000000 ) ) 
 REPRESENTATION_ITEM ( '' )  );
#4045=CARTESIAN_POINT ( 'NONE',  ( 115.0664733795247798, -8.938348069036489818, -17.46756447353520159 ) ) ;
#4061=CARTESIAN_POINT ( 'NONE',  ( 115.6915515045247531, -6.936859964151250502, -18.39754474579286025 ) ) ;
#4073=CARTESIAN_POINT ( 'NONE',  ( 112.4272546295247821, -4.863998795839590272, -18.39754474579285315 ) ) ;
#4075=ORIENTED_EDGE ( 'NONE', *, *, #42977, .F. ) ;
#4084=CARTESIAN_POINT ( 'NONE',  ( 110.3455291257774888, 0.2334052082820642360, -12.14321520033831625 ) ) ;
#4089=CARTESIAN_POINT ( 'NONE',  ( 115.6915515045247531, -6.936859964151250502, -18.39754474579286025 ) ) ;
#4096=CARTESIAN_POINT ( 'NONE',  ( 111.5497331777918788, -0.01829820670803256055, -14.64321520033831447 ) ) ;
#4098=ORIENTED_EDGE ( 'NONE', *, *, #11680, .T. ) ;
#4100=AXIS2_PLACEMENT_3D ( 'NONE', #5709, #43809, #32628 ) ;
#4101=CARTESIAN_POINT ( 'NONE',  ( 117.2294421295248270, 0.5103437856549055684, -4.893215200338311810 ) ) ;
#4116=ORIENTED_EDGE ( 'NONE', *, *, #27250, .T. ) ;
#4122=CARTESIAN_POINT ( 'NONE',  ( 112.4272546295247821, -4.863998795839590272, -18.39754474579285315 ) ) ;
#4123=CARTESIAN_POINT ( 'NONE',  ( 108.1906140045248037, 0.1403307496149616695, -15.46607636864997204 ) ) ;
#4124=CARTESIAN_POINT ( 'NONE',  ( 114.2330358795247776, -8.402594152722688392, -9.854619843455216355 ) ) ;
#4127=( BOUNDED_CURVE ( )  B_SPLINE_CURVE ( 2, ( #4096, #32587, #25322, #42424, #35553, #1575, #36234, #39894, #1357, #15269, #43090, #18913, #29403, #11628, #31916, #25764, #28964 ),
 .UNSPECIFIED., .F., .T. ) 
 B_SPLINE_CURVE_WITH_KNOTS ( ( 3, 2, 2, 2, 2, 2, 2, 2, 3 ),
 ( 0.4040431156034944848, 0.4124999999999999778, 0.4249999999999999889, 0.4375000000000000000, 0.4500000000000000111, 0.4625000000000000222, 0.4749999999999999778, 0.4874999999999999889, 0.4959568843965059814 ),
 .UNSPECIFIED. ) 
 CURVE ( )  GEOMETRIC_REPRESENTATION_ITEM ( )  RATIONAL_B_SPLINE_CURVE ( ( 0.9666851417651740608, 0.9485006404992000206, 1.000000000000000000, 0.9238795325112869605, 1.000000000000000000, 0.9238795325112869605, 1.000000000000000000, 0.9238795325112869605, 1.000000000000000000, 0.9238795325112869605, 1.000000000000000000, 0.9238795325112869605, 1.000000000000000000, 0.9238795325112869605, 1.000000000000000000, 0.9485006404991980222, 0.9666851417651760592 ) ) 
 REPRESENTATION_ITEM ( '' )  );
#4128=ORIENTED_EDGE ( 'NONE', *, *, #1924, .T. ) ;
#4130=CARTESIAN_POINT ( 'NONE',  ( 107.8433483795247838, -0.7896495226426338832, -9.318865927141430916 ) ) ;
#4137=CARTESIAN_POINT ( 'NONE',  ( 113.7468640045248236, -10.62599879583958717, -11.00651665394454604 ) ) ;
#4138=CARTESIAN_POINT ( 'NONE',  ( 113.6079577545248043, -2.791137627527939813, -18.39754474579286025 ) ) ;
#4139=ORIENTED_EDGE ( 'NONE', *, *, #44843, .F. ) ;
#4140=CARTESIAN_POINT ( 'NONE',  ( 116.2659068881580708, -12.01880880694303855, -6.893215200338315363 ) ) ;
#4158=CARTESIAN_POINT ( 'NONE',  ( 117.2294421295247844, -4.863998795839590272, -19.02821520033831604 ) ) ;
#4160=CARTESIAN_POINT ( 'NONE',  ( 111.7327233795247849, -1.325403438956436419, -9.854619843455211026 ) ) ;
#4170=CARTESIAN_POINT ( 'NONE',  ( 111.6632702545248605, -10.62599879583958717, -15.77991374673208469 ) ) ;
#4176=ORIENTED_EDGE ( 'NONE', *, *, #4713, .F. ) ;
#4179=CARTESIAN_POINT ( 'NONE',  ( 85.67997340455728761, -28.00936669380753585, -8.898069645441740505 ) ) ;
#4185=CARTESIAN_POINT ( 'NONE',  ( 111.4549108795247747, -8.938348069036489818, -9.318865927141430916 ) ) ;
#4191=CARTESIAN_POINT ( 'NONE',  ( 110.6909265045248247, -2.791137627527939813, -8.388885654883777576 ) ) ;
#4193=EDGE_LOOP ( 'NONE', ( #148, #21367, #47, #26700 ) ) ;
#4195=CARTESIAN_POINT ( 'NONE',  ( 109.2296420770869645, -6.046829405984460948, -18.50501756593391178 ) ) ;
#4199=CARTESIAN_POINT ( 'NONE',  ( 110.9687390045248350, 0.8980012041604421569, -15.77991374673208469 ) ) ;
#4212=ORIENTED_EDGE ( 'NONE', *, *, #41209, .F. ) ;
#4217=CARTESIAN_POINT ( 'NONE',  ( 109.0240515045248202, -2.477300249445798297, -7.631215200338321125 ) ) ;
#4218=FACE_OUTER_BOUND ( 'NONE', #37197, .T. ) ;
#4220=CARTESIAN_POINT ( 'NONE',  ( 115.5526452545247622, -9.868328341294098749, -15.46607636864997204 ) ) ;
#4226=CARTESIAN_POINT ( 'NONE',  ( 113.9552233795247815, -1.325403438956436419, -9.854619843455211026 ) ) ;
#4238=CARTESIAN_POINT ( 'NONE',  ( 112.4967077545247633, -2.791137627527939813, -18.39754474579286025 ) ) ;
#4243=CARTESIAN_POINT ( 'NONE',  ( 110.9687390045248350, 0.8980012041604421569, -15.77991374673208469 ) ) ;
#4246=CARTESIAN_POINT ( 'NONE',  ( 116.1777233795247781, -1.325403438956436419, -9.854619843455244776 ) ) ;
#4247=CARTESIAN_POINT ( 'NONE',  ( 109.2293038749584753, -2.355862545069713043, -8.536032044935492280 ) ) ;
#4249=CARTESIAN_POINT ( 'NONE',  ( 116.0388171295248014, -10.62599879583958540, -13.39321520033831447 ) ) ;
#4253=CARTESIAN_POINT ( 'NONE',  ( 110.8992858795247827, -0.7896495226426338832, -17.46756447353520159 ) ) ;
#4263=CARTESIAN_POINT ( 'NONE',  ( 112.1494421295248003, 0.8980012041604618078, -13.39321520033831447 ) ) ;
#4271=ORIENTED_EDGE ( 'NONE', *, *, #16277, .T. ) ;
#4277=CARTESIAN_POINT ( 'NONE',  ( 66.38809756183205479, -36.79083284667497367, -4.893215200338314474 ) ) ;
#4291=CARTESIAN_POINT ( 'NONE',  ( 112.7745202545247878, 0.1403307496149616695, -11.32035403202665336 ) ) ;
#4293=CARTESIAN_POINT ( 'NONE',  ( 113.8604010812576774, -0.01829820670803256055, -12.14321520033831625 ) ) ;
#4303=CARTESIAN_POINT ( 'NONE',  ( 110.2047546295247855, -4.863998795839590272, -18.39754474579285315 ) ) ;
#4316=CARTESIAN_POINT ( 'NONE',  ( 110.0616521944299819, 0.6269505268395592079, -12.14321520033828428 ) ) ;
#4322=VERTEX_POINT ( 'NONE', #38822 ) ;
#4323=DIRECTION ( 'NONE',  ( 0.000000000000000000, -1.000000000000000000, 1.195183497228115774E-16 ) ) ;
#4325=CARTESIAN_POINT ( 'NONE',  ( 66.69189222814998175, -41.76310523276723785, -24.89321520033831447 ) ) ;
#4330=DIRECTION ( 'NONE',  ( 0.000000000000000000, 0.000000000000000000, -1.000000000000000000 ) ) ;
#4332=CARTESIAN_POINT ( 'NONE',  ( 79.45722259695331502, 5.067161157875061939, -20.39651227415351542 ) ) ;
#4335=LINE ( 'NONE', #35791, #5117 ) ;
#4336=CARTESIAN_POINT ( 'NONE',  ( 109.3272331777918822, -0.01829820670803256055, -14.64321520033831447 ) ) ;
#4338=VECTOR ( 'NONE', #22507, 1000.000000000000000 ) ;
#4341=CARTESIAN_POINT ( 'NONE',  ( 116.6216037019470235, -9.736060787689369889, -14.64821204404636745 ) ) ;
#4345=ORIENTED_EDGE ( 'NONE', *, *, #20682, .T. ) ;
#4349=CARTESIAN_POINT ( 'NONE',  ( 115.3442858795247759, -8.402594152722688392, -9.854619843455216355 ) ) ;
#4350=CARTESIAN_POINT ( 'NONE',  ( 112.4967077545247633, -2.791137627527939813, -18.39754474579286025 ) ) ;
#4355=CARTESIAN_POINT ( 'NONE',  ( 105.8292077545248446, -7.250697342233347165, -7.631215200338321125 ) ) ;
#4356=DIRECTION ( 'NONE',  ( 0.000000000000000000, 0.000000000000000000, -1.000000000000000000 ) ) ;
#4359=CARTESIAN_POINT ( 'NONE',  ( 79.36790013323479798, 5.032986779684683221, -6.252821205110531189 ) ) ;
#4361=CARTESIAN_POINT ( 'NONE',  ( 112.8439733795247832, -8.938348069036489818, -17.46756447353520159 ) ) ;
#4362=CARTESIAN_POINT ( 'NONE',  ( 110.4825671295247815, 0.1403307496149613920, -13.39321520033831447 ) ) ;
#4368=B_SPLINE_CURVE_WITH_KNOTS ( 'NONE', 3,
 ( #14121, #24611, #45147, #38954, #27597, #6842, #35064, #20749, #41945, #34627 ),
 .UNSPECIFIED., .F., .F.,
 ( 4, 3, 3, 4 ),
 ( 0.000000000000000000, 0.0002476486447138875262, 0.0004952972925464129957, 0.0009604418836934569808 ),
 .UNSPECIFIED. ) ;
#4369=CARTESIAN_POINT ( 'NONE',  ( 82.38065881859543538, -29.99489077589589314, -11.39321520033831447 ) ) ;
#4384=EDGE_CURVE ( 'NONE', #31317, #13043, #12118, .T. ) ;
#4385=CARTESIAN_POINT ( 'NONE',  ( 106.9404577545248145, -2.791137627527939813, -18.39754474579286025 ) ) ;
#4388=ORIENTED_EDGE ( 'NONE', *, *, #27284, .F. ) ;
#4393=ORIENTED_EDGE ( 'NONE', *, *, #31960, .T. ) ;
#4396=CARTESIAN_POINT ( 'NONE',  ( 110.1353015045248469, -2.477300249445798297, -7.631215200338321125 ) ) ;
#4400=EDGE_CURVE ( 'NONE', #40778, #37706, #37595, .T. ) ;
#4408=CARTESIAN_POINT ( 'NONE',  ( 112.1874712410415924, 0.7607806665037644134, -12.14321520033829493 ) ) ;
#4412=VERTEX_POINT ( 'NONE', #29464 ) ;
#4415=CARTESIAN_POINT ( 'NONE',  ( 109.8766384760652812, 0.6362173239733635022, -12.14321520033831625 ) ) ;
#4416=CARTESIAN_POINT ( 'NONE',  ( 111.5938171295247940, -10.62599879583958540, -13.39321520033831447 ) ) ;
#4421=CARTESIAN_POINT ( 'NONE',  ( 106.2459265045248173, -2.791137627527939813, -8.388885654883777576 ) ) ;
#4422=ORIENTED_EDGE ( 'NONE', *, *, #38977, .T. ) ;
#4423=CARTESIAN_POINT ( 'NONE',  ( 115.6220983795247861, -0.7896495226426338832, -9.318865927141430916 ) ) ;
#4424=CARTESIAN_POINT ( 'NONE',  ( 109.2295940650973876, -4.951169889926434031, -18.58642991963417046 ) ) ;
#4427=CARTESIAN_POINT ( 'NONE',  ( 115.9693640045247776, 0.1403307496149616695, -15.46607636864997204 ) ) ;
#4428=CARTESIAN_POINT ( 'NONE',  ( 115.2053796295247849, -4.863998795839590272, -8.388885654883775800 ) ) ;
#4437=VECTOR ( 'NONE', #14917, 1000.000000000000000 ) ;
#4440=ORIENTED_EDGE ( 'NONE', *, *, #28510, .F. ) ;
#4445=CARTESIAN_POINT ( 'NONE',  ( 108.4684265045247997, -7.250697342233347165, -19.15521520033831138 ) ) ;
#4448=DIRECTION ( 'NONE',  ( -1.000000000000000000, 0.000000000000000000, 0.000000000000000000 ) ) ;
#4449=CARTESIAN_POINT ( 'NONE',  ( 111.7327233795247849, -1.325403438956436419, -9.854619843455211026 ) ) ;
#4451=CYLINDRICAL_SURFACE ( 'NONE', #12799, 1.000000000000000888 ) ;
#4456=CARTESIAN_POINT ( 'NONE',  ( 109.7185827545247889, -6.936859964151250502, -8.388885654883777576 ) ) ;
#4458=DIRECTION ( 'NONE',  ( 0.000000000000000000, 0.000000000000000000, 1.000000000000000000 ) ) ;
#4469=CARTESIAN_POINT ( 'NONE',  ( 114.7192077545248594, -2.791137627527939813, -18.39754474579286025 ) ) ;
#4472=CARTESIAN_POINT ( 'NONE',  ( 86.24197381513980076, -26.64821576645285717, -8.446815953897829132 ) ) ;
#4473=CARTESIAN_POINT ( 'NONE',  ( 107.7738952545248310, 0.8980012041604421569, -11.00651665394454071 ) ) ;
#4477=CARTESIAN_POINT ( 'NONE',  ( 109.2293033147500125, -2.564670721265329689, -8.421802055769131101 ) ) ;
#4479=CARTESIAN_POINT ( 'NONE',  ( 106.0375671295248310, 0.1403307496149613920, -13.39321520033831447 ) ) ;
#4481=CARTESIAN_POINT ( 'NONE',  ( 83.86221371915534917, -31.76296181758290516, -22.89672297930211187 ) ) ;
#4484=CARTESIAN_POINT ( 'NONE',  ( 111.8716296295247901, -4.863998795839590272, -19.15521520033831493 ) ) ;
#4494=CARTESIAN_POINT ( 'NONE',  ( 111.7327233795247849, -8.938348069036489818, -17.46756447353520159 ) ) ;
#4503=LINE ( 'NONE', #11581, #4338 ) ;
#4508=CARTESIAN_POINT ( 'NONE',  ( 77.49133083685892132, -56.78909331150907036, -1.672169083734631689 ) ) ;
#4509=CARTESIAN_POINT ( 'NONE',  ( 64.43697033563542220, -36.18204866848747514, -5.722960826912006027 ) ) ;
#4514=CARTESIAN_POINT ( 'NONE',  ( 117.1171583007951966, 0.5154571626197618217, -14.64321520033831447 ) ) ;
#4524=CARTESIAN_POINT ( 'NONE',  ( 115.2748327545248657, -6.936859964151250502, -8.388885654883777576 ) ) ;
#4534=CARTESIAN_POINT ( 'NONE',  ( 105.4819421295248247, -9.868328341294093420, -13.39321520033831447 ) ) ;
#4543=DIRECTION ( 'NONE',  ( 0.000000000000000000, -1.000000000000000000, 0.000000000000000000 ) ) ;
#4549=PLANE ( 'NONE',  #25480 ) ;
#4554=ORIENTED_EDGE ( 'NONE', *, *, #5509, .T. ) ;
#4562=VECTOR ( 'NONE', #10190, 1000.000000000000000 ) ;
#4567=CARTESIAN_POINT ( 'NONE',  ( 116.6973107111196271, -7.645574652714573816, -17.67460368773177493 ) ) ;
#4572=CARTESIAN_POINT ( 'NONE',  ( 116.3860827545247787, -2.477300249445798297, -19.15521520033831138 ) ) ;
#4573=CARTESIAN_POINT ( 'NONE',  ( 115.4137390045248566, -9.868328341294098749, -11.32035403202665869 ) ) ;
#4574=CARTESIAN_POINT ( 'NONE',  ( 115.4831921295247952, -9.868328341294093420, -13.39321520033831447 ) ) ;
#4579=CARTESIAN_POINT ( 'NONE',  ( 106.4542858795248179, -0.7896495226426338832, -17.46756447353520159 ) ) ;
#4582=( BOUNDED_CURVE ( )  B_SPLINE_CURVE ( 2, ( #37283, #2630, #2403, #20209, #44606, #23862, #20433, #27044, #37748, #33861, #40961, #27274, #44155, #33627, #17235, #19743, #30908 ),
 .UNSPECIFIED., .F., .F. ) 
 B_SPLINE_CURVE_WITH_KNOTS ( ( 3, 2, 2, 2, 2, 2, 2, 2, 3 ),
 ( 0.1035091206787220053, 0.1125000000000000028, 0.1250000000000000000, 0.1375000000000000111, 0.1499999999999999944, 0.1625000000000000056, 0.1749999999999999889, 0.1875000000000000000, 0.1964908793212780114 ),
 .UNSPECIFIED. ) 
 CURVE ( )  GEOMETRIC_REPRESENTATION_ITEM ( )  RATIONAL_B_SPLINE_CURVE ( ( 0.9692594319298230010, 0.9452488050343769155, 1.000000000000000000, 0.9238795325112869605, 1.000000000000000000, 0.9238795325112869605, 1.000000000000000000, 0.9238795325112869605, 1.000000000000000000, 0.9238795325112869605, 1.000000000000000000, 0.9238795325112869605, 1.000000000000000000, 0.9238795325112869605, 1.000000000000000000, 0.9452488050343769155, 0.9692594319298220018 ) ) 
 REPRESENTATION_ITEM ( '' )  );
#4586=AXIS2_PLACEMENT_3D ( 'NONE', #44356, #30212, #43666 ) ;
#4587=CARTESIAN_POINT ( 'NONE',  ( 112.5661608795247872, -8.938348069036489818, -9.318865927141430916 ) ) ;
#4588=CARTESIAN_POINT ( 'NONE',  ( 112.8439733795247832, -1.325403438956436419, -9.854619843455211026 ) ) ;
#4599=VERTEX_POINT ( 'NONE', #11696 ) ;
#4602=CARTESIAN_POINT ( 'NONE',  ( 70.19189222814998175, -83.06146523326388831, -51.81246404331846378 ) ) ;
#4604=ORIENTED_EDGE ( 'NONE', *, *, #36969, .T. ) ;
#4605=DIRECTION ( 'NONE',  ( 0.000000000000000000, 0.000000000000000000, 1.000000000000000000 ) ) ;
#4607=CARTESIAN_POINT ( 'NONE',  ( 115.6915515045247531, -2.477300249445798297, -7.631215200338321125 ) ) ;
#4615=ORIENTED_EDGE ( 'NONE', *, *, #41306, .F. ) ;
#4618=CARTESIAN_POINT ( 'NONE',  ( 61.75619731659804756, -65.97429037005174735, -43.35256525270300187 ) ) ;
#4619=CARTESIAN_POINT ( 'NONE',  ( 111.8021765045248372, -7.250697342233347165, -19.15521520033831138 ) ) ;
#4626=CARTESIAN_POINT ( 'NONE',  ( 116.4555358795247884, -0.7896495226426338832, -17.46756447353520159 ) ) ;
#4629=CARTESIAN_POINT ( 'NONE',  ( 114.9275671295247889, -10.62599879583958540, -13.39321520033831447 ) ) ;
#4634=CARTESIAN_POINT ( 'NONE',  ( 107.5655358795247736, -0.7896495226426338832, -17.46756447353520159 ) ) ;
#4639=CARTESIAN_POINT ( 'NONE',  ( 107.7738952545248310, -9.868328341294098749, -15.46607636864997204 ) ) ;
#4642=CARTESIAN_POINT ( 'NONE',  ( 109.2294689093245523, -8.931516418046212991, -16.93750435124538356 ) ) ;
#4644=CARTESIAN_POINT ( 'NONE',  ( 112.8439733795247832, -1.325403438956436419, -9.854619843455211026 ) ) ;
#4645=CARTESIAN_POINT ( 'NONE',  ( 113.6774108795247997, -1.325403438956436419, -16.93181055722141792 ) ) ;
#4663=CARTESIAN_POINT ( 'NONE',  ( 108.3295202545248657, -10.62599879583958717, -15.77991374673208469 ) ) ;
#4666=CARTESIAN_POINT ( 'NONE',  ( 113.2606921295247702, -9.868328341294093420, -13.39321520033831447 ) ) ;
#4673=CARTESIAN_POINT ( 'NONE',  ( 111.3854577545248645, -2.791137627527939813, -18.39754474579286025 ) ) ;
#4685=CARTESIAN_POINT ( 'NONE',  ( 115.4137390045248566, -9.868328341294098749, -11.32035403202665869 ) ) ;
#4691=CARTESIAN_POINT ( 'NONE',  ( 86.51169734173754478, -25.99489077589583630, -8.393215200338314474 ) ) ;
#4692=CARTESIAN_POINT ( 'NONE',  ( 106.3153796295248412, -4.863998795839590272, -19.15521520033831493 ) ) ;
#4698=CARTESIAN_POINT ( 'NONE',  ( 114.9970202545248412, -10.62599879583958717, -15.77991374673208469 ) ) ;
#4700=CARTESIAN_POINT ( 'NONE',  ( 116.9314277858571955, 1.864452410925628856, -21.08963232287759837 ) ) ;
#4701=CARTESIAN_POINT ( 'NONE',  ( 116.2471765045247594, -7.250697342233347165, -19.15521520033831138 ) ) ;
#4704=CARTESIAN_POINT ( 'NONE',  ( 107.7044421295247929, 0.8980012041604618078, -13.39321520033831447 ) ) ;
#4706=LINE ( 'NONE', #32516, #24999 ) ;
#4708=CARTESIAN_POINT ( 'NONE',  ( 116.2503515045248719, -2.792930983974093007, -8.393215200338321580 ) ) ;
#4713=EDGE_CURVE ( 'NONE', #16653, #3445, #36003, .T. ) ;
#4719=CARTESIAN_POINT ( 'NONE',  ( 114.8581140045248361, -10.62599879583958717, -11.00651665394454604 ) ) ;
#4722=LINE ( 'NONE', #24802, #27924 ) ;
#4727=LINE ( 'NONE', #32753, #29842 ) ;
#4746=CARTESIAN_POINT ( 'NONE',  ( 112.9134265045247645, -2.791137627527939813, -8.388885654883777576 ) ) ;
#4747=CARTESIAN_POINT ( 'NONE',  ( 82.55633208288642777, -31.76683555124534664, -22.98062779949958312 ) ) ;
#4749=CARTESIAN_POINT ( 'NONE',  ( 86.04230958663552542, -25.82262605124138943, -7.893215200338315363 ) ) ;
#4757=CARTESIAN_POINT ( 'NONE',  ( 108.5378796295247810, -4.863998795839590272, -8.388885654883775800 ) ) ;
#4758=ORIENTED_EDGE ( 'NONE', *, *, #41547, .F. ) ;
#4760=DIRECTION ( 'NONE',  ( 1.000000000000000000, 0.000000000000000000, 0.000000000000000000 ) ) ;
#4765=CARTESIAN_POINT ( 'NONE',  ( 63.10250807381770244, -31.76310523276723430, -22.89321520033831803 ) ) ;
#4766=DIRECTION ( 'NONE',  ( 0.000000000000000000, 0.000000000000000000, -1.000000000000000000 ) ) ;
#4769=AXIS2_PLACEMENT_3D ( 'NONE', #35677, #5351, #15166 ) ;
#4775=CARTESIAN_POINT ( 'NONE',  ( 73.37572422742091760, -11.86958442233774313, -21.89321520033831447 ) ) ;
#4784=DIRECTION ( 'NONE',  ( 4.844864995884620227E-15, -6.938893903907220489E-15, 1.000000000000000000 ) ) ;
#4791=CARTESIAN_POINT ( 'NONE',  ( 116.7009281483881296, -7.496663152239960048, -17.77315041048467847 ) ) ;
#4799=CARTESIAN_POINT ( 'NONE',  ( 110.8298327545248299, -6.936859964151250502, -8.388885654883777576 ) ) ;
#4800=CARTESIAN_POINT ( 'NONE',  ( 109.0240515045248202, -6.936859964151250502, -18.39754474579286025 ) ) ;
#4805=CARTESIAN_POINT ( 'NONE',  ( 109.0240515045248202, -2.477300249445798297, -7.631215200338321125 ) ) ;
#4809=FACE_BOUND ( 'NONE', #14857, .T. ) ;
#4811=CARTESIAN_POINT ( 'NONE',  ( 109.9269421295247753, 0.8980012041604618078, -13.39321520033831447 ) ) ;
#4812=CARTESIAN_POINT ( 'NONE',  ( 110.2742077545248094, -2.791137627527939813, -18.39754474579286025 ) ) ;
#4824=VECTOR ( 'NONE', #24022, 1000.000000000000114 ) ;
#4825=CARTESIAN_POINT ( 'NONE',  ( 113.7248434012278722, 0.04929351793716424401, -14.64321520033828605 ) ) ;
#4830=CARTESIAN_POINT ( 'NONE',  ( 108.3989733795247759, -1.325403438956436419, -9.854619843455211026 ) ) ;
#4841=EDGE_LOOP ( 'NONE', ( #27472, #24 ) ) ;
#4843=CARTESIAN_POINT ( 'NONE',  ( 61.69189222814999596, -66.25068106556746272, -42.68838236875360792 ) ) ;
#4844=CARTESIAN_POINT ( 'NONE',  ( 109.3713171295247832, -10.62599879583958540, -13.39321520033831447 ) ) ;
#4861=CARTESIAN_POINT ( 'NONE',  ( 63.16139403827867937, -37.76446527787062735, -4.964738833969116527 ) ) ;
#4862=CARTESIAN_POINT ( 'NONE',  ( 107.9822546295247889, -4.863998795839590272, -7.631215200338315796 ) ) ;
#4866=CARTESIAN_POINT ( 'NONE',  ( 117.2294421295247844, -10.76310523276723785, -5.182735500338556456 ) ) ;
#4869=EDGE_LOOP ( 'NONE', ( #19071, #18537, #13713, #22784 ) ) ;
#4871=CARTESIAN_POINT ( 'NONE',  ( 109.2294420847119625, -10.34908636181675412, -14.14639072714987833 ) ) ;
#4873=CARTESIAN_POINT ( 'NONE',  ( 110.6214733795247867, -1.325403438956436419, -9.854619843455211026 ) ) ;
#4874=CARTESIAN_POINT ( 'NONE',  ( 107.0793640045248196, -10.62599879583958717, -11.00651665394454604 ) ) ;
#4891=CARTESIAN_POINT ( 'NONE',  ( 113.8163171295247764, 0.1403307496149613920, -13.39321520033831447 ) ) ;
#4898=CARTESIAN_POINT ( 'NONE',  ( 111.1076452545248259, -9.868328341294098749, -15.46607636864997204 ) ) ;
#4906=VERTEX_POINT ( 'NONE', #21652 ) ;
#4909=CARTESIAN_POINT ( 'NONE',  ( 108.6073327545248048, -6.936859964151250502, -8.388885654883777576 ) ) ;
#4915=CARTESIAN_POINT ( 'NONE',  ( 108.8851452545248151, 0.8980012041604421569, -11.00651665394454071 ) ) ;
#4922=CARTESIAN_POINT ( 'NONE',  ( 116.1777233795247781, -8.938348069036489818, -17.46756447353520159 ) ) ;
#4924=CARTESIAN_POINT ( 'NONE',  ( 83.60368610585459237, -32.46739910898208592, -21.41484521824674658 ) ) ;
#4927=CARTESIAN_POINT ( 'NONE',  ( 107.0793640045248196, -10.62599879583958717, -11.00651665394454604 ) ) ;
#4931=LINE ( 'NONE', #15431, #13790 ) ;
#4937=EDGE_CURVE ( 'NONE', #12500, #23757, #18234, .T. ) ;
#4938=CARTESIAN_POINT ( 'NONE',  ( 111.4549108795247747, -8.938348069036489818, -9.318865927141430916 ) ) ;
#4940=DIRECTION ( 'NONE',  ( 0.000000000000000000, 0.000000000000000000, -1.000000000000000000 ) ) ;
#4947=ORIENTED_EDGE ( 'NONE', *, *, #8308, .T. ) ;
#4952=DIRECTION ( 'NONE',  ( 1.000000000000000000, 0.000000000000000000, 0.000000000000000000 ) ) ;
#4961=ADVANCED_FACE ( 'NONE', ( #22106 ), #21206, .T. ) ;
#4965=CARTESIAN_POINT ( 'NONE',  ( 115.8999108795247821, -1.325403438956436419, -16.93181055722141792 ) ) ;
#4969=ORIENTED_EDGE ( 'NONE', *, *, #15053, .F. ) ;
#4971=CARTESIAN_POINT ( 'NONE',  ( 115.8304577545247582, -7.250697342233347165, -7.631215200338321125 ) ) ;
#4972=CARTESIAN_POINT ( 'NONE',  ( 107.2877233795247776, -1.325403438956436419, -9.854619843455211026 ) ) ;
#4973=CARTESIAN_POINT ( 'NONE',  ( 70.19189222814998175, -65.04786711941002864, -39.22192925581980916 ) ) ;
#4979=DIRECTION ( 'NONE',  ( 0.000000000000000000, 0.000000000000000000, 1.000000000000000000 ) ) ;
#4982=CARTESIAN_POINT ( 'NONE',  ( 107.0793640045248196, 0.1403307496149616695, -15.46607636864997204 ) ) ;
#4983=EDGE_LOOP ( 'NONE', ( #33509, #43895, #4007, #12481 ) ) ;
#4993=CARTESIAN_POINT ( 'NONE',  ( 116.5944421295247793, -9.868328341294093420, -13.39321520033831447 ) ) ;
#5005=CARTESIAN_POINT ( 'NONE',  ( 109.7185827545248600, -6.936859964151250502, -8.388885654883788234 ) ) ;
#5014=CARTESIAN_POINT ( 'NONE',  ( 116.6368254076533759, -9.513716847284458211, -15.34440693972388559 ) ) ;
#5020=ORIENTED_EDGE ( 'NONE', *, *, #28401, .T. ) ;
#5021=CARTESIAN_POINT ( 'NONE',  ( 114.6032811052981941, 0.4930828106259610433, -12.14321520033831625 ) ) ;
#5022=CARTESIAN_POINT ( 'NONE',  ( 114.4413952545248350, 0.8980012041604421569, -11.00651665394454071 ) ) ;
#5023=CARTESIAN_POINT ( 'NONE',  ( 111.3854577545248645, -2.791137627527939813, -18.39754474579286025 ) ) ;
#5024=CARTESIAN_POINT ( 'NONE',  ( 110.9687390045248350, -9.868328341294098749, -11.32035403202665869 ) ) ;
#5029=CARTESIAN_POINT ( 'NONE',  ( 106.5237390045248418, 0.8980012041604421569, -15.77991374673208469 ) ) ;
#5031=ADVANCED_FACE ( 'NONE', ( #15274 ), #1361, .T. ) ;
#5036=CARTESIAN_POINT ( 'NONE',  ( 111.7327233795247849, -8.938348069036489818, -17.46756447353520159 ) ) ;
#5037=CARTESIAN_POINT ( 'NONE',  ( 112.2188952545247531, -9.868328341294098749, -15.46607636864997204 ) ) ;
#5046=VERTEX_POINT ( 'NONE', #25994 ) ;
#5048=VECTOR ( 'NONE', #24433, 1000.000000000000000 ) ;
#5049=CARTESIAN_POINT ( 'NONE',  ( 113.3992004682427819, 0.5115630086001619059, -14.64321520033833401 ) ) ;
#5055=CARTESIAN_POINT ( 'NONE',  ( 107.4960827545248350, -6.936859964151250502, -8.388885654883777576 ) ) ;
#5062=ORIENTED_EDGE ( 'NONE', *, *, #42087, .T. ) ;
#5064=CARTESIAN_POINT ( 'NONE',  ( 62.64709028481676967, -64.81681335280190126, -45.78210799152465427 ) ) ;
#5065=CARTESIAN_POINT ( 'NONE',  ( 107.9822546295247889, -4.863998795839590272, -7.631215200338315796 ) ) ;
#5074=CARTESIAN_POINT ( 'NONE',  ( 113.2606921295247702, 0.8980012041604618078, -13.39321520033831447 ) ) ;
#5075=CARTESIAN_POINT ( 'NONE',  ( 115.8999108795247821, -1.325403438956436419, -16.93181055722141792 ) ) ;
#5076=CARTESIAN_POINT ( 'NONE',  ( 110.4825671295247815, -10.62599879583958540, -13.39321520033831447 ) ) ;
#5077=EDGE_CURVE ( 'NONE', #29714, #43791, #36116, .T. ) ;
#5082=CARTESIAN_POINT ( 'NONE',  ( 62.74100695445530818, -37.51187114369871978, -5.133703732075733939 ) ) ;
#5083=CARTESIAN_POINT ( 'NONE',  ( 105.8292077545248446, -7.250697342233347165, -7.631215200338321125 ) ) ;
#5087=CARTESIAN_POINT ( 'NONE',  ( 117.1518534370333811, -11.20570961459246107, -5.509241833875157646 ) ) ;
#5089=PLANE ( 'NONE',  #32480 ) ;
#5090=CARTESIAN_POINT ( 'NONE',  ( 109.2294604103198452, -10.11295469467371966, -11.27150632045694323 ) ) ;
#5092=CARTESIAN_POINT ( 'NONE',  ( 110.3436608795247764, -1.325403438956436419, -16.93181055722141792 ) ) ;
#5093=CARTESIAN_POINT ( 'NONE',  ( 115.8304577545247582, -2.791137627527939813, -18.39754474579286025 ) ) ;
#5097=CARTESIAN_POINT ( 'NONE',  ( 71.10462995142283660, -24.78225172292188816, -5.217245182122844938 ) ) ;
#5112=CARTESIAN_POINT ( 'NONE',  ( 109.0935046295247872, -4.863998795839590272, -7.631215200338315796 ) ) ;
#5114=CARTESIAN_POINT ( 'NONE',  ( 112.4967077545247633, -2.791137627527939813, -18.39754474579286025 ) ) ;
#5117=VECTOR ( 'NONE', #28975, 1000.000000000000000 ) ;
#5123=CARTESIAN_POINT ( 'NONE',  ( 116.4587108795247730, -8.399532701772287169, -9.857681294405580275 ) ) ;
#5124=CARTESIAN_POINT ( 'NONE',  ( 111.1770983795247787, -8.402594152722688392, -16.93181055722141792 ) ) ;
#5127=DIRECTION ( 'NONE',  ( 0.000000000000000000, 0.000000000000000000, -1.000000000000000000 ) ) ;
#5134=CARTESIAN_POINT ( 'NONE',  ( 110.2486464071292858, 0.2518737723193609224, -14.64321520033833934 ) ) ;
#5136=CARTESIAN_POINT ( 'NONE',  ( 108.6767858795247861, -8.402594152722688392, -9.854619843455216355 ) ) ;
#5141=CARTESIAN_POINT ( 'NONE',  ( 106.8015515045248378, -2.477300249445798297, -7.631215200338321125 ) ) ;
#5145=CARTESIAN_POINT ( 'NONE',  ( 70.19189222814998175, -86.77534409585553021, -42.52768597413476925 ) ) ;
#5146=CARTESIAN_POINT ( 'NONE',  ( 115.5526452545247622, 0.8980012041604421569, -11.00651665394454071 ) ) ;
#5148=CARTESIAN_POINT ( 'NONE',  ( 82.58377657508042091, -31.55352463209563751, -23.50578125650315542 ) ) ;
#5151=CARTESIAN_POINT ( 'NONE',  ( 69.69189222814998175, -41.76310523276723785, -23.89321520033831803 ) ) ;
#5163=CARTESIAN_POINT ( 'NONE',  ( 109.8574890045247940, 0.8980012041604421569, -15.77991374673208469 ) ) ;
#5166=CARTESIAN_POINT ( 'NONE',  ( 116.1082702545247827, -10.62599879583958717, -15.77991374673208469 ) ) ;
#5179=AXIS2_PLACEMENT_3D ( 'NONE', #39761, #43635, #1237 ) ;
#5187=CARTESIAN_POINT ( 'NONE',  ( 114.8581140045248361, 0.1403307496149616695, -15.46607636864997204 ) ) ;
#5193=CARTESIAN_POINT ( 'NONE',  ( 106.1070202545248407, 0.1403307496149616695, -11.32035403202665336 ) ) ;
#5194=CARTESIAN_POINT ( 'NONE',  ( 111.1076452545248259, -9.868328341294098749, -15.46607636864997204 ) ) ;
#5198=CARTESIAN_POINT ( 'NONE',  ( 116.3166296295247832, -4.863998795839590272, -8.388885654883775800 ) ) ;
#5205=CARTESIAN_POINT ( 'NONE',  ( 108.2600671295247992, 0.1403307496149613920, -13.39321520033831447 ) ) ;
#5206=ORIENTED_EDGE ( 'NONE', *, *, #10240, .F. ) ;
#5217=CARTESIAN_POINT ( 'NONE',  ( 113.7468640045248236, 0.1403307496149616695, -15.46607636864997204 ) ) ;
#5222=EDGE_CURVE ( 'NONE', #21278, #37706, #20878, .T. ) ;
#5231=DIRECTION ( 'NONE',  ( 0.000000000000000000, 0.000000000000000000, -1.000000000000000000 ) ) ;
#5233=CARTESIAN_POINT ( 'NONE',  ( 115.4451630180080883, 0.7607806665037644134, -14.64321520033834467 ) ) ;
#5237=CIRCLE ( 'NONE', #14693, 2.000000000000001776 ) ;
#5241=CARTESIAN_POINT ( 'NONE',  ( 116.6378439406596073, -9.495374643002518766, -15.38986610286289647 ) ) ;
#5248=CARTESIAN_POINT ( 'NONE',  ( 112.9134265045247645, -7.250697342233347165, -19.15521520033831138 ) ) ;
#5250=CARTESIAN_POINT ( 'NONE',  ( 112.1494421295248003, -9.868328341294093420, -13.39321520033831447 ) ) ;
#5251=CARTESIAN_POINT ( 'NONE',  ( 109.8574890045248509, -9.868328341294098749, -11.32035403202665869 ) ) ;
#5254=ORIENTED_EDGE ( 'NONE', *, *, #6693, .T. ) ;
#5256=DIRECTION ( 'NONE',  ( -0.9970811988817434024, 0.07634843047859724008, 0.000000000000000000 ) ) ;
#5263=CARTESIAN_POINT ( 'NONE',  ( 111.8021765045248372, -7.250697342233347165, -19.15521520033831138 ) ) ;
#5266=CARTESIAN_POINT ( 'NONE',  ( 115.4451630180080883, 0.7607806665037644134, -14.64321520033834467 ) ) ;
#5276=VECTOR ( 'NONE', #32610, 1000.000000000000114 ) ;
#5283=ADVANCED_FACE ( 'NONE', ( #22561 ), #36680, .T. ) ;
#5285=CARTESIAN_POINT ( 'NONE',  ( 115.4137390045248566, 0.8980012041604421569, -15.77991374673208469 ) ) ;
#5295=CARTESIAN_POINT ( 'NONE',  ( 62.76162801216658949, -64.72030100442231060, -45.93989290692245220 ) ) ;
#5296=CARTESIAN_POINT ( 'NONE',  ( 108.3989733795248753, -8.938348069036489818, -17.46756447353520159 ) ) ;
#5304=CIRCLE ( 'NONE', #7517, 1.500000000000001332 ) ;
#5306=CARTESIAN_POINT ( 'NONE',  ( 114.3024890045248156, 0.8980012041604421569, -15.77991374673208469 ) ) ;
#5308=CARTESIAN_POINT ( 'NONE',  ( 115.6220983795247861, -8.402594152722688392, -16.93181055722141792 ) ) ;
#5309=CARTESIAN_POINT ( 'NONE',  ( 111.3160046295247838, -4.863998795839590272, -7.631215200338315796 ) ) ;
#5314=CARTESIAN_POINT ( 'NONE',  ( 109.1629577545248395, -7.250697342233347165, -7.631215200338321125 ) ) ;
#5321=CARTESIAN_POINT ( 'NONE',  ( 109.2294421287695059, -10.35035779373698972, -14.13938231603832207 ) ) ;
#5323=CARTESIAN_POINT ( 'NONE',  ( 109.9269421295247753, -9.868328341294093420, -13.39321520033831447 ) ) ;
#5324=CARTESIAN_POINT ( 'NONE',  ( 111.5938171295247940, 0.1403307496149613920, -13.39321520033831447 ) ) ;
#5327=CARTESIAN_POINT ( 'NONE',  ( 70.88883345414545545, -25.51877778662253604, -5.473826388607204940 ) ) ;
#5348=CARTESIAN_POINT ( 'NONE',  ( 109.5796765045248122, -2.791137627527939813, -8.388885654883777576 ) ) ;
#5351=DIRECTION ( 'NONE',  ( -0.07634843047859724008, -0.9970811988817435134, 0.000000000000000000 ) ) ;
#5356=CARTESIAN_POINT ( 'NONE',  ( 116.7365233795247832, -8.399532701772287169, -16.92874910627105223 ) ) ;
#5357=CARTESIAN_POINT ( 'NONE',  ( 110.7603796295247918, -4.863998795839590272, -8.388885654883775800 ) ) ;
#5366=CARTESIAN_POINT ( 'NONE',  ( 114.4222457829843762, 0.6362173239733635022, -14.64321520033831447 ) ) ;
#5368=CARTESIAN_POINT ( 'NONE',  ( 109.0935046295247872, -4.863998795839590272, -18.39754474579285315 ) ) ;
#5373=CARTESIAN_POINT ( 'NONE',  ( 108.6073327545248048, -2.477300249445798297, -19.15521520033831138 ) ) ;
#5376=LINE ( 'NONE', #36374, #8066 ) ;
#5377=CARTESIAN_POINT ( 'NONE',  ( 112.9134265045247645, -7.250697342233347165, -19.15521520033831138 ) ) ;
#5379=CARTESIAN_POINT ( 'NONE',  ( 83.16394245587648015, -30.76310523276723785, -21.89321520033831447 ) ) ;
#5385=ORIENTED_EDGE ( 'NONE', *, *, #12196, .F. ) ;
#5393=CARTESIAN_POINT ( 'NONE',  ( 110.2047546295247855, -4.863998795839590272, -7.631215200338315796 ) ) ;
#5401=CARTESIAN_POINT ( 'NONE',  ( 113.5385046295247804, -4.863998795839541422, -18.39754474579285315 ) ) ;
#5418=CARTESIAN_POINT ( 'NONE',  ( 116.0388171295248014, 0.1403307496149613920, -13.39321520033831447 ) ) ;
#5422=CARTESIAN_POINT ( 'NONE',  ( 113.9552233795247815, -8.938348069036489818, -17.46756447353520159 ) ) ;
#5423=CARTESIAN_POINT ( 'NONE',  ( 108.3295202545248657, 0.1403307496149616695, -11.32035403202665336 ) ) ;
#5427=CARTESIAN_POINT ( 'NONE',  ( 115.1359265045248605, -2.791137627527939813, -8.388885654883777576 ) ) ;
#5432=FACE_OUTER_BOUND ( 'NONE', #37320, .T. ) ;
#5433=CARTESIAN_POINT ( 'NONE',  ( 109.3018640045248304, 0.1403307496149616695, -15.46607636864997204 ) ) ;
#5438=DIRECTION ( 'NONE',  ( 0.07634843047859418697, 0.9970811988817437355, 0.000000000000000000 ) ) ;
#5439=CARTESIAN_POINT ( 'NONE',  ( 74.69189222814998175, -41.76310523276723785, -47.71602681600972318 ) ) ;
#5441=CARTESIAN_POINT ( 'NONE',  ( 112.4272546295247821, -4.863998795839590272, -18.39754474579285315 ) ) ;
#5446=PLANE ( 'NONE',  #10384 ) ;
#5450=CARTESIAN_POINT ( 'NONE',  ( 70.19189222814998175, -61.33395589173655793, -37.73637771078311687 ) ) ;
#5452=CARTESIAN_POINT ( 'NONE',  ( 115.3484820646196880, 0.6269505268395592079, -14.64321520033831447 ) ) ;
#5465=ORIENTED_EDGE ( 'NONE', *, *, #10853, .T. ) ;
#5467=CARTESIAN_POINT ( 'NONE',  ( 109.7185827545247889, -2.477300249445798297, -19.15521520033831138 ) ) ;
#5468=CARTESIAN_POINT ( 'NONE',  ( 108.1906140045248463, 0.1403307496149616695, -15.46607636864997204 ) ) ;
#5469=CARTESIAN_POINT ( 'NONE',  ( 109.9269421295247753, -9.868328341294093420, -13.39321520033831447 ) ) ;
#5479=CARTESIAN_POINT ( 'NONE',  ( 108.3989733795248753, -8.938348069036489818, -17.46756447353520159 ) ) ;
#5498=CARTESIAN_POINT ( 'NONE',  ( 112.9134265045247645, -7.250697342233347165, -19.15521520033831138 ) ) ;
#5507=ADVANCED_FACE ( 'NONE', ( #9338 ), #30760, .T. ) ;
#5509=EDGE_CURVE ( 'NONE', #7030, #25472, #20059, .T. ) ;
#5518=VECTOR ( 'NONE', #6984, 1000.000000000000114 ) ;
#5520=EDGE_CURVE ( 'NONE', #24697, #25472, #15787, .T. ) ;
#5522=CARTESIAN_POINT ( 'NONE',  ( 112.2188952545247531, 0.8980012041604421569, -11.00651665394454071 ) ) ;
#5523=CARTESIAN_POINT ( 'NONE',  ( 114.9275671295247889, 0.1403307496149613920, -13.39321520033831447 ) ) ;
#5524=CARTESIAN_POINT ( 'NONE',  ( 113.4690515045247992, -2.477300249445798297, -7.631215200338321125 ) ) ;
#5530=CARTESIAN_POINT ( 'NONE',  ( 108.2600671295247992, -10.62599879583958540, -13.39321520033831447 ) ) ;
#5532=EDGE_CURVE ( 'NONE', #574, #1124, #41996, .T. ) ;
#5536=CARTESIAN_POINT ( 'NONE',  ( 116.9293938463531219, -11.59383920986051919, -5.945542079317219120 ) ) ;
#5537=ORIENTED_EDGE ( 'NONE', *, *, #18972, .F. ) ;
#5539=CARTESIAN_POINT ( 'NONE',  ( 109.2294825911599645, -9.927280692135916240, -15.47594509028579779 ) ) ;
#5542=CARTESIAN_POINT ( 'NONE',  ( 113.5385046295247804, -4.863998795839590272, -18.39754474579285315 ) ) ;
#5543=CARTESIAN_POINT ( 'NONE',  ( 109.1629577545248395, -2.791137627527939813, -18.39754474579286025 ) ) ;
#5545=PLANE ( 'NONE',  #17569 ) ;
#5546=CARTESIAN_POINT ( 'NONE',  ( 70.92670879693453401, -25.79851902929913976, -5.473826388607135662 ) ) ;
#5549=ORIENTED_EDGE ( 'NONE', *, *, #5598, .F. ) ;
#5561=CARTESIAN_POINT ( 'NONE',  ( 107.7044421295247929, 0.8980012041604618078, -13.39321520033831447 ) ) ;
#5564=CARTESIAN_POINT ( 'NONE',  ( 109.6491296295247793, -4.863998795839590272, -8.388885654883775800 ) ) ;
#5570=CARTESIAN_POINT ( 'NONE',  ( 116.1777233795247781, -1.325403438956436419, -9.854619843455211026 ) ) ;
#5580=CARTESIAN_POINT ( 'NONE',  ( 110.3436454522301915, 0.1168444861213632779, -14.64321520033833934 ) ) ;
#5582=CARTESIAN_POINT ( 'NONE',  ( 108.3989733795247759, -1.325403438956436419, -9.854619843455211026 ) ) ;
#5583=ADVANCED_FACE ( 'NONE', ( #19825 ), #33713, .F. ) ;
#5588=CARTESIAN_POINT ( 'NONE',  ( 113.7468640045248236, 0.1403307496149616695, -15.46607636864997204 ) ) ;
#5589=DIRECTION ( 'NONE',  ( 0.000000000000000000, 0.000000000000000000, 1.000000000000000000 ) ) ;
#5592=CARTESIAN_POINT ( 'NONE',  ( 109.2324108795247923, -8.938348069036489818, -9.318865927141430916 ) ) ;
#5594=CARTESIAN_POINT ( 'NONE',  ( 115.6915515045247531, -2.477300249445798297, -7.631215200338321125 ) ) ;
#5597=CARTESIAN_POINT ( 'NONE',  ( 108.3989733795248753, -8.938348069036489818, -17.46756447353520159 ) ) ;
#5598=EDGE_CURVE ( 'NONE', #38815, #28999, #16638, .T. ) ;
#5611=CARTESIAN_POINT ( 'NONE',  ( 110.2742077545248094, -7.250697342233347165, -7.631215200338321125 ) ) ;
#5613=CARTESIAN_POINT ( 'NONE',  ( 110.2047546295247855, -4.863998795839590272, -7.631215200338315796 ) ) ;
#5621=CARTESIAN_POINT ( 'NONE',  ( 115.3446837908067835, 0.5115630086001619059, -12.14321520033831625 ) ) ;
#5636=CARTESIAN_POINT ( 'NONE',  ( 114.0246765045248196, -2.791137627527939813, -8.388885654883777576 ) ) ;
#5640=CARTESIAN_POINT ( 'NONE',  ( 115.0664733795247798, -8.938348069036489818, -17.46756447353520159 ) ) ;
#5641=CARTESIAN_POINT ( 'NONE',  ( 108.6073327545248048, -6.936859964151250502, -8.388885654883777576 ) ) ;
#5647=CARTESIAN_POINT ( 'NONE',  ( 111.4549108795247747, -1.325403438956436419, -16.93181055722141792 ) ) ;
#5648=VERTEX_POINT ( 'NONE', #9565 ) ;
#5652=ORIENTED_EDGE ( 'NONE', *, *, #40774, .F. ) ;
#5654=LINE ( 'NONE', #33452, #2053 ) ;
#5661=DIRECTION ( 'NONE',  ( 0.000000000000000000, -0.9284778069183722282, -0.3713878862591645791 ) ) ;
#5662=CARTESIAN_POINT ( 'NONE',  ( 71.62231439647737830, -24.74987456741813929, -4.893215200338314474 ) ) ;
#5664=CARTESIAN_POINT ( 'NONE',  ( 110.9687390045248350, -9.868328341294098749, -11.32035403202665869 ) ) ;
#5667=B_SPLINE_CURVE_WITH_KNOTS ( 'NONE', 3,
 ( #3734, #20856, #17657, #39073, #11267, #38604, #3957, #7380, #4415, #14234 ),
 .UNSPECIFIED., .F., .F.,
 ( 4, 3, 3, 4 ),
 ( 0.000000000000000000, 0.0002476487219222909880, 0.0004952974148303589856, 0.0009534114850261710648 ),
 .UNSPECIFIED. ) ;
#5692=CARTESIAN_POINT ( 'NONE',  ( 111.2465515045248168, -2.477300249445798297, -7.631215200338321125 ) ) ;
#5693=CARTESIAN_POINT ( 'NONE',  ( 112.2883483795247770, -8.402594152722688392, -16.93181055722141792 ) ) ;
#5694=CARTESIAN_POINT ( 'NONE',  ( 108.1211608795247798, -1.325403438956436419, -16.93181055722141792 ) ) ;
#5697=CARTESIAN_POINT ( 'NONE',  ( 109.8368621053768948, 0.3967854368540359999, -16.28112951403850772 ) ) ;
#5704=CARTESIAN_POINT ( 'NONE',  ( 106.7320983795247855, -8.402594152722688392, -16.93181055722141792 ) ) ;
#5706=CARTESIAN_POINT ( 'NONE',  ( 107.2877233795247776, -8.938348069036489818, -17.46756447353520159 ) ) ;
#5707=DIRECTION ( 'NONE',  ( -1.387778780781445478E-15, -1.000000000000000000, 0.000000000000000000 ) ) ;
#5709=CARTESIAN_POINT ( 'NONE',  ( 61.76986277844709861, -39.32091226840162079, -4.893215200338314474 ) ) ;
#5724=CARTESIAN_POINT ( 'NONE',  ( 112.8439733795247832, -8.938348069036489818, -17.46756447353520159 ) ) ;
#5726=ORIENTED_EDGE ( 'NONE', *, *, #13331, .T. ) ;
#5727=ORIENTED_EDGE ( 'NONE', *, *, #36629, .T. ) ;
#5731=B_SPLINE_CURVE_WITH_KNOTS ( 'NONE', 3,
 ( #26165, #8615, #33210, #19324, #40069, #29584, #22513, #30258, #2203, #43949 ),
 .UNSPECIFIED., .F., .F.,
 ( 4, 3, 3, 4 ),
 ( 0.000000000000000000, 0.0002476486447138780394, 0.0004952972925464190672, 0.0009604418836934719428 ),
 .UNSPECIFIED. ) ;
#5732=DIRECTION ( 'NONE',  ( 4.295035233247849253E-16, 0.3713878862591650232, -0.9284778069183718952 ) ) ;
#5734=CARTESIAN_POINT ( 'NONE',  ( 105.9681140045248355, -10.62599879583958717, -11.00651665394454604 ) ) ;
#5743=CARTESIAN_POINT ( 'NONE',  ( 114.4413952545248350, 0.8980012041604421569, -11.00651665394454071 ) ) ;
#5744=CARTESIAN_POINT ( 'NONE',  ( 112.9134265045247645, -2.791137627527939813, -8.388885654883777576 ) ) ;
#5745=CARTESIAN_POINT ( 'NONE',  ( 113.9552233795247815, -8.938348069036489818, -17.46756447353520159 ) ) ;
#5755=CARTESIAN_POINT ( 'NONE',  ( 116.2659068881580708, -12.01880880694303855, -6.893215200338315363 ) ) ;
#5762=CARTESIAN_POINT ( 'NONE',  ( 116.1777233795247781, -8.938348069036489818, -17.46756447353520159 ) ) ;
#5763=CARTESIAN_POINT ( 'NONE',  ( 111.4549108795247747, -1.325403438956436419, -16.93181055722141792 ) ) ;
#5765=CIRCLE ( 'NONE', #37804, 20.00000000000000355 ) ;
#5766=CARTESIAN_POINT ( 'NONE',  ( 82.47484345711939113, -31.70193537549793916, -22.53651891743845681 ) ) ;
#5767=CARTESIAN_POINT ( 'NONE',  ( 68.97151291332768608, -25.95882592635068420, -5.893215200338315363 ) ) ;
#5771=EDGE_CURVE ( 'NONE', #9951, #34537, #42595, .T. ) ;
#5776=ORIENTED_EDGE ( 'NONE', *, *, #31902, .T. ) ;
#5777=CARTESIAN_POINT ( 'NONE',  ( 61.69084222814998242, 7.836001204160461420, -14.64321520033831447 ) ) ;
#5783=CARTESIAN_POINT ( 'NONE',  ( 107.0099108795247815, -8.938348069036489818, -9.318865927141430916 ) ) ;
#5788=DIRECTION ( 'NONE',  ( 1.000000000000000000, 0.000000000000000000, 0.000000000000000000 ) ) ;
#5789=CARTESIAN_POINT ( 'NONE',  ( 109.9269421295247753, -9.868328341294093420, -13.39321520033831447 ) ) ;
#5791=CYLINDRICAL_SURFACE ( 'NONE', #40144, 0.8718221387495478369 ) ;
#5799=AXIS2_PLACEMENT_3D ( 'NONE', #2855, #20428, #16786 ) ;
#5809=CARTESIAN_POINT ( 'NONE',  ( 111.2465515045248168, -6.936859964151250502, -18.39754474579286025 ) ) ;
#5813=CARTESIAN_POINT ( 'NONE',  ( 112.6356140045247827, 0.1403307496149616695, -15.46607636864997204 ) ) ;
#5818=CARTESIAN_POINT ( 'NONE',  ( 109.5102233795247884, -8.938348069036489818, -17.46756447353520159 ) ) ;
#5820=CARTESIAN_POINT ( 'NONE',  ( 115.4831921295247952, 0.8980012041604618078, -13.39321520033831447 ) ) ;
#5831=AXIS2_PLACEMENT_3D ( 'NONE', #15067, #36249, #39910 ) ;
#5834=ORIENTED_EDGE ( 'NONE', *, *, #7475, .T. ) ;
#5837=CARTESIAN_POINT ( 'NONE',  ( 108.4684265045247997, -7.250697342233347165, -19.15521520033831138 ) ) ;
#5839=CARTESIAN_POINT ( 'NONE',  ( 110.0658483795247804, -0.7896495226426338832, -9.318865927141436245 ) ) ;
#5841=ORIENTED_EDGE ( 'NONE', *, *, #24435, .T. ) ;
#5842=VECTOR ( 'NONE', #42208, 1000.000000000000000 ) ;
#5846=CARTESIAN_POINT ( 'NONE',  ( 112.7491510812576934, -0.01829820670803256055, -12.14321520033831625 ) ) ;
#5849=ADVANCED_FACE ( 'NONE', ( #7700 ), #7928, .F. ) ;
#5851=CARTESIAN_POINT ( 'NONE',  ( 109.2324108795247923, -1.325403438956436419, -16.93181055722141792 ) ) ;
#5859=ORIENTED_EDGE ( 'NONE', *, *, #35036, .T. ) ;
#5862=CARTESIAN_POINT ( 'NONE',  ( 116.1777233795247781, -1.325403438956436419, -9.854619843455211026 ) ) ;
#5866=CARTESIAN_POINT ( 'NONE',  ( 116.1082702545247827, -10.62599879583958717, -15.77991374673208469 ) ) ;
#5867=CARTESIAN_POINT ( 'NONE',  ( 110.8992858795247827, -8.402594152722688392, -9.854619843455216355 ) ) ;
#5870=AXIS2_PLACEMENT_3D ( 'NONE', #5151, #8141, #35936 ) ;
#5872=CARTESIAN_POINT ( 'NONE',  ( 113.2987212410415765, 0.7607806665037644134, -12.14321520033829493 ) ) ;
#5873=CARTESIAN_POINT ( 'NONE',  ( 112.8439733795247832, -1.325403438956436419, -9.854619843455211026 ) ) ;
#5882=CARTESIAN_POINT ( 'NONE',  ( 116.5287898038745169, -11.91700341232977500, -21.13838130341561339 ) ) ;
#5883=EDGE_LOOP ( 'NONE', ( #20444, #11131, #27403, #31731 ) ) ;
#5887=DIRECTION ( 'NONE',  ( 0.000000000000000000, 0.3713878862591638574, -0.9284778069183724503 ) ) ;
#5891=CARTESIAN_POINT ( 'NONE',  ( 110.4131140045248287, 0.1403307496149616695, -15.46607636864997204 ) ) ;
#5900=EDGE_LOOP ( 'NONE', ( #21914, #10512, #19218, #30353 ) ) ;
#5903=DIRECTION ( 'NONE',  ( 0.000000000000000000, 0.000000000000000000, 1.000000000000000000 ) ) ;
#5907=CARTESIAN_POINT ( 'NONE',  ( 77.67538405296900805, -57.05391890152773726, -1.450191271579374774 ) ) ;
#5922=CARTESIAN_POINT ( 'NONE',  ( 113.2606921295247702, 0.8980012041604618078, -13.39321520033831447 ) ) ;
#5926=CARTESIAN_POINT ( 'NONE',  ( 109.4407702545248355, -10.62599879583953388, -15.77991374673210601 ) ) ;
#5930=DIRECTION ( 'NONE',  ( -0.9387755102040817867, 0.3445294493088593701, 0.000000000000000000 ) ) ;
#5932=CARTESIAN_POINT ( 'NONE',  ( 105.4819421295248247, -9.868328341294093420, -13.39321520033831447 ) ) ;
#5934=CARTESIAN_POINT ( 'NONE',  ( 114.7886608795247696, -1.325403438956436419, -16.93181055722141792 ) ) ;
#5950=VERTEX_POINT ( 'NONE', #14328 ) ;
#5953=CARTESIAN_POINT ( 'NONE',  ( 110.9687390045248350, 0.8980012041604421569, -15.77991374673208469 ) ) ;
#5958=EDGE_CURVE ( 'NONE', #40637, #10734, #39999, .T. ) ;
#5963=CARTESIAN_POINT ( 'NONE',  ( 106.1070202545248407, -10.62599879583958717, -15.77991374673208469 ) ) ;
#5974=CARTESIAN_POINT ( 'NONE',  ( 108.1906140045248463, -10.62599879583958717, -11.00651665394454604 ) ) ;
#5975=CARTESIAN_POINT ( 'NONE',  ( 111.3854577545248645, -2.791137627527939813, -18.39754474579286025 ) ) ;
#5976=CARTESIAN_POINT ( 'NONE',  ( 112.9828796295247884, -4.863998795839590272, -19.15521520033831493 ) ) ;
#5989=DIRECTION ( 'NONE',  ( 0.000000000000000000, 0.000000000000000000, -1.000000000000000000 ) ) ;
#5996=CARTESIAN_POINT ( 'NONE',  ( 106.8710046295248759, -4.863998795839590272, -18.39754474579285315 ) ) ;
#5997=CARTESIAN_POINT ( 'NONE',  ( 111.1770983795247787, -8.402594152722688392, -16.93181055722141792 ) ) ;
#5999=CARTESIAN_POINT ( 'NONE',  ( 70.98136983621358809, -24.64626890834123785, -5.214987668974215396 ) ) ;
#6013=CARTESIAN_POINT ( 'NONE',  ( 107.3571765045248299, -7.250697342233347165, -19.15521520033831138 ) ) ;
#6015=ORIENTED_EDGE ( 'NONE', *, *, #23687, .F. ) ;
#6018=CARTESIAN_POINT ( 'NONE',  ( 107.7738952545248310, -9.868328341294098749, -15.46607636864997204 ) ) ;
#6020=CARTESIAN_POINT ( 'NONE',  ( 115.4831921295247952, -9.868328341294093420, -13.39321520033836066 ) ) ;
#6031=CARTESIAN_POINT ( 'NONE',  ( 71.27025657587988405, -26.62083706768503077, -5.176427355402450914 ) ) ;
#6034=ORIENTED_EDGE ( 'NONE', *, *, #26253, .T. ) ;
#6037=CARTESIAN_POINT ( 'NONE',  ( 116.3166296295247832, -4.863998795839590272, -19.15521520033831493 ) ) ;
#6041=CARTESIAN_POINT ( 'NONE',  ( 115.8999108795247821, -1.325403438956436419, -16.93181055722141792 ) ) ;
#6045=CARTESIAN_POINT ( 'NONE',  ( 111.6632702545248605, -10.62599879583958717, -15.77991374673208469 ) ) ;
#6047=CARTESIAN_POINT ( 'NONE',  ( 112.9134265045247645, -7.250697342233347165, -19.15521520033831138 ) ) ;
#6063=VERTEX_POINT ( 'NONE', #12035 ) ;
#6066=CARTESIAN_POINT ( 'NONE',  ( 110.6214733795247867, -8.938348069036489818, -17.46756447353520159 ) ) ;
#6067=AXIS2_PLACEMENT_3D ( 'NONE', #27342, #3162, #30976 ) ;
#6068=CARTESIAN_POINT ( 'NONE',  ( 111.8716296295247901, -4.863998795839590272, -8.388885654883775800 ) ) ;
#6070=CARTESIAN_POINT ( 'NONE',  ( 116.8250374321000606, -1.625910394394186609, -17.50100589979427568 ) ) ;
#6071=CARTESIAN_POINT ( 'NONE',  ( 116.2471765045247594, -7.250697342233347165, -19.15521520033831138 ) ) ;
#6078=CARTESIAN_POINT ( 'NONE',  ( 116.8014327639767771, 1.999291220100584354, -5.886126520694280551 ) ) ;
#6081=CARTESIAN_POINT ( 'NONE',  ( 109.3713171295247832, 0.1403307496149613920, -13.39321520033831447 ) ) ;
#6087=CARTESIAN_POINT ( 'NONE',  ( 115.7628276191212819, 0.4261359969231631739, -12.14321520033831625 ) ) ;
#6099=CARTESIAN_POINT ( 'NONE',  ( 111.4549108795247747, -8.938348069036489818, -9.318865927141430916 ) ) ;
#6101=CARTESIAN_POINT ( 'NONE',  ( 116.1082702545247827, -10.62599879583958717, -15.77991374673208469 ) ) ;
#6105=CARTESIAN_POINT ( 'NONE',  ( 79.05243529145373316, 4.793396140045460108, -5.736853407927685389 ) ) ;
#6106=CARTESIAN_POINT ( 'NONE',  ( 113.3995983795247895, -8.402594152722688392, -16.93181055722141792 ) ) ;
#6107=VERTEX_POINT ( 'NONE', #1979 ) ;
#6108=ADVANCED_FACE ( 'NONE', ( #15450 ), #25715, .T. ) ;
#6109=CARTESIAN_POINT ( 'NONE',  ( 109.2294421295247275, -1.212886387410460065, -16.83921471868269393 ) ) ;
#6115=EDGE_CURVE ( 'NONE', #43568, #27006, #10016, .T. ) ;
#6116=ORIENTED_EDGE ( 'NONE', *, *, #1366, .T. ) ;
#6118=CARTESIAN_POINT ( 'NONE',  ( 116.2659068881580708, -12.01880880694303855, -20.89321520033831447 ) ) ;
#6127=CARTESIAN_POINT ( 'NONE',  ( 110.5520202545248054, 0.1403307496149616695, -11.32035403202665336 ) ) ;
#6136=ORIENTED_EDGE ( 'NONE', *, *, #33165, .T. ) ;
#6158=CARTESIAN_POINT ( 'NONE',  ( 111.3160046295247838, -4.863998795839590272, -7.631215200338315796 ) ) ;
#6159=CARTESIAN_POINT ( 'NONE',  ( 105.8292077545248446, -2.791137627527939813, -18.39754474579286025 ) ) ;
#6160=CARTESIAN_POINT ( 'NONE',  ( 106.6626452545248611, -9.868328341294098749, -15.46607636864997204 ) ) ;
#6169=CARTESIAN_POINT ( 'NONE',  ( 114.5108483795247878, -8.402594152722688392, -16.93181055722141792 ) ) ;
#6171=ORIENTED_EDGE ( 'NONE', *, *, #20591, .F. ) ;
#6191=CARTESIAN_POINT ( 'NONE',  ( 111.2465515045248168, -2.477300249445798297, -7.631215200338321125 ) ) ;
#6198=DIRECTION ( 'NONE',  ( 0.000000000000000000, 0.000000000000000000, -1.000000000000000000 ) ) ;
#6207=ORIENTED_EDGE ( 'NONE', *, *, #14497, .F. ) ;
#6209=DIRECTION ( 'NONE',  ( 0.000000000000000000, 0.000000000000000000, -1.000000000000000000 ) ) ;
#6211=VECTOR ( 'NONE', #19034, 1000.000000000000000 ) ;
#6212=CARTESIAN_POINT ( 'NONE',  ( 109.4407702545248355, -10.62599879583958717, -15.77991374673208469 ) ) ;
#6213=CARTESIAN_POINT ( 'NONE',  ( 114.4413952545248350, -9.868328341294098749, -15.46607636864997204 ) ) ;
#6214=CARTESIAN_POINT ( 'NONE',  ( 105.7597546295248350, -4.863998795839590272, -7.631215200338315796 ) ) ;
#6220=CARTESIAN_POINT ( 'NONE',  ( 64.84865456828643460, -21.86021636429758530, -5.893215200338315363 ) ) ;
#6233=CARTESIAN_POINT ( 'NONE',  ( 107.8433483795247838, -8.402594152722688392, -16.93181055722141792 ) ) ;
#6234=CARTESIAN_POINT ( 'NONE',  ( 112.1494421295248003, -9.868328341294093420, -13.39321520033831447 ) ) ;
#6236=CARTESIAN_POINT ( 'NONE',  ( 79.00611218289952831, -44.99489077589586827, -4.893215200338314474 ) ) ;
#6243=AXIS2_PLACEMENT_3D ( 'NONE', #30226, #12229, #5589 ) ;
#6245=VERTEX_POINT ( 'NONE', #16584 ) ;
#6249=EDGE_CURVE ( 'NONE', #40888, #36261, #27486, .T. ) ;
#6253=VECTOR ( 'NONE', #27239, 1000.000000000000000 ) ;
#6257=CARTESIAN_POINT ( 'NONE',  ( 109.2324108795247923, -1.325403438956436419, -16.93181055722141792 ) ) ;
#6264=CYLINDRICAL_SURFACE ( 'NONE', #38947, 5.132259260909266985 ) ;
#6267=DIRECTION ( 'NONE',  ( 0.000000000000000000, 0.000000000000000000, -1.000000000000000000 ) ) ;
#6271=AXIS2_PLACEMENT_3D ( 'NONE', #43628, #43406, #1887 ) ;
#6273=ORIENTED_EDGE ( 'NONE', *, *, #13370, .T. ) ;
#6276=CARTESIAN_POINT ( 'NONE',  ( 115.8304577545247582, -7.250697342233347165, -7.631215200338321125 ) ) ;
#6280=CARTESIAN_POINT ( 'NONE',  ( 114.9275671295247889, 0.1403307496149613920, -13.39321520033831447 ) ) ;
#6281=CARTESIAN_POINT ( 'NONE',  ( 111.4549108795247747, -8.938348069036489818, -9.318865927141430916 ) ) ;
#6283=CARTESIAN_POINT ( 'NONE',  ( 105.8292077545248446, -7.250697342233347165, -7.631215200338321125 ) ) ;
#6285=CARTESIAN_POINT ( 'NONE',  ( 115.6220983795247861, -0.7896495226426338832, -9.318865927141430916 ) ) ;
#6292=CARTESIAN_POINT ( 'NONE',  ( 109.4154010812577837, -0.01829820670803256055, -12.14321520033831625 ) ) ;
#6293=AXIS2_PLACEMENT_3D ( 'NONE', #449, #10948, #39202 ) ;
#6302=CARTESIAN_POINT ( 'NONE',  ( 108.8156921295247912, -9.868328341294093420, -13.39321520033831447 ) ) ;
#6306=CARTESIAN_POINT ( 'NONE',  ( 113.6079577545248043, -7.250697342233347165, -7.631215200338321125 ) ) ;
#6307=VERTEX_POINT ( 'NONE', #20456 ) ;
#6314=CARTESIAN_POINT ( 'NONE',  ( 108.1906140045248463, 0.1403307496149616695, -15.46607636864997204 ) ) ;
#6331=CARTESIAN_POINT ( 'NONE',  ( 110.7603796295247918, -4.863998795839590272, -19.15521520033831493 ) ) ;
#6338=CARTESIAN_POINT ( 'NONE',  ( 112.2883483795247770, -8.402594152722688392, -16.93181055722141792 ) ) ;
#6343=CARTESIAN_POINT ( 'NONE',  ( 79.61425486644590421, 5.119637120372100725, -6.626096235795095879 ) ) ;
#6347=ORIENTED_EDGE ( 'NONE', *, *, #38682, .F. ) ;
#6361=CARTESIAN_POINT ( 'NONE',  ( 106.8710046295248759, -4.863998795839590272, -18.39754474579285315 ) ) ;
#6363=DIRECTION ( 'NONE',  ( 0.000000000000000000, -1.000000000000000000, 1.195183497228115774E-16 ) ) ;
#6372=DIRECTION ( 'NONE',  ( -1.000000000000000000, 0.000000000000000000, 0.000000000000000000 ) ) ;
#6374=ADVANCED_FACE ( 'NONE', ( #8391 ), #40071, .F. ) ;
#6379=CARTESIAN_POINT ( 'NONE',  ( 70.19691569158496236, 3.834886253390165756, -6.893215200338315363 ) ) ;
#6388=AXIS2_PLACEMENT_3D ( 'NONE', #1481, #39573, #42776 ) ;
#6392=CARTESIAN_POINT ( 'NONE',  ( 107.2877233795247776, -8.938348069036489818, -17.46756447353520159 ) ) ;
#6393=CARTESIAN_POINT ( 'NONE',  ( 107.8433483795247838, -8.402594152722688392, -16.93181055722141792 ) ) ;
#6394=CARTESIAN_POINT ( 'NONE',  ( 106.8015515045248378, -6.936859964151250502, -18.39754474579286025 ) ) ;
#6404=CARTESIAN_POINT ( 'NONE',  ( 115.4831921295247952, -9.868328341294093420, -13.39321520033831447 ) ) ;
#6421=ORIENTED_EDGE ( 'NONE', *, *, #15843, .F. ) ;
#6426=CARTESIAN_POINT ( 'NONE',  ( 113.6079577545248043, -7.250697342233347165, -7.631215200338321125 ) ) ;
#6428=ORIENTED_EDGE ( 'NONE', *, *, #3317, .F. ) ;
#6429=ORIENTED_EDGE ( 'NONE', *, *, #9761, .F. ) ;
#6433=EDGE_CURVE ( 'NONE', #5950, #38773, #2660, .T. ) ;
#6439=DIRECTION ( 'NONE',  ( -1.000000000000000000, 0.000000000000000000, 0.000000000000000000 ) ) ;
#6446=ORIENTED_EDGE ( 'NONE', *, *, #26323, .F. ) ;
#6449=CARTESIAN_POINT ( 'NONE',  ( 108.5378796295247810, -4.863998795839590272, -19.15521520033831493 ) ) ;
#6450=CARTESIAN_POINT ( 'NONE',  ( 112.4272546295247821, -4.863998795839590272, -18.39754474579285315 ) ) ;
#6451=CARTESIAN_POINT ( 'NONE',  ( 109.3018640045248304, -10.62599879583958717, -11.00651665394454604 ) ) ;
#6456=CARTESIAN_POINT ( 'NONE',  ( 63.69189222814998175, -69.76310523276724496, -16.89321520033831447 ) ) ;
#6461=DIRECTION ( 'NONE',  ( 1.000000000000000000, 0.000000000000000000, 0.000000000000000000 ) ) ;
#6462=CARTESIAN_POINT ( 'NONE',  ( 107.6349890045248401, 0.8980012041604421569, -15.77991374673208469 ) ) ;
#6467=CARTESIAN_POINT ( 'NONE',  ( 108.4684265045247997, -2.791137627527939813, -8.388885654883777576 ) ) ;
#6468=CARTESIAN_POINT ( 'NONE',  ( 107.0793640045248196, 0.1403307496149616695, -15.46607636864997204 ) ) ;
#6479=ORIENTED_EDGE ( 'NONE', *, *, #14761, .T. ) ;
#6487=CARTESIAN_POINT ( 'NONE',  ( 115.2748327545248657, -2.477300249445798297, -19.15521520033831138 ) ) ;
#6489=CARTESIAN_POINT ( 'NONE',  ( 115.8304577545247582, -2.791137627527887410, -18.39754474579284249 ) ) ;
#6495=CARTESIAN_POINT ( 'NONE',  ( 116.2665301496069929, 0.3591747506842615789, -14.64321520033831447 ) ) ;
#6496=CARTESIAN_POINT ( 'NONE',  ( 112.4967077545247633, -7.250697342233347165, -7.631215200338321125 ) ) ;
#6498=CARTESIAN_POINT ( 'NONE',  ( 65.89554156778412164, -36.79628389010467515, -5.218367175095595556 ) ) ;
#6504=PLANE ( 'NONE',  #686 ) ;
#6505=CARTESIAN_POINT ( 'NONE',  ( 114.4413952545248350, 0.8980012041604421569, -11.00651665394454071 ) ) ;
#6509=CARTESIAN_POINT ( 'NONE',  ( 113.8857702545248003, 0.1403307496149616695, -11.32035403202665336 ) ) ;
#6513=CARTESIAN_POINT ( 'NONE',  ( 105.4819421295248247, 0.8980012041604618078, -13.39321520033831447 ) ) ;
#6514=DIRECTION ( 'NONE',  ( 1.000000000000000000, 0.000000000000000000, 0.000000000000000000 ) ) ;
#6515=CARTESIAN_POINT ( 'NONE',  ( 115.2748327545248657, -2.477300249445798297, -19.15521520033831138 ) ) ;
#6518=DIRECTION ( 'NONE',  ( -0.2588190451025185190, 0.9659258262890689783, 0.000000000000000000 ) ) ;
#6529=CARTESIAN_POINT ( 'NONE',  ( 61.69189222814998175, -40.21211973637273474, -23.89321520033831803 ) ) ;
#6532=CARTESIAN_POINT ( 'NONE',  ( 111.5938171295247940, -10.62599879583958540, -13.39321520033831447 ) ) ;
#6533=EDGE_LOOP ( 'NONE', ( #13112, #18857 ) ) ;
#6537=CARTESIAN_POINT ( 'NONE',  ( 116.3860827545247787, -6.936859964151250502, -8.388885654883777576 ) ) ;
#6541=CARTESIAN_POINT ( 'NONE',  ( 116.8098156552294000, 1.991649196448622039, -5.874233632703256269 ) ) ;
#6543=CARTESIAN_POINT ( 'NONE',  ( 105.5513952545248060, -9.868328341294098749, -15.46607636864997204 ) ) ;
#6544=CARTESIAN_POINT ( 'NONE',  ( 111.4073959279789960, 0.1843591316377651834, -14.64321520033828783 ) ) ;
#6556=CARTESIAN_POINT ( 'NONE',  ( 112.7050671295247923, -10.62599879583958540, -13.39321520033831447 ) ) ;
#6558=CARTESIAN_POINT ( 'NONE',  ( 115.5526452545247622, 0.8980012041604421569, -11.00651665394454071 ) ) ;
#6561=CARTESIAN_POINT ( 'NONE',  ( 111.5497331777918788, -0.01829820670803256055, -14.64321520033831447 ) ) ;
#6564=CARTESIAN_POINT ( 'NONE',  ( 108.1906140045248037, 0.1403307496149616695, -15.46607636864997204 ) ) ;
#6568=CARTESIAN_POINT ( 'NONE',  ( 79.48253577138170556, 5.079490123878041885, -6.428895771584159924 ) ) ;
#6575=AXIS2_PLACEMENT_3D ( 'NONE', #39139, #18620, #32064 ) ;
#6579=DIRECTION ( 'NONE',  ( 0.000000000000000000, 0.000000000000000000, -1.000000000000000000 ) ) ;
#6582=CARTESIAN_POINT ( 'NONE',  ( 116.1082702545247827, -10.62599879583958717, -15.77991374673208469 ) ) ;
#6584=PLANE ( 'NONE',  #14084 ) ;
#6587=MANIFOLD_SOLID_BREP ( 'NONE', #28685 ) ;
#6590=EDGE_LOOP ( 'NONE', ( #37068, #26186, #4604, #2995 ) ) ;
#6592=VECTOR ( 'NONE', #30057, 1000.000000000000000 ) ;
#6595=CARTESIAN_POINT ( 'NONE',  ( 78.26539945782576524, -58.08196990603463661, -0.6585284536243714015 ) ) ;
#6596=( BOUNDED_CURVE ( )  B_SPLINE_CURVE ( 3, ( #31668, #39190, #31895, #14806 ),
 .UNSPECIFIED., .F., .T. ) 
 B_SPLINE_CURVE_WITH_KNOTS ( ( 4, 4 ),
 ( 3.141592653589795336, 6.283185307179590673 ),
 .UNSPECIFIED. ) 
 CURVE ( )  GEOMETRIC_REPRESENTATION_ITEM ( )  RATIONAL_B_SPLINE_CURVE ( ( 1.000000000000000000, 0.3333333333333335369, 0.3333333333333335369, 1.000000000000000000 ) ) 
 REPRESENTATION_ITEM ( '' )  );
#6598=B_SPLINE_CURVE_WITH_KNOTS ( 'NONE', 3,
 ( #27925, #35403, #28144, #34943, #42502, #11262, #7375, #34729 ),
 .UNSPECIFIED., .F., .F.,
 ( 4, 2, 2, 4 ),
 ( 0.000000000000000000, 0.5000000000000000000, 0.7500000000000000000, 1.000000000000000000 ),
 .UNSPECIFIED. ) ;
#6612=CARTESIAN_POINT ( 'NONE',  ( 106.3848327545248651, -2.477300249445798297, -19.15521520033831138 ) ) ;
#6613=DIRECTION ( 'NONE',  ( 0.000000000000000000, 0.9284778069183717841, 0.3713878862591654673 ) ) ;
#6617=EDGE_LOOP ( 'NONE', ( #16693, #25151 ) ) ;
#6622=CARTESIAN_POINT ( 'NONE',  ( 107.0099108795247815, -8.938348069036489818, -9.318865927141430916 ) ) ;
#6623=CARTESIAN_POINT ( 'NONE',  ( 61.69189222814998175, -40.21211973637273474, -6.893215200338315363 ) ) ;
#6644=VECTOR ( 'NONE', #22480, 1000.000000000000114 ) ;
#6648=CARTESIAN_POINT ( 'NONE',  ( 107.8433483795247838, -0.7896495226426338832, -9.318865927141430916 ) ) ;
#6657=EDGE_CURVE ( 'NONE', #38752, #33939, #35684, .T. ) ;
#6671=CARTESIAN_POINT ( 'NONE',  ( 107.0099108795247815, -8.938348069036489818, -9.318865927141430916 ) ) ;
#6673=CARTESIAN_POINT ( 'NONE',  ( 107.9822546295247889, -4.863998795839590272, -18.39754474579285315 ) ) ;
#6674=CARTESIAN_POINT ( 'NONE',  ( 108.6767858795247861, -0.7896495226426338832, -17.46756447353520159 ) ) ;
#6679=CARTESIAN_POINT ( 'NONE',  ( 112.3578015045248861, -2.477300249445798297, -7.631215200338321125 ) ) ;
#6686=CARTESIAN_POINT ( 'NONE',  ( 115.9693640045247776, 0.1403307496149616695, -15.46607636864997204 ) ) ;
#6687=ORIENTED_EDGE ( 'NONE', *, *, #20591, .T. ) ;
#6691=CARTESIAN_POINT ( 'NONE',  ( 108.0517077545248696, -2.791137627527939813, -18.39754474579286025 ) ) ;
#6692=CARTESIAN_POINT ( 'NONE',  ( 105.6208483795248299, -8.402594152722688392, -16.93181055722141792 ) ) ;
#6693=EDGE_CURVE ( 'NONE', #28148, #15377, #10642, .T. ) ;
#6704=ORIENTED_EDGE ( 'NONE', *, *, #28576, .F. ) ;
#6706=AXIS2_PLACEMENT_3D ( 'NONE', #25280, #14790, #1322 ) ;
#6707=ORIENTED_EDGE ( 'NONE', *, *, #32913, .F. ) ;
#6712=ORIENTED_EDGE ( 'NONE', *, *, #22060, .F. ) ;
#6715=CARTESIAN_POINT ( 'NONE',  ( 115.4137390045248566, 0.8980012041604421569, -15.77991374673208469 ) ) ;
#6716=CARTESIAN_POINT ( 'NONE',  ( 115.5526452545247622, -9.868328341294102302, -15.46607636865001645 ) ) ;
#6726=CARTESIAN_POINT ( 'NONE',  ( 65.96249443994719286, -37.38467533475423465, -4.893215200338314474 ) ) ;
#6732=CARTESIAN_POINT ( 'NONE',  ( 73.53114257624162065, -54.10809544429395856, -19.39321520033831447 ) ) ;
#6733=CARTESIAN_POINT ( 'NONE',  ( 115.6915515045247531, -2.477300249445798297, -7.631215200338321125 ) ) ;
#6734=EDGE_CURVE ( 'NONE', #24095, #41818, #14382, .T. ) ;
#6738=CARTESIAN_POINT ( 'NONE',  ( 112.0105358795248804, -8.402594152722688392, -9.854619843455216355 ) ) ;
#6743=CARTESIAN_POINT ( 'NONE',  ( 106.5931921295248372, 0.8980012041604618078, -13.39321520033831447 ) ) ;
#6744=LINE ( 'NONE', #44374, #21890 ) ;
#6745=CARTESIAN_POINT ( 'NONE',  ( 109.9269421295247753, 0.8980012041604618078, -13.39321520033831447 ) ) ;
#6763=CARTESIAN_POINT ( 'NONE',  ( 116.8252597214867308, -1.616710930489624776, -17.49401746026956772 ) ) ;
#6764=CARTESIAN_POINT ( 'NONE',  ( 113.8163171295247764, -10.62599879583958540, -13.39321520033831447 ) ) ;
#6768=CARTESIAN_POINT ( 'NONE',  ( 116.1082702545247827, 0.1403307496149616695, -11.32035403202665336 ) ) ;
#6772=CARTESIAN_POINT ( 'NONE',  ( 105.7597546295248350, -4.863998795839590272, -18.39754474579285315 ) ) ;
#6774=CARTESIAN_POINT ( 'NONE',  ( 115.4137390045248566, -9.868328341294098749, -11.32035403202665869 ) ) ;
#6783=CARTESIAN_POINT ( 'NONE',  ( 117.0111608795247946, -1.325403438956436419, -16.93181055722141792 ) ) ;
#6787=CARTESIAN_POINT ( 'NONE',  ( 112.4967077545247633, -7.250697342233347165, -7.631215200338321125 ) ) ;
#6788=CARTESIAN_POINT ( 'NONE',  ( 70.19189222814998175, -56.50588100528558044, -39.03625958650156491 ) ) ;
#6789=CARTESIAN_POINT ( 'NONE',  ( 112.4967077545247633, -7.250697342233347165, -7.631215200338321125 ) ) ;
#6793=DIRECTION ( 'NONE',  ( -1.000000000000000000, 0.000000000000000000, 0.000000000000000000 ) ) ;
#6795=CARTESIAN_POINT ( 'NONE',  ( 107.9822546295247889, -4.863998795839590272, -18.39754474579285315 ) ) ;
#6802=ORIENTED_EDGE ( 'NONE', *, *, #27375, .T. ) ;
#6808=CARTESIAN_POINT ( 'NONE',  ( 87.44708369096657918, -25.99489077589588604, -11.39321520033831447 ) ) ;
#6811=CARTESIAN_POINT ( 'NONE',  ( 109.2324108795247923, -1.325403438956436419, -16.93181055722141792 ) ) ;
#6816=CIRCLE ( 'NONE', #2433, 15.89999999999999680 ) ;
#6819=ORIENTED_EDGE ( 'NONE', *, *, #11970, .F. ) ;
#6820=CARTESIAN_POINT ( 'NONE',  ( 107.2877233795247776, -1.325403438956436419, -9.854619843455211026 ) ) ;
#6824=CARTESIAN_POINT ( 'NONE',  ( 143.3676850761856940, -69.76310523276724496, 3.106784799661685526 ) ) ;
#6826=CARTESIAN_POINT ( 'NONE',  ( 78.01659465443469799, -57.60307796775784084, -1.014495093810897863 ) ) ;
#6831=FACE_BOUND ( 'NONE', #906, .T. ) ;
#6837=ORIENTED_EDGE ( 'NONE', *, *, #41809, .F. ) ;
#6839=CARTESIAN_POINT ( 'NONE',  ( 109.5102233795247884, -8.938348069036489818, -17.46756447353520159 ) ) ;
#6840=DIRECTION ( 'NONE',  ( 1.000000000000000000, 0.000000000000000000, 0.000000000000000000 ) ) ;
#6841=CARTESIAN_POINT ( 'NONE',  ( 105.2735827545248810, -6.936859964151250502, -8.388885654883777576 ) ) ;
#6842=CARTESIAN_POINT ( 'NONE',  ( 113.5403276191212854, 0.4261359969231631739, -12.14321520033833046 ) ) ;
#6844=ORIENTED_EDGE ( 'NONE', *, *, #35027, .F. ) ;
#6850=CARTESIAN_POINT ( 'NONE',  ( 112.0799890045248475, -9.868328341294098749, -11.32035403202665869 ) ) ;
#6865=ORIENTED_EDGE ( 'NONE', *, *, #10240, .T. ) ;
#6869=CARTESIAN_POINT ( 'NONE',  ( 107.7044421295247929, 0.8980012041604618078, -13.39321520033831447 ) ) ;
#6871=EDGE_LOOP ( 'NONE', ( #26996, #22919, #18770, #23061 ) ) ;
#6876=CARTESIAN_POINT ( 'NONE',  ( 117.2294421295247844, 1.035107641088057973, -4.893215200338314474 ) ) ;
#6888=CARTESIAN_POINT ( 'NONE',  ( 110.2047546295247855, -4.863998795839590272, -7.631215200338315796 ) ) ;
#6889=CARTESIAN_POINT ( 'NONE',  ( 109.7880358795247986, -8.402594152722688392, -9.854619843455216355 ) ) ;
#6890=CARTESIAN_POINT ( 'NONE',  ( 106.8015515045248378, -2.477300249445798297, -7.631215200338321125 ) ) ;
#6895=CARTESIAN_POINT ( 'NONE',  ( 112.9828796295247884, -4.863998795839590272, -19.15521520033831493 ) ) ;
#6896=DIRECTION ( 'NONE',  ( 0.9387755102040817867, -0.3445294493088593701, 0.000000000000000000 ) ) ;
#6902=CARTESIAN_POINT ( 'NONE',  ( 115.2053796295247849, -4.863998795839590272, -8.388885654883775800 ) ) ;
#6905=FACE_OUTER_BOUND ( 'NONE', #27682, .T. ) ;
#6908=CARTESIAN_POINT ( 'NONE',  ( 115.1359265045248605, -7.250697342233347165, -19.15521520033831138 ) ) ;
#6909=CARTESIAN_POINT ( 'NONE',  ( 107.4266296295248821, -4.863998795839590272, -8.388885654883775800 ) ) ;
#6927=CARTESIAN_POINT ( 'NONE',  ( 116.5944421295247793, -4.863998795839590272, -8.393215200338314474 ) ) ;
#6934=CARTESIAN_POINT ( 'NONE',  ( 114.9275671295247889, -10.62599879583958540, -13.39321520033831447 ) ) ;
#6939=CARTESIAN_POINT ( 'NONE',  ( 109.2294421295247844, 0.2400687412228638684, -12.14321520033831625 ) ) ;
#6940=EDGE_CURVE ( 'NONE', #3847, #34659, #43718, .T. ) ;
#6946=CARTESIAN_POINT ( 'NONE',  ( 84.72166425534338430, -29.42112683882138668, -9.627754957239334388 ) ) ;
#6952=CARTESIAN_POINT ( 'NONE',  ( 114.7886608795247696, -8.938348069036489818, -9.318865927141430916 ) ) ;
#6956=CARTESIAN_POINT ( 'NONE',  ( 112.4272546295247821, -4.863998795839541422, -18.39754474579285315 ) ) ;
#6957=CARTESIAN_POINT ( 'NONE',  ( 109.6491296295247793, -4.863998795839590272, -8.388885654883775800 ) ) ;
#6959=CARTESIAN_POINT ( 'NONE',  ( 109.2294315388255228, -7.824389221362666902, -17.82941758066625582 ) ) ;
#6961=CARTESIAN_POINT ( 'NONE',  ( 107.7044421295247929, 0.8980012041604618078, -13.39321520033831447 ) ) ;
#6963=CARTESIAN_POINT ( 'NONE',  ( 109.7880358795247986, -0.7896495226426338832, -17.46756447353520159 ) ) ;
#6970=AXIS2_PLACEMENT_3D ( 'NONE', #24595, #38478, #32090 ) ;
#6978=EDGE_CURVE ( 'NONE', #18690, #16480, #29681, .T. ) ;
#6981=CARTESIAN_POINT ( 'NONE',  ( 114.9275671295247889, -10.62599879583958540, -13.39321520033831447 ) ) ;
#6983=CARTESIAN_POINT ( 'NONE',  ( 65.82164714941100669, 4.169909004287361221, -7.393215200338315363 ) ) ;
#6984=DIRECTION ( 'NONE',  ( 0.9659258262890690894, 0.2588190451025180749, 0.000000000000000000 ) ) ;
#6985=DIRECTION ( 'NONE',  ( 4.336808689942015271E-16, -1.000000000000000000, 1.517883041479705024E-15 ) ) ;
#6992=CARTESIAN_POINT ( 'NONE',  ( 114.7886608795247696, -1.325403438956436419, -16.93181055722141792 ) ) ;
#6998=VERTEX_POINT ( 'NONE', #12667 ) ;
#7008=CARTESIAN_POINT ( 'NONE',  ( 110.8992858795247827, -0.7896495226426338832, -17.46756447353520159 ) ) ;
#7011=CARTESIAN_POINT ( 'NONE',  ( 109.2293480927346252, -6.550713907899789135, -8.000234073319102635 ) ) ;
#7013=CARTESIAN_POINT ( 'NONE',  ( 110.3436608795247764, -1.325403438956436419, -16.93181055722141792 ) ) ;
#7027=CARTESIAN_POINT ( 'NONE',  ( 108.1211608795247798, -1.325403438956436419, -16.93181055722141792 ) ) ;
#7029=DIRECTION ( 'NONE',  ( 0.000000000000000000, -1.000000000000000000, 0.000000000000000000 ) ) ;
#7030=VERTEX_POINT ( 'NONE', #43673 ) ;
#7036=VERTEX_POINT ( 'NONE', #25675 ) ;
#7037=CARTESIAN_POINT ( 'NONE',  ( 107.4960827545248350, -6.936859964151250502, -8.388885654883777576 ) ) ;
#7054=CARTESIAN_POINT ( 'NONE',  ( 108.8156921295247912, 0.8980012041604618078, -13.39321520033831447 ) ) ;
#7056=DIRECTION ( 'NONE',  ( 1.000000000000000000, 0.000000000000000000, 0.000000000000000000 ) ) ;
#7065=CARTESIAN_POINT ( 'NONE',  ( 113.1912390045248031, -9.868328341294098749, -11.32035403202665869 ) ) ;
#7078=DIRECTION ( 'NONE',  ( 0.000000000000000000, 0.000000000000000000, -1.000000000000000000 ) ) ;
#7085=CARTESIAN_POINT ( 'NONE',  ( 109.3713171295247832, -10.62599879583958540, -13.39321520033831447 ) ) ;
#7101=CARTESIAN_POINT ( 'NONE',  ( 66.82415148905926117, -40.21211973637273474, -7.393215200338315363 ) ) ;
#7105=CARTESIAN_POINT ( 'NONE',  ( 114.8581140045248361, 0.1403307496149616695, -15.46607636864997204 ) ) ;
#7106=CARTESIAN_POINT ( 'NONE',  ( 109.5102233795247884, -1.325403438956436419, -9.854619843455211026 ) ) ;
#7107=CARTESIAN_POINT ( 'NONE',  ( 115.8999108795247821, -1.325403438956436419, -16.93181055722141792 ) ) ;
#7108=CIRCLE ( 'NONE', #18764, 5.000000000000004441 ) ;
#7113=CARTESIAN_POINT ( 'NONE',  ( 112.6356140045247827, -10.62599879583958717, -11.00651665394454604 ) ) ;
#7114=CARTESIAN_POINT ( 'NONE',  ( 83.84865386347668448, -25.99489077589588604, -11.39321520033831447 ) ) ;
#7117=CARTESIAN_POINT ( 'NONE',  ( 64.69189222814998175, -41.76310523276723785, -20.39321520033831447 ) ) ;
#7119=CARTESIAN_POINT ( 'NONE',  ( 113.1912390045248031, 0.8980012041604421569, -15.77991374673208469 ) ) ;
#7120=CARTESIAN_POINT ( 'NONE',  ( 105.8292077545248446, -7.250697342233347165, -7.631215200338321125 ) ) ;
#7121=ORIENTED_EDGE ( 'NONE', *, *, #23071, .T. ) ;
#7125=CARTESIAN_POINT ( 'NONE',  ( 114.3024890045248156, 0.8980012041604421569, -15.77991374673208469 ) ) ;
#7126=CARTESIAN_POINT ( 'NONE',  ( 106.7320983795247855, -8.402594152722688392, -16.93181055722141792 ) ) ;
#7136=CARTESIAN_POINT ( 'NONE',  ( 110.2742077545248094, -2.791137627527939813, -18.39754474579286025 ) ) ;
#7140=CARTESIAN_POINT ( 'NONE',  ( 78.69189222814998175, -62.82237896425675672, -47.71602681600972318 ) ) ;
#7144=FACE_OUTER_BOUND ( 'NONE', #20978, .T. ) ;
#7145=CARTESIAN_POINT ( 'NONE',  ( 116.5944421295247793, 0.8980012041604618078, -13.39321520033831447 ) ) ;
#7152=EDGE_CURVE ( 'NONE', #22218, #26016, #13680, .T. ) ;
#7160=CARTESIAN_POINT ( 'NONE',  ( 111.8716296295247901, -4.863998795839590272, -19.15521520033831493 ) ) ;
#7165=DIRECTION ( 'NONE',  ( 0.000000000000000000, -1.000000000000000000, 0.000000000000000000 ) ) ;
#7166=CARTESIAN_POINT ( 'NONE',  ( 111.8716296295247901, -4.863998795839590272, -8.388885654883775800 ) ) ;
#7168=CARTESIAN_POINT ( 'NONE',  ( 109.2294546431617306, -8.427163038048201216, -17.40843757233801270 ) ) ;
#7173=CARTESIAN_POINT ( 'NONE',  ( 107.7044421295247929, 0.8980012041604618078, -13.39321520033831447 ) ) ;
#7176=FACE_OUTER_BOUND ( 'NONE', #35122, .T. ) ;
#7184=EDGE_LOOP ( 'NONE', ( #15252, #18459, #20537, #28291 ) ) ;
#7185=EDGE_CURVE ( 'NONE', #35850, #22322, #20642, .T. ) ;
#7191=CARTESIAN_POINT ( 'NONE',  ( 112.7745202545247878, -10.62599879583958717, -15.77991374673208469 ) ) ;
#7194=CARTESIAN_POINT ( 'NONE',  ( 117.1500671295247713, 0.1403307496149613920, -13.39321520033831447 ) ) ;
#7198=CARTESIAN_POINT ( 'NONE',  ( 76.69189222814998175, -50.16718729050181480, -4.893215200338314474 ) ) ;
#7200=CARTESIAN_POINT ( 'NONE',  ( 116.8028015045247940, -6.936859964151250502, -18.39754474579286025 ) ) ;
#7203=EDGE_CURVE ( 'NONE', #10687, #38595, #552, .T. ) ;
#7204=FACE_OUTER_BOUND ( 'NONE', #38585, .T. ) ;
#7212=CARTESIAN_POINT ( 'NONE',  ( 116.4555358795247884, -8.402594152722688392, -9.854619843455216355 ) ) ;
#7216=CARTESIAN_POINT ( 'NONE',  ( 85.06881860370363313, -29.48994604112064621, -10.44326554851264888 ) ) ;
#7217=CARTESIAN_POINT ( 'NONE',  ( 111.3160046295247838, -4.863998795839590272, -7.631215200338315796 ) ) ;
#7221=CARTESIAN_POINT ( 'NONE',  ( 109.2294548365425015, -3.781108693792560871, -7.969886040473982192 ) ) ;
#7223=CARTESIAN_POINT ( 'NONE',  ( 109.5102233795247884, -1.325403438956436419, -9.854619843455211026 ) ) ;
#7224=CARTESIAN_POINT ( 'NONE',  ( 117.1147479696649185, 1.569042602373198481, -21.39323033354518344 ) ) ;
#7227=CARTESIAN_POINT ( 'NONE',  ( 111.1770983795247787, -0.7896495226426338832, -9.318865927141430916 ) ) ;
#7228=CARTESIAN_POINT ( 'NONE',  ( 70.36267391504958368, -5.685877709920885259, -7.393215200338315363 ) ) ;
#7239=CARTESIAN_POINT ( 'NONE',  ( 107.4960827545248350, -6.936859964151250502, -8.388885654883777576 ) ) ;
#7241=CARTESIAN_POINT ( 'NONE',  ( 117.2294421295247844, 7.836001204160461420, -12.14321520033831625 ) ) ;
#7242=ORIENTED_EDGE ( 'NONE', *, *, #2511, .F. ) ;
#7249=CARTESIAN_POINT ( 'NONE',  ( 106.3153796295248412, -4.863998795839590272, -8.388885654883775800 ) ) ;
#7266=CARTESIAN_POINT ( 'NONE',  ( 106.4542858795248179, -0.7896495226426338832, -17.46756447353520159 ) ) ;
#7268=CARTESIAN_POINT ( 'NONE',  ( 113.9094545411902857, -0.3595008806742185925, -10.82052240173742064 ) ) ;
#7269=VECTOR ( 'NONE', #892, 1000.000000000000000 ) ;
#7277=CARTESIAN_POINT ( 'NONE',  ( 109.2781797178594019, -0.3595008806742686081, -15.96590799893915857 ) ) ;
#7279=CARTESIAN_POINT ( 'NONE',  ( 110.8298327545248299, -6.936859964151250502, -8.388885654883777576 ) ) ;
#7280=DIRECTION ( 'NONE',  ( 0.000000000000000000, 1.069961080215129965E-32, -1.000000000000000000 ) ) ;
#7297=VERTEX_POINT ( 'NONE', #23382 ) ;
#7300=CARTESIAN_POINT ( 'NONE',  ( 106.6626452545248611, 0.8980012041604421569, -11.00651665394454071 ) ) ;
#7306=CARTESIAN_POINT ( 'NONE',  ( 79.40485529179196078, 5.048385126289187674, -20.47678328014367821 ) ) ;
#7319=CARTESIAN_POINT ( 'NONE',  ( 115.4831921295247952, -9.868328341294093420, -13.39321520033831447 ) ) ;
#7320=CARTESIAN_POINT ( 'NONE',  ( 110.9687390045248350, -9.868328341294098749, -11.32035403202665869 ) ) ;
#7321=CARTESIAN_POINT ( 'NONE',  ( 112.2883483795247770, -8.402594152722688392, -16.93181055722141792 ) ) ;
#7322=CIRCLE ( 'NONE', #25562, 4.500000000000003553 ) ;
#7325=( BOUNDED_CURVE ( )  B_SPLINE_CURVE ( 3, ( #1744, #39612, #8600, #15896 ),
 .UNSPECIFIED., .F., .T. ) 
 B_SPLINE_CURVE_WITH_KNOTS ( ( 4, 4 ),
 ( 2.617993877991494855, 4.712388980384689674 ),
 .UNSPECIFIED. ) 
 CURVE ( )  GEOMETRIC_REPRESENTATION_ITEM ( )  RATIONAL_B_SPLINE_CURVE ( ( 1.000000000000000000, 0.6666666666666670737, 0.6666666666666670737, 1.000000000000000000 ) ) 
 REPRESENTATION_ITEM ( '' )  );
#7328=CARTESIAN_POINT ( 'NONE',  ( 113.3301452545248083, 0.8980012041604421569, -11.00651665394454071 ) ) ;
#7334=CARTESIAN_POINT ( 'NONE',  ( 112.7745202545247878, -10.62599879583958717, -15.77991374673208469 ) ) ;
#7335=CARTESIAN_POINT ( 'NONE',  ( 115.7610046295247912, -4.863998795839590272, -18.39754474579285315 ) ) ;
#7336=ORIENTED_EDGE ( 'NONE', *, *, #11969, .T. ) ;
#7337=FACE_OUTER_BOUND ( 'NONE', #40602, .T. ) ;
#7341=CARTESIAN_POINT ( 'NONE',  ( 114.5108483795247878, -0.7896495226426338832, -9.318865927141430916 ) ) ;
#7342=CARTESIAN_POINT ( 'NONE',  ( 104.9263171295248327, 0.1403307496149613920, -13.39321520033831447 ) ) ;
#7348=ORIENTED_EDGE ( 'NONE', *, *, #32913, .T. ) ;
#7350=ADVANCED_FACE ( 'NONE', ( #19958 ), #6504, .F. ) ;
#7353=EDGE_LOOP ( 'NONE', ( #45122, #29834, #37218, #10005 ) ) ;
#7355=CARTESIAN_POINT ( 'NONE',  ( 105.6903015045248253, -2.477300249445798297, -7.631215200338321125 ) ) ;
#7356=CARTESIAN_POINT ( 'NONE',  ( 109.4407702545248355, 0.1403307496149616695, -11.32035403202665336 ) ) ;
#7366=CARTESIAN_POINT ( 'NONE',  ( 115.4831921295247952, 0.8980012041604618078, -13.39321520033831447 ) ) ;
#7367=VECTOR ( 'NONE', #21424, 1000.000000000000000 ) ;
#7372=ORIENTED_EDGE ( 'NONE', *, *, #21874, .F. ) ;
#7375=CARTESIAN_POINT ( 'NONE',  ( 64.22513517183551812, -35.03390339818633947, -5.893215200338315363 ) ) ;
#7380=CARTESIAN_POINT ( 'NONE',  ( 109.7884337908067920, 0.5115630086001619059, -12.14321520033828072 ) ) ;
#7381=CARTESIAN_POINT ( 'NONE',  ( 112.0799890045248475, 0.8980012041604421569, -15.77991374673208469 ) ) ;
#7386=CARTESIAN_POINT ( 'NONE',  ( 111.7327233795247849, -1.325403438956436419, -9.854619843455211026 ) ) ;
#7387=ORIENTED_EDGE ( 'NONE', *, *, #36889, .T. ) ;
#7389=CARTESIAN_POINT ( 'NONE',  ( 109.2295392859521570, -8.890170852696687831, -16.98076245472113044 ) ) ;
#7390=VECTOR ( 'NONE', #19709, 1000.000000000000000 ) ;
#7393=CARTESIAN_POINT ( 'NONE',  ( 115.8999108795247821, -1.325403438956436419, -16.93181055722141792 ) ) ;
#7394=CARTESIAN_POINT ( 'NONE',  ( 110.8992858795247827, -0.7896495226426338832, -17.46756447353520159 ) ) ;
#7409=CARTESIAN_POINT ( 'NONE',  ( 110.8298327545248299, -2.477300249445798297, -19.15521520033831138 ) ) ;
#7412=CARTESIAN_POINT ( 'NONE',  ( 116.7333483795247844, -8.402594152722688392, -16.93181055722141792 ) ) ;
#7417=CARTESIAN_POINT ( 'NONE',  ( 112.6586338361194919, 0.1075849324168598464, -12.14321520033831625 ) ) ;
#7418=CARTESIAN_POINT ( 'NONE',  ( 115.8999108795247821, -1.325403438956436419, -16.93181055722141792 ) ) ;
#7429=CARTESIAN_POINT ( 'NONE',  ( 114.9275671295247889, 0.1403307496149613920, -13.39321520033831447 ) ) ;
#7431=EDGE_CURVE ( 'NONE', #27006, #8254, #7952, .T. ) ;
#7433=CARTESIAN_POINT ( 'NONE',  ( 86.21853402767062846, -26.70494960632584736, -8.456736516205184628 ) ) ;
#7434=CARTESIAN_POINT ( 'NONE',  ( 111.8021765045248372, -7.250697342233347165, -19.15521520033831138 ) ) ;
#7438=CARTESIAN_POINT ( 'NONE',  ( 109.2294421276549912, -0.9135388418710063130, -9.738026583846760786 ) ) ;
#7440=CARTESIAN_POINT ( 'NONE',  ( 109.3713171295247832, 0.1403307496149613920, -13.39321520033831447 ) ) ;
#7445=CARTESIAN_POINT ( 'NONE',  ( 109.2324108795247923, -8.938348069036489818, -9.318865927141430916 ) ) ;
#7456=EDGE_CURVE ( 'NONE', #20884, #40668, #321, .T. ) ;
#7457=CARTESIAN_POINT ( 'NONE',  ( 114.4413952545248350, 0.8980012041604421569, -11.00651665394454071 ) ) ;
#7458=AXIS2_PLACEMENT_3D ( 'NONE', #39410, #8399, #39636 ) ;
#7468=CARTESIAN_POINT ( 'NONE',  ( 106.0375671295248310, 0.1403307496149613920, -13.39321520033831447 ) ) ;
#7475=EDGE_CURVE ( 'NONE', #34675, #36736, #5667, .T. ) ;
#7480=EDGE_CURVE ( 'NONE', #11473, #26016, #17879, .T. ) ;
#7486=EDGE_CURVE ( 'NONE', #28223, #31466, #21748, .T. ) ;
#7488=VERTEX_POINT ( 'NONE', #3517 ) ;
#7490=CARTESIAN_POINT ( 'NONE',  ( 112.2883483795247770, -8.402594152722688392, -16.93181055722141792 ) ) ;
#7494=CARTESIAN_POINT ( 'NONE',  ( 61.69189222814998175, -63.77884951796256274, -31.62409037935697143 ) ) ;
#7496=ORIENTED_EDGE ( 'NONE', *, *, #30687, .T. ) ;
#7497=DIRECTION ( 'NONE',  ( 0.000000000000000000, 0.9284778069183720062, 0.3713878862591650232 ) ) ;
#7502=CARTESIAN_POINT ( 'NONE',  ( 109.9963952545248134, -9.868328341294098749, -15.46607636864997204 ) ) ;
#7510=LINE ( 'NONE', #6236, #7708 ) ;
#7516=ORIENTED_EDGE ( 'NONE', *, *, #10853, .F. ) ;
#7517=AXIS2_PLACEMENT_3D ( 'NONE', #22594, #32842, #2063 ) ;
#7518=DIRECTION ( 'NONE',  ( 0.000000000000000000, 0.000000000000000000, -1.000000000000000000 ) ) ;
#7525=CARTESIAN_POINT ( 'NONE',  ( 108.7462390045248242, 0.8980012041604421569, -15.77991374673208469 ) ) ;
#7530=CARTESIAN_POINT ( 'NONE',  ( 62.92618109310924268, -32.76310523276723785, -23.89321520033831803 ) ) ;
#7531=DIRECTION ( 'NONE',  ( 0.000000000000000000, 0.000000000000000000, -1.000000000000000000 ) ) ;
#7534=EDGE_CURVE ( 'NONE', #38311, #36696, #11041, .T. ) ;
#7543=EDGE_LOOP ( 'NONE', ( #4128, #12032, #11215, #24908 ) ) ;
#7548=CARTESIAN_POINT ( 'NONE',  ( 113.4690515045247992, -6.936859964151250502, -18.39754474579286025 ) ) ;
#7550=CARTESIAN_POINT ( 'NONE',  ( 109.7185827545247889, -6.936859964151250502, -8.388885654883777576 ) ) ;
#7551=CARTESIAN_POINT ( 'NONE',  ( 113.2606921295247702, -9.868328341294093420, -13.39321520033831447 ) ) ;
#7556=CARTESIAN_POINT ( 'NONE',  ( 109.9269421295247753, 0.8980012041604618078, -13.39321520033831447 ) ) ;
#7563=CARTESIAN_POINT ( 'NONE',  ( 114.0941296295247867, -4.863998795839590272, -19.15521520033831493 ) ) ;
#7564=CARTESIAN_POINT ( 'NONE',  ( 113.5385046295247804, -4.863998795839590272, -18.39754474579285315 ) ) ;
#7578=ORIENTED_EDGE ( 'NONE', *, *, #8890, .T. ) ;
#7580=CARTESIAN_POINT ( 'NONE',  ( 106.9404577545248145, -7.250697342233347165, -7.631215200338321125 ) ) ;
#7581=AXIS2_PLACEMENT_3D ( 'NONE', #37428, #6198, #29920 ) ;
#7582=CARTESIAN_POINT ( 'NONE',  ( 112.5661608795247872, -1.325403438956436419, -16.93181055722141792 ) ) ;
#7590=ORIENTED_EDGE ( 'NONE', *, *, #11969, .F. ) ;
#7592=DIRECTION ( 'NONE',  ( 0.000000000000000000, 0.000000000000000000, -1.000000000000000000 ) ) ;
#7593=CARTESIAN_POINT ( 'NONE',  ( 112.8439733795247832, -8.938348069036489818, -17.46756447353520159 ) ) ;
#7594=DIRECTION ( 'NONE',  ( -1.000000000000000000, 0.000000000000000000, 0.000000000000000000 ) ) ;
#7598=EDGE_LOOP ( 'NONE', ( #32902, #5727, #2414, #21061 ) ) ;
#7601=CARTESIAN_POINT ( 'NONE',  ( 115.2053796295247849, -4.863998795839590272, -19.15521520033831493 ) ) ;
#7602=CARTESIAN_POINT ( 'NONE',  ( 85.11152112150389826, -28.35884296389746595, -9.118680713869798282 ) ) ;
#7609=CARTESIAN_POINT ( 'NONE',  ( 113.0523327545247838, -2.477300249445798297, -19.15521520033831138 ) ) ;
#7613=CIRCLE ( 'NONE', #44783, 1.300000000000000044 ) ;
#7614=CARTESIAN_POINT ( 'NONE',  ( 111.8021765045248372, -2.791137627527939813, -8.388885654883754484 ) ) ;
#7615=CARTESIAN_POINT ( 'NONE',  ( 110.8992858795247827, -8.402594152722688392, -9.854619843455216355 ) ) ;
#7618=CARTESIAN_POINT ( 'NONE',  ( 109.2294421586085775, -7.222005445833587167, -18.14121012771779462 ) ) ;
#7622=CARTESIAN_POINT ( 'NONE',  ( 111.0381921295247878, 0.8980012041604618078, -13.39321520033831447 ) ) ;
#7632=EDGE_CURVE ( 'NONE', #9687, #24866, #5765, .T. ) ;
#7638=CARTESIAN_POINT ( 'NONE',  ( 83.82415148905927538, -32.76310523276723785, -22.89321520033831803 ) ) ;
#7639=CARTESIAN_POINT ( 'NONE',  ( 109.2324108795247923, -8.938348069036489818, -9.318865927141430916 ) ) ;
#7641=LINE ( 'NONE', #10854, #18416 ) ;
#7643=CARTESIAN_POINT ( 'NONE',  ( 115.2748327545248657, -6.936859964151250502, -8.388885654883777576 ) ) ;
#7649=CARTESIAN_POINT ( 'NONE',  ( 113.3301452545248083, -9.868328341294098749, -15.46607636864997204 ) ) ;
#7652=CARTESIAN_POINT ( 'NONE',  ( 84.86020291624612355, -29.99489077589588959, -18.39321520033831803 ) ) ;
#7661=CARTESIAN_POINT ( 'NONE',  ( 113.4690515045247992, -6.936859964151250502, -18.39754474579286025 ) ) ;
#7665=CARTESIAN_POINT ( 'NONE',  ( 113.7468640045248236, -10.62599879583958717, -11.00651665394454604 ) ) ;
#7666=CIRCLE ( 'NONE', #33136, 3.000000000000002665 ) ;
#7670=CARTESIAN_POINT ( 'NONE',  ( 109.2293241013981060, -6.781090337013601754, -8.066615733728053073 ) ) ;
#7672=B_SPLINE_CURVE_WITH_KNOTS ( 'NONE', 3,
 ( #22369, #943, #25352, #2457, #28994, #42901, #36265, #18947, #39476, #33447, #2227, #26639, #16379, #30281, #39246, #12968, #21700, #35588, #18278, #13420, #20705, #41460, #37571, #27324, #17066, #30505, #20028, #3582, #6109, #17286 ),
 .UNSPECIFIED., .F., .F.,
 ( 4, 2, 1, 1, 1, 1, 1, 2, 2, 2, 2, 2, 1, 1, 1, 2, 2, 2, 4 ),
 ( 0.000000000000000000, 0.1250000000000580647, 0.1875000000000879297, 0.2187500000001020017, 0.2343750000001090517, 0.2421875000001116884, 0.2460937500001130485, 0.2480468750001137146, 0.2500000000001144085, 0.3750000000001373346, 0.4375000000001479927, 0.4687500000001532663, 0.4843750000001549871, 0.4921875000001567635, 0.4960937500001575962, 0.4980468750001580958, 0.5000000000001585398, 0.7500000000000792699, 1.000000000000000000 ),
 .UNSPECIFIED. ) ;
#7673=CARTESIAN_POINT ( 'NONE',  ( 113.2606921295247702, 0.8980012041604618078, -13.39321520033831447 ) ) ;
#7677=CARTESIAN_POINT ( 'NONE',  ( 111.3160046295247838, -4.863998795839590272, -7.631215200338315796 ) ) ;
#7679=ORIENTED_EDGE ( 'NONE', *, *, #25980, .T. ) ;
#7688=CARTESIAN_POINT ( 'NONE',  ( 112.9134265045247645, -7.250697342233347165, -19.15521520033831138 ) ) ;
#7696=AXIS2_PLACEMENT_3D ( 'NONE', #13674, #9574, #34829 ) ;
#7698=CARTESIAN_POINT ( 'NONE',  ( 115.6915515045247531, -2.477300249445798297, -7.631215200338321125 ) ) ;
#7700=FACE_OUTER_BOUND ( 'NONE', #27323, .T. ) ;
#7703=CARTESIAN_POINT ( 'NONE',  ( 64.47830633734803030, -35.88190373598614258, -5.786960771376335799 ) ) ;
#7708=VECTOR ( 'NONE', #20158, 1000.000000000000000 ) ;
#7718=CARTESIAN_POINT ( 'NONE',  ( 111.9410827545248708, -6.936859964151250502, -8.388885654883777576 ) ) ;
#7721=CARTESIAN_POINT ( 'NONE',  ( 114.0941296295247867, -4.863998795839638234, -8.388885654883775800 ) ) ;
#7727=CARTESIAN_POINT ( 'NONE',  ( 116.5944421295247793, -4.863998795839590272, -13.39321520033831447 ) ) ;
#7731=CARTESIAN_POINT ( 'NONE',  ( 110.7603796295247918, -4.863998795839590272, -8.388885654883775800 ) ) ;
#7732=AXIS2_PLACEMENT_3D ( 'NONE', #27357, #2948, #24379 ) ;
#7742=PLANE ( 'NONE',  #41933 ) ;
#7747=CARTESIAN_POINT ( 'NONE',  ( 114.2330358795247776, -8.402594152722688392, -9.854619843455216355 ) ) ;
#7759=EDGE_LOOP ( 'NONE', ( #27228, #6712, #33060, #34498 ) ) ;
#7761=AXIS2_PLACEMENT_3D ( 'NONE', #7798, #3917, #17836 ) ;
#7767=CARTESIAN_POINT ( 'NONE',  ( 71.37572422742091760, -11.86958442233774313, -21.89321520033831447 ) ) ;
#7782=CARTESIAN_POINT ( 'NONE',  ( 115.2748327545248657, -6.936859964151250502, -8.388885654883777576 ) ) ;
#7783=CARTESIAN_POINT ( 'NONE',  ( 111.5938171295247940, 0.1403307496149613920, -13.39321520033831447 ) ) ;
#7788=CARTESIAN_POINT ( 'NONE',  ( 106.1764733795248219, -8.938348069036489818, -17.46756447353520159 ) ) ;
#7795=CARTESIAN_POINT ( 'NONE',  ( 113.6774108795247997, -8.938348069036489818, -9.318865927141430916 ) ) ;
#7796=CARTESIAN_POINT ( 'NONE',  ( 109.7185827545247889, -6.936859964151250502, -8.388885654883777576 ) ) ;
#7797=ORIENTED_EDGE ( 'NONE', *, *, #17908, .T. ) ;
#7798=CARTESIAN_POINT ( 'NONE',  ( 79.72353890764954087, 4.236894767232761261, -4.893215200338314474 ) ) ;
#7816=CARTESIAN_POINT ( 'NONE',  ( 114.9970202545248412, -10.62599879583958717, -15.77991374673208469 ) ) ;
#7822=EDGE_CURVE ( 'NONE', #12720, #14709, #35539, .T. ) ;
#7825=ORIENTED_EDGE ( 'NONE', *, *, #33475, .T. ) ;
#7826=DIRECTION ( 'NONE',  ( -1.000000000000000000, 1.352015467487876840E-15, 0.000000000000000000 ) ) ;
#7828=CARTESIAN_POINT ( 'NONE',  ( 109.1629577545248395, -7.250697342233347165, -7.631215200338321125 ) ) ;
#7836=FACE_OUTER_BOUND ( 'NONE', #16378, .T. ) ;
#7837=CARTESIAN_POINT ( 'NONE',  ( 84.39081516114468684, -30.32262605123988664, -11.80406037722653600 ) ) ;
#7838=CARTESIAN_POINT ( 'NONE',  ( 115.8304577545247582, -7.250697342233347165, -7.631215200338321125 ) ) ;
#7843=CARTESIAN_POINT ( 'NONE',  ( 113.8163171295247764, -10.62599879583958540, -13.39321520033831447 ) ) ;
#7848=CARTESIAN_POINT ( 'NONE',  ( 111.9410827545248708, -6.936859964151250502, -8.388885654883788234 ) ) ;
#7849=CARTESIAN_POINT ( 'NONE',  ( 107.3571765045248299, -2.791137627527939813, -8.388885654883777576 ) ) ;
#7850=ORIENTED_EDGE ( 'NONE', *, *, #212, .T. ) ;
#7852=CARTESIAN_POINT ( 'NONE',  ( 109.2294272264277026, -3.501945941663147099, -18.33763782056176694 ) ) ;
#7855=CARTESIAN_POINT ( 'NONE',  ( 114.9970202545248412, 0.1403307496149616695, -11.32035403202665336 ) ) ;
#7856=CARTESIAN_POINT ( 'NONE',  ( 105.9681140045248355, -10.62599879583958717, -11.00651665394454604 ) ) ;
#7873=CARTESIAN_POINT ( 'NONE',  ( 111.3160046295247838, -4.863998795839590272, -7.631215200338315796 ) ) ;
#7874=LINE ( 'NONE', #25433, #22792 ) ;
#7876=CARTESIAN_POINT ( 'NONE',  ( 115.8999108795247821, -1.325403438956436419, -16.93181055722141792 ) ) ;
#7882=CARTESIAN_POINT ( 'NONE',  ( 109.9963952545248134, -9.868328341294098749, -15.46607636864997204 ) ) ;
#7893=CARTESIAN_POINT ( 'NONE',  ( 113.6774108795247997, -1.325403438956436419, -16.93181055722141792 ) ) ;
#7896=CARTESIAN_POINT ( 'NONE',  ( 86.38598499330589675, -26.29959636144449675, -8.402972644559891791 ) ) ;
#7897=CARTESIAN_POINT ( 'NONE',  ( 109.3018640045248304, -10.62599879583958717, -11.00651665394454604 ) ) ;
#7901=CARTESIAN_POINT ( 'NONE',  ( 109.2294671201922966, -5.181012237870030290, -7.812175924317291908 ) ) ;
#7903=CARTESIAN_POINT ( 'NONE',  ( 113.1217858795247935, -0.7896495226426338832, -17.46756447353520159 ) ) ;
#7905=CARTESIAN_POINT ( 'NONE',  ( 84.10271796608054728, -31.10763468207612092, -21.89321520033831447 ) ) ;
#7908=CARTESIAN_POINT ( 'NONE',  ( 109.4407702545248355, -10.62599879583958717, -15.77991374673208469 ) ) ;
#7917=CARTESIAN_POINT ( 'NONE',  ( 111.9410827545248708, -2.477300249445798297, -19.15521520033831138 ) ) ;
#7918=ADVANCED_FACE ( 'NONE', ( #37681 ), #31256, .T. ) ;
#7928=CYLINDRICAL_SURFACE ( 'NONE', #24522, 0.4999999999999970024 ) ;
#7940=LINE ( 'NONE', #8173, #40186 ) ;
#7944=CARTESIAN_POINT ( 'NONE',  ( 113.0523327545247838, -6.936859964151250502, -8.388885654883777576 ) ) ;
#7946=CARTESIAN_POINT ( 'NONE',  ( 114.1635827545248247, -6.936859964151250502, -8.388885654883788234 ) ) ;
#7952=CIRCLE ( 'NONE', #12325, 2.000000000000001776 ) ;
#7957=CARTESIAN_POINT ( 'NONE',  ( 108.7462390045248242, -9.868328341294098749, -11.32035403202665869 ) ) ;
#7983=CIRCLE ( 'NONE', #27667, 0.5000000000000004441 ) ;
#7993=CARTESIAN_POINT ( 'NONE',  ( 116.6749492131033747, -8.511528440524470440, -16.92981788454075698 ) ) ;
#7998=VERTEX_POINT ( 'NONE', #26524 ) ;
#8000=CARTESIAN_POINT ( 'NONE',  ( 115.6220983795247861, -0.7896495226426338832, -9.318865927141430916 ) ) ;
#8001=CARTESIAN_POINT ( 'NONE',  ( 115.8304577545247582, -2.791137627527939813, -18.39754474579286025 ) ) ;
#8002=CARTESIAN_POINT ( 'NONE',  ( 114.0941296295247867, -4.863998795839590272, -8.388885654883775800 ) ) ;
#8007=CARTESIAN_POINT ( 'NONE',  ( 106.2459265045248173, -7.250697342233347165, -19.15521520033831138 ) ) ;
#8012=DIRECTION ( 'NONE',  ( 0.3445294493088594256, 0.9387755102040817867, 0.000000000000000000 ) ) ;
#8015=CARTESIAN_POINT ( 'NONE',  ( 113.3995983795247895, -0.7896495226426338832, -9.318865927141430916 ) ) ;
#8016=CARTESIAN_POINT ( 'NONE',  ( 113.4690515045247992, -6.936859964151250502, -18.39754474579286025 ) ) ;
#8022=DIRECTION ( 'NONE',  ( 0.000000000000000000, -0.9284778069183722282, -0.3713878862591645791 ) ) ;
#8032=AXIS2_PLACEMENT_3D ( 'NONE', #7767, #28749, #43099 ) ;
#8036=CARTESIAN_POINT ( 'NONE',  ( 116.2471765045247594, -7.250697342233347165, -19.15521520033831138 ) ) ;
#8039=EDGE_LOOP ( 'NONE', ( #28305, #29492, #32787, #16315, #1338, #37364, #44950, #36108, #10743, #30641, #8524 ) ) ;
#8044=EDGE_CURVE ( 'NONE', #15763, #35799, #31323, .T. ) ;
#8046=ORIENTED_EDGE ( 'NONE', *, *, #2612, .T. ) ;
#8050=CARTESIAN_POINT ( 'NONE',  ( 113.1912390045248031, 0.8980012041604421569, -15.77991374673208469 ) ) ;
#8051=CIRCLE ( 'NONE', #2939, 18.00000000000000000 ) ;
#8056=LINE ( 'NONE', #29031, #42250 ) ;
#8061=AXIS2_PLACEMENT_3D ( 'NONE', #29277, #35877, #36326 ) ;
#8063=CARTESIAN_POINT ( 'NONE',  ( 114.7192077545248594, -7.250697342233347165, -7.631215200338321125 ) ) ;
#8066=VECTOR ( 'NONE', #26358, 1000.000000000000114 ) ;
#8067=EDGE_CURVE ( 'NONE', #42470, #42269, #17000, .T. ) ;
#8069=CARTESIAN_POINT ( 'NONE',  ( 63.04939936085997232, -37.71678474238356671, -4.998464946505073669 ) ) ;
#8070=CARTESIAN_POINT ( 'NONE',  ( 110.2047546295247855, -4.863998795839590272, -7.631215200338315796 ) ) ;
#8080=CARTESIAN_POINT ( 'NONE',  ( 109.2294421468926799, -10.01755377227571664, -11.02232003854844145 ) ) ;
#8082=CARTESIAN_POINT ( 'NONE',  ( 112.0105358795247810, -8.402594152722688392, -9.854619843455216355 ) ) ;
#8083=CARTESIAN_POINT ( 'NONE',  ( 107.0099108795247815, -8.938348069036489818, -9.318865927141430916 ) ) ;
#8100=CARTESIAN_POINT ( 'NONE',  ( 109.0935046295247872, -4.863998795839590272, -7.631215200338315796 ) ) ;
#8104=CARTESIAN_POINT ( 'NONE',  ( 112.9134265045247645, -2.791137627527939813, -8.388885654883777576 ) ) ;
#8112=CARTESIAN_POINT ( 'NONE',  ( 108.5378796295247810, -4.863998795839590272, -8.388885654883775800 ) ) ;
#8116=LINE ( 'NONE', #43221, #36941 ) ;
#8124=CARTESIAN_POINT ( 'NONE',  ( 115.3442858795247759, -8.402594152722688392, -9.854619843455216355 ) ) ;
#8129=CARTESIAN_POINT ( 'NONE',  ( 106.4542858795248179, -0.7896495226426338832, -17.46756447353520159 ) ) ;
#8131=VECTOR ( 'NONE', #44261, 1000.000000000000000 ) ;
#8133=CARTESIAN_POINT ( 'NONE',  ( 116.0829010812576882, -0.01829820670803256055, -12.14321520033834290 ) ) ;
#8136=CARTESIAN_POINT ( 'NONE',  ( 115.6220983795247861, -0.7896495226426338832, -9.318865927141430916 ) ) ;
#8137=CARTESIAN_POINT ( 'NONE',  ( 116.7648838078721525, 2.033349373364758961, -20.84824896580845177 ) ) ;
#8138=CARTESIAN_POINT ( 'NONE',  ( 83.88969763788190903, -31.68807350287827163, -22.38302129830086784 ) ) ;
#8141=DIRECTION ( 'NONE',  ( 0.000000000000000000, 0.000000000000000000, -1.000000000000000000 ) ) ;
#8144=ORIENTED_EDGE ( 'NONE', *, *, #20311, .F. ) ;
#8145=CARTESIAN_POINT ( 'NONE',  ( 116.5944421295247793, -9.863109299026486809, -13.29890625629612622 ) ) ;
#8150=CARTESIAN_POINT ( 'NONE',  ( 115.5526452545247622, 0.8980012041604421569, -11.00651665394454071 ) ) ;
#8151=AXIS2_PLACEMENT_3D ( 'NONE', #40976, #11239, #31751 ) ;
#8173=CARTESIAN_POINT ( 'NONE',  ( 143.3676850761856940, -69.76310523276724496, -32.79321520033831661 ) ) ;
#8177=CARTESIAN_POINT ( 'NONE',  ( 114.0246765045248196, -2.791137627527939813, -8.388885654883777576 ) ) ;
#8183=CARTESIAN_POINT ( 'NONE',  ( 116.0388171295248014, 0.1403307496149613920, -13.39321520033831447 ) ) ;
#8189=CARTESIAN_POINT ( 'NONE',  ( 107.5655358795247736, -8.402594152722688392, -9.854619843455216355 ) ) ;
#8200=CARTESIAN_POINT ( 'NONE',  ( 115.2748327545248657, -6.936859964151250502, -8.388885654883777576 ) ) ;
#8211=ORIENTED_EDGE ( 'NONE', *, *, #26672, .F. ) ;
#8221=FACE_OUTER_BOUND ( 'NONE', #22666, .T. ) ;
#8224=CARTESIAN_POINT ( 'NONE',  ( 116.5987716749792895, -9.866677412677834269, -13.52174868289714027 ) ) ;
#8226=FACE_OUTER_BOUND ( 'NONE', #39995, .T. ) ;
#8228=EDGE_LOOP ( 'NONE', ( #11434, #22844, #16388, #18425 ) ) ;
#8229=CARTESIAN_POINT ( 'NONE',  ( 114.5549666496844878, 0.5600166689815611054, -12.14321520033831625 ) ) ;
#8231=CARTESIAN_POINT ( 'NONE',  ( 111.3160046295247838, -4.863998795839590272, -18.39754474579285315 ) ) ;
#8232=CARTESIAN_POINT ( 'NONE',  ( 112.7050671295247923, 0.1403307496149613920, -13.39321520033831447 ) ) ;
#8237=CARTESIAN_POINT ( 'NONE',  ( 107.4960827545248350, -2.477300249445798297, -19.15521520033831138 ) ) ;
#8243=CARTESIAN_POINT ( 'NONE',  ( 111.8716296295247901, -4.863998795839590272, -19.15521520033831493 ) ) ;
#8244=CARTESIAN_POINT ( 'NONE',  ( 113.0523327545247838, -6.936859964151250502, -8.388885654883777576 ) ) ;
#8245=ORIENTED_EDGE ( 'NONE', *, *, #36969, .F. ) ;
#8249=CARTESIAN_POINT ( 'NONE',  ( 83.84865386347668448, -25.99489077589588604, -11.39321520033831447 ) ) ;
#8254=VERTEX_POINT ( 'NONE', #42503 ) ;
#8260=CARTESIAN_POINT ( 'NONE',  ( 111.0762212410415799, 0.7607806665037644134, -12.14321520033829316 ) ) ;
#8262=CARTESIAN_POINT ( 'NONE',  ( 107.7044421295247929, -9.868328341294093420, -13.39321520033831447 ) ) ;
#8274=CARTESIAN_POINT ( 'NONE',  ( 61.90822566489802625, -65.63993958762723935, -44.13121205742435649 ) ) ;
#8275=CARTESIAN_POINT ( 'NONE',  ( 109.4407702545248355, -10.62599879583958717, -15.77991374673208469 ) ) ;
#8281=LINE ( 'NONE', #39736, #12372 ) ;
#8285=CARTESIAN_POINT ( 'NONE',  ( 115.6220983795247861, -0.7896495226426338832, -9.318865927141430916 ) ) ;
#8288=CARTESIAN_POINT ( 'NONE',  ( 114.3719421295247827, 0.8980012041604618078, -13.39321520033831447 ) ) ;
#8293=CARTESIAN_POINT ( 'NONE',  ( 105.4819421295248247, 0.8980012041604618078, -13.39321520033831447 ) ) ;
#8298=CARTESIAN_POINT ( 'NONE',  ( 104.9957702545248566, 0.1403307496149616695, -11.32035403202665336 ) ) ;
#8300=ORIENTED_EDGE ( 'NONE', *, *, #39630, .F. ) ;
#8302=CARTESIAN_POINT ( 'NONE',  ( 109.2294421295247417, -9.077645375966321595, -9.469096113667132997 ) ) ;
#8304=CARTESIAN_POINT ( 'NONE',  ( 111.0381921295247878, -9.868328341294093420, -13.39321520033831447 ) ) ;
#8305=CARTESIAN_POINT ( 'NONE',  ( 105.5513952545248060, 0.8980012041604421569, -11.00651665394454071 ) ) ;
#8307=CARTESIAN_POINT ( 'NONE',  ( 82.42995973409283295, -31.76308506831635725, -22.83422094025958415 ) ) ;
#8308=EDGE_CURVE ( 'NONE', #21853, #25264, #13206, .T. ) ;
#8312=ADVANCED_FACE ( 'NONE', ( #991 ), #31355, .T. ) ;
#8323=EDGE_CURVE ( 'NONE', #31933, #18860, #24171, .T. ) ;
#8324=EDGE_CURVE ( 'NONE', #3191, #5950, #2733, .T. ) ;
#8328=CARTESIAN_POINT ( 'NONE',  ( 114.1635827545248389, -6.936859964151250502, -8.388885654883777576 ) ) ;
#8329=FACE_OUTER_BOUND ( 'NONE', #35749, .T. ) ;
#8334=CARTESIAN_POINT ( 'NONE',  ( 112.5661608795247872, -1.325403438956436419, -16.93181055722141792 ) ) ;
#8344=CARTESIAN_POINT ( 'NONE',  ( 109.1629577545248395, -2.791137627527939813, -18.39754474579286025 ) ) ;
#8349=CARTESIAN_POINT ( 'NONE',  ( 108.0517077545248696, -7.250697342233347165, -7.631215200338321125 ) ) ;
#8352=DIRECTION ( 'NONE',  ( -0.6836572958096082120, 0.7298031939408691215, 0.000000000000000000 ) ) ;
#8355=CARTESIAN_POINT ( 'NONE',  ( 106.4542858795248179, -8.402594152722688392, -9.854619843455216355 ) ) ;
#8357=CARTESIAN_POINT ( 'NONE',  ( 83.36817807618649567, -33.10911252753713541, -22.72403028787429591 ) ) ;
#8364=CARTESIAN_POINT ( 'NONE',  ( 112.4711464071292824, 0.2518737723193609224, -14.64321520033832691 ) ) ;
#8372=CARTESIAN_POINT ( 'NONE',  ( 111.6632702545248605, -10.62599879583958717, -15.77991374673208469 ) ) ;
#8382=DIRECTION ( 'NONE',  ( 0.1736481776669305255, 0.9848077530122081313, 0.000000000000000000 ) ) ;
#8384=CARTESIAN_POINT ( 'NONE',  ( 115.2090389883689880, 0.3193521225029610777, -12.14321520033831625 ) ) ;
#8391=FACE_OUTER_BOUND ( 'NONE', #2111, .T. ) ;
#8399=DIRECTION ( 'NONE',  ( 0.000000000000000000, -1.000000000000000000, 0.000000000000000000 ) ) ;
#8404=CARTESIAN_POINT ( 'NONE',  ( 113.5385046295247804, -4.863998795839590272, -7.631215200338315796 ) ) ;
#8405=CARTESIAN_POINT ( 'NONE',  ( 113.3995983795247895, -8.402594152722688392, -16.93181055722141792 ) ) ;
#8408=CARTESIAN_POINT ( 'NONE',  ( 84.39081516114413262, -30.32262605124143562, -12.39321520033834645 ) ) ;
#8415=CARTESIAN_POINT ( 'NONE',  ( 105.8292077545248446, -2.791137627527939813, -18.39754474579286025 ) ) ;
#8418=CARTESIAN_POINT ( 'NONE',  ( 77.12856116249137983, -44.30583187727815186, -6.893215200338315363 ) ) ;
#8425=EDGE_CURVE ( 'NONE', #31466, #28016, #26973, .T. ) ;
#8427=CARTESIAN_POINT ( 'NONE',  ( 115.4831921295247952, -9.868328341294093420, -13.39321520033831447 ) ) ;
#8430=ORIENTED_EDGE ( 'NONE', *, *, #2612, .F. ) ;
#8440=DIRECTION ( 'NONE',  ( 0.000000000000000000, 0.9284778069183720062, 0.3713878862591650232 ) ) ;
#8457=CARTESIAN_POINT ( 'NONE',  ( 108.5378796295247810, -4.863998795839590272, -8.388885654883775800 ) ) ;
#8458=CARTESIAN_POINT ( 'NONE',  ( 110.2047546295247855, -4.863998795839590272, -18.39754474579285315 ) ) ;
#8463=CARTESIAN_POINT ( 'NONE',  ( 106.8710046295248759, -4.863998795839590272, -7.631215200338315796 ) ) ;
#8466=CARTESIAN_POINT ( 'NONE',  ( 77.22947525540432423, -44.03086066871760096, -6.893215200338315363 ) ) ;
#8469=CARTESIAN_POINT ( 'NONE',  ( 109.0240515045248202, -2.477300249445798297, -7.631215200338321125 ) ) ;
#8470=CARTESIAN_POINT ( 'NONE',  ( 110.5520202545248054, 0.1403307496149616695, -11.32035403202665336 ) ) ;
#8471=ORIENTED_EDGE ( 'NONE', *, *, #35047, .T. ) ;
#8475=CARTESIAN_POINT ( 'NONE',  ( 82.38065881859543538, -29.99489077589589314, -15.39321520033831447 ) ) ;
#8479=VERTEX_POINT ( 'NONE', #38721 ) ;
#8487=CARTESIAN_POINT ( 'NONE',  ( 106.1764733795248219, -1.325403438956436419, -9.854619843455211026 ) ) ;
#8489=AXIS2_PLACEMENT_3D ( 'NONE', #20289, #3402, #17320 ) ;
#8495=CARTESIAN_POINT ( 'NONE',  ( 77.77634386988368931, 3.254514819260763581, -4.893215200338314474 ) ) ;
#8499=CARTESIAN_POINT ( 'NONE',  ( 62.25607609626064942, -65.18564391136567338, -45.10442085122217293 ) ) ;
#8500=CARTESIAN_POINT ( 'NONE',  ( 112.0105358795247810, -0.7896495226426338832, -17.46756447353520159 ) ) ;
#8509=CARTESIAN_POINT ( 'NONE',  ( 112.1494421295248003, 0.8980012041604618078, -13.39321520033831447 ) ) ;
#8511=CARTESIAN_POINT ( 'NONE',  ( 111.1076452545248259, 0.8980012041604421569, -11.00651665394454071 ) ) ;
#8517=CARTESIAN_POINT ( 'NONE',  ( 108.9545983795247821, -0.7896495226426338832, -9.318865927141430916 ) ) ;
#8522=CARTESIAN_POINT ( 'NONE',  ( 65.19189222814998175, -41.76310523276723785, -24.39321520033831447 ) ) ;
#8524=ORIENTED_EDGE ( 'NONE', *, *, #42676, .T. ) ;
#8526=CARTESIAN_POINT ( 'NONE',  ( 109.2294415708224591, -10.34084703323438958, -14.19095601892115255 ) ) ;
#8528=CARTESIAN_POINT ( 'NONE',  ( 112.9134265045247645, -2.791137627527939813, -8.388885654883777576 ) ) ;
#8529=CARTESIAN_POINT ( 'NONE',  ( 106.5237390045248418, 0.8980012041604421569, -15.77991374673208469 ) ) ;
#8531=PLANE ( 'NONE',  #24856 ) ;
#8532=CARTESIAN_POINT ( 'NONE',  ( 68.92755183904094451, -25.82220866885473853, -5.893215200338315363 ) ) ;
#8550=CARTESIAN_POINT ( 'NONE',  ( 115.9693640045247776, 0.1403307496149616695, -15.46607636864997204 ) ) ;
#8557=CARTESIAN_POINT ( 'NONE',  ( 116.8028015045247940, -6.936859964151250502, -18.39754474579286025 ) ) ;
#8558=CARTESIAN_POINT ( 'NONE',  ( 109.3018640045248304, 0.1403307496149616695, -15.46607636864997204 ) ) ;
#8568=CARTESIAN_POINT ( 'NONE',  ( 114.6936464071293784, 0.2518737723193609224, -14.64321520033831447 ) ) ;
#8570=CARTESIAN_POINT ( 'NONE',  ( 108.0517077545248696, -2.791137627527939813, -18.39754474579286025 ) ) ;
#8575=CARTESIAN_POINT ( 'NONE',  ( 108.3989733795248753, -8.938348069036489818, -17.46756447353520159 ) ) ;
#8579=DIRECTION ( 'NONE',  ( 1.000000000000000000, 0.000000000000000000, 0.000000000000000000 ) ) ;
#8581=CARTESIAN_POINT ( 'NONE',  ( 114.4413952545248350, 0.8980012041604421569, -11.00651665394454071 ) ) ;
#8586=CARTESIAN_POINT ( 'NONE',  ( 107.7738952545248310, 0.8980012041604421569, -11.00651665394454071 ) ) ;
#8589=ADVANCED_FACE ( 'NONE', ( #3844 ), #28933, .T. ) ;
#8590=CARTESIAN_POINT ( 'NONE',  ( 87.44708369096657918, -21.99489077589588604, -6.893215200338315363 ) ) ;
#8591=ORIENTED_EDGE ( 'NONE', *, *, #3448, .F. ) ;
#8592=CARTESIAN_POINT ( 'NONE',  ( 116.5263184158184799, -9.825083310266851555, -11.28323190290009492 ) ) ;
#8595=SHAPE_DEFINITION_REPRESENTATION ( #41973, #15458 ) ;
#8598=CARTESIAN_POINT ( 'NONE',  ( 108.8156921295247912, 0.8980012041604618078, -13.39321520033831447 ) ) ;
#8600=CARTESIAN_POINT ( 'NONE',  ( 83.46705746533211823, -32.83968548964498524, -20.89321520033831092 ) ) ;
#8601=CARTESIAN_POINT ( 'NONE',  ( 116.3860827545247787, -2.477300249445798297, -19.15521520033831138 ) ) ;
#8602=ORIENTED_EDGE ( 'NONE', *, *, #33649, .T. ) ;
#8609=VECTOR ( 'NONE', #42176, 1000.000000000000000 ) ;
#8612=CARTESIAN_POINT ( 'NONE',  ( 64.86955682001475054, -35.96757841592401661, -5.723731037142695044 ) ) ;
#8615=CARTESIAN_POINT ( 'NONE',  ( 109.8405644685027767, 0.6938714319018670640, -14.64321520033831447 ) ) ;
#8624=CARTESIAN_POINT ( 'NONE',  ( 115.5526452545247622, -9.868328341294098749, -15.46607636864997204 ) ) ;
#8628=CARTESIAN_POINT ( 'NONE',  ( 116.3860827545247787, -2.477300249445798297, -19.15521520033831138 ) ) ;
#8629=CARTESIAN_POINT ( 'NONE',  ( 110.9687390045248350, -9.868328341294098749, -11.32035403202665869 ) ) ;
#8630=DIRECTION ( 'NONE',  ( 0.000000000000000000, 0.9284778069183722282, 0.3713878862591645791 ) ) ;
#8633=CARTESIAN_POINT ( 'NONE',  ( 116.5249890045247980, -9.868328341294098749, -11.32035403202665869 ) ) ;
#8638=EDGE_CURVE ( 'NONE', #529, #18915, #28179, .T. ) ;
#8640=CARTESIAN_POINT ( 'NONE',  ( 109.6491296295247793, -4.863998795839590272, -8.388885654883775800 ) ) ;
#8641=ORIENTED_EDGE ( 'NONE', *, *, #25857, .T. ) ;
#8646=CYLINDRICAL_SURFACE ( 'NONE', #8929, 1.999999999999998668 ) ;
#8649=CARTESIAN_POINT ( 'NONE',  ( 109.7185827545247889, -6.936859964151250502, -8.388885654883777576 ) ) ;
#8655=CARTESIAN_POINT ( 'NONE',  ( 105.6903015045248253, -2.477300249445798297, -7.631215200338321125 ) ) ;
#8660=LINE ( 'NONE', #23248, #9499 ) ;
#8669=CARTESIAN_POINT ( 'NONE',  ( 116.6178968253198605, -9.773106258948061509, -14.47218176588315508 ) ) ;
#8677=CARTESIAN_POINT ( 'NONE',  ( 110.3436608795247764, -8.938348069036489818, -9.318865927141430916 ) ) ;
#8678=CARTESIAN_POINT ( 'NONE',  ( 109.9269421295247753, -9.868328341294093420, -13.39321520033831447 ) ) ;
#8679=CARTESIAN_POINT ( 'NONE',  ( 107.7044421295247929, -9.868328341294093420, -13.39321520033831447 ) ) ;
#8683=CARTESIAN_POINT ( 'NONE',  ( 107.2877233795247776, -8.938348069036489818, -17.46756447353520159 ) ) ;
#8688=CARTESIAN_POINT ( 'NONE',  ( 109.5102233795247884, -8.938348069036489818, -17.46756447353520159 ) ) ;
#8689=CARTESIAN_POINT ( 'NONE',  ( 74.19189222814998175, -41.76310523276723785, -24.39321520033831447 ) ) ;
#8706=CARTESIAN_POINT ( 'NONE',  ( 110.8116360982116788, 0.3867979994853637526, -12.14321520033833224 ) ) ;
#8708=CARTESIAN_POINT ( 'NONE',  ( 115.9693640045247776, -10.62599879583958717, -11.00651665394454604 ) ) ;
#8710=ORIENTED_EDGE ( 'NONE', *, *, #24838, .T. ) ;
#8714=( BOUNDED_CURVE ( )  B_SPLINE_CURVE ( 3, ( #34923, #31084, #14208, #14653 ),
 .UNSPECIFIED., .F., .F. ) 
 B_SPLINE_CURVE_WITH_KNOTS ( ( 4, 4 ),
 ( 1.570796326794895004, 2.525095272406109981 ),
 .UNSPECIFIED. ) 
 CURVE ( )  GEOMETRIC_REPRESENTATION_ITEM ( )  RATIONAL_B_SPLINE_CURVE ( ( 1.000000000000000000, 0.9255384209705489473, 0.9255384209705489473, 1.000000000000000000 ) ) 
 REPRESENTATION_ITEM ( '' )  );
#8718=CARTESIAN_POINT ( 'NONE',  ( 61.85355368920866681, -65.73604765264855132, -43.91139043025361133 ) ) ;
#8719=CARTESIAN_POINT ( 'NONE',  ( 105.4819421295248247, 0.8980012041604618078, -13.39321520033831447 ) ) ;
#8728=CARTESIAN_POINT ( 'NONE',  ( 113.4690515045247992, -2.477300249445798297, -7.631215200338321125 ) ) ;
#8730=CARTESIAN_POINT ( 'NONE',  ( 112.2188952545247531, 0.8980012041604421569, -11.00651665394454071 ) ) ;
#8733=ORIENTED_EDGE ( 'NONE', *, *, #9214, .T. ) ;
#8736=CARTESIAN_POINT ( 'NONE',  ( 108.4684265045247997, -7.250697342233347165, -19.15521520033831138 ) ) ;
#8740=CARTESIAN_POINT ( 'NONE',  ( 117.1427234793119396, -11.22998347280470455, -5.531657149556616915 ) ) ;
#8741=ORIENTED_EDGE ( 'NONE', *, *, #18790, .F. ) ;
#8744=CARTESIAN_POINT ( 'NONE',  ( 109.2294576096139878, -8.937404933060426160, -16.93127305845157338 ) ) ;
#8747=CARTESIAN_POINT ( 'NONE',  ( 109.9963952545248134, -9.868328341294098749, -15.46607636864997204 ) ) ;
#8748=CARTESIAN_POINT ( 'NONE',  ( 114.7886608795247696, -1.325403438956436419, -16.93181055722141792 ) ) ;
#8752=CARTESIAN_POINT ( 'NONE',  ( 70.07290130439605491, -26.13131486452389041, -5.723131632646605738 ) ) ;
#8766=CARTESIAN_POINT ( 'NONE',  ( 108.1211608795247798, -8.938348069036489818, -9.318865927141430916 ) ) ;
#8767=DIRECTION ( 'NONE',  ( 0.000000000000000000, 0.000000000000000000, -1.000000000000000000 ) ) ;
#8769=CARTESIAN_POINT ( 'NONE',  ( 107.2877233795247776, -1.325403438956436419, -9.854619843455211026 ) ) ;
#8776=LINE ( 'NONE', #33149, #17752 ) ;
#8778=CARTESIAN_POINT ( 'NONE',  ( 116.3198046295247963, -4.863998795839590272, -8.393215200338314474 ) ) ;
#8779=CARTESIAN_POINT ( 'NONE',  ( 109.0240515045248202, -6.936859964151250502, -18.39754474579286025 ) ) ;
#8784=CARTESIAN_POINT ( 'NONE',  ( 86.51169734173754478, -25.99489077589583630, -7.893215200338315363 ) ) ;
#8788=CARTESIAN_POINT ( 'NONE',  ( 110.0654504682428865, 0.5115630086001619059, -14.64321520033831447 ) ) ;
#8790=CARTESIAN_POINT ( 'NONE',  ( 110.6909265045248247, -2.791137627527939813, -8.388885654883777576 ) ) ;
#8794=CARTESIAN_POINT ( 'NONE',  ( 106.2459265045248173, -7.250697342233347165, -19.15521520033831138 ) ) ;
#8799=CARTESIAN_POINT ( 'NONE',  ( 110.6214733795247867, -8.938348069036489818, -17.46756447353520159 ) ) ;
#8805=CARTESIAN_POINT ( 'NONE',  ( 105.4819421295248247, 0.8980012041604618078, -13.39321520033831447 ) ) ;
#8818=CARTESIAN_POINT ( 'NONE',  ( 108.7462390045248242, 0.8980012041604421569, -15.77991374673208469 ) ) ;
#8820=CARTESIAN_POINT ( 'NONE',  ( 116.7739797030027376, -3.961280311787784836, -18.49561454135252703 ) ) ;
#8821=CARTESIAN_POINT ( 'NONE',  ( 115.9693640045247776, -10.62599879583958717, -11.00651665394454604 ) ) ;
#8831=DIRECTION ( 'NONE',  ( 0.000000000000000000, 0.000000000000000000, -1.000000000000000000 ) ) ;
#8835=DIRECTION ( 'NONE',  ( 0.000000000000000000, -0.9284778069183722282, -0.3713878862591645791 ) ) ;
#8844=CARTESIAN_POINT ( 'NONE',  ( 115.3442858795247759, -8.402594152722688392, -9.854619843455216355 ) ) ;
#8848=CARTESIAN_POINT ( 'NONE',  ( 113.1217858795247935, -0.7896495226426338832, -17.46756447353520159 ) ) ;
#8849=CARTESIAN_POINT ( 'NONE',  ( 107.3571765045248299, -2.791137627527939813, -8.388885654883777576 ) ) ;
#8853=CARTESIAN_POINT ( 'NONE',  ( 113.1912390045248031, -9.868328341294098749, -11.32035403202665869 ) ) ;
#8854=VERTEX_POINT ( 'NONE', #29149 ) ;
#8859=CARTESIAN_POINT ( 'NONE',  ( 106.5931921295248372, -9.868328341294093420, -13.39321520033831447 ) ) ;
#8864=AXIS2_PLACEMENT_3D ( 'NONE', #44728, #10074, #10289 ) ;
#8873=CARTESIAN_POINT ( 'NONE',  ( 113.9552233795247815, -1.325403438956436419, -9.854619843455211026 ) ) ;
#8888=CARTESIAN_POINT ( 'NONE',  ( 115.1552801496069947, 0.3591747506842615789, -14.64321520033831447 ) ) ;
#8890=EDGE_CURVE ( 'NONE', #6245, #35524, #35984, .T. ) ;
#8894=AXIS2_PLACEMENT_3D ( 'NONE', #13925, #24855, #20326 ) ;
#8905=CARTESIAN_POINT ( 'NONE',  ( 110.4131140045248287, -10.62599879583958717, -11.00651665394454604 ) ) ;
#8906=CARTESIAN_POINT ( 'NONE',  ( 109.3018640045248304, 0.1403307496149616695, -15.46607636864997204 ) ) ;
#8907=VECTOR ( 'NONE', #35747, 1000.000000000000000 ) ;
#8908=CARTESIAN_POINT ( 'NONE',  ( 108.9545983795247821, -8.402594152722688392, -16.93181055722141792 ) ) ;
#8911=ORIENTED_EDGE ( 'NONE', *, *, #28125, .F. ) ;
#8914=DIRECTION ( 'NONE',  ( 1.000000000000000000, 0.000000000000000000, 0.000000000000000000 ) ) ;
#8917=CARTESIAN_POINT ( 'NONE',  ( 111.1770983795247787, -0.7896495226426338832, -9.318865927141430916 ) ) ;
#8929=AXIS2_PLACEMENT_3D ( 'NONE', #19131, #18901, #5438 ) ;
#8938=CARTESIAN_POINT ( 'NONE',  ( 113.5385046295247804, -4.863998795839590272, -7.631215200338315796 ) ) ;
#8948=CARTESIAN_POINT ( 'NONE',  ( 62.22678445075433018, -36.72958069525633817, -5.531797115907686191 ) ) ;
#8949=CARTESIAN_POINT ( 'NONE',  ( 61.79762598887304392, -65.86410496095400902, -43.61203885794885338 ) ) ;
#8956=EDGE_CURVE ( 'NONE', #38354, #25316, #6596, .T. ) ;
#8962=CARTESIAN_POINT ( 'NONE',  ( 114.5803015045248117, -2.477300249445798297, -7.631215200338321125 ) ) ;
#8964=CARTESIAN_POINT ( 'NONE',  ( 112.7745202545247878, -10.62599879583958717, -15.77991374673208469 ) ) ;
#8966=ORIENTED_EDGE ( 'NONE', *, *, #31267, .T. ) ;
#8968=CARTESIAN_POINT ( 'NONE',  ( 63.34631942287607842, -37.83243761108621328, -4.915970705112973960 ) ) ;
#8969=CARTESIAN_POINT ( 'NONE',  ( 107.2182702545248105, -10.62599879583958717, -15.77991374673208469 ) ) ;
#8974=ORIENTED_EDGE ( 'NONE', *, *, #25111, .T. ) ;
#8977=CARTESIAN_POINT ( 'NONE',  ( 109.2295516025745030, -10.43151013607753974, -13.43516445080127752 ) ) ;
#8979=CARTESIAN_POINT ( 'NONE',  ( 110.8298327545248299, -6.936859964151250502, -8.388885654883777576 ) ) ;
#8980=CARTESIAN_POINT ( 'NONE',  ( 110.8992858795247827, -8.402594152722688392, -9.854619843455216355 ) ) ;
#8983=CARTESIAN_POINT ( 'NONE',  ( 70.83207129814674374, -26.36080320520898823, -5.469311635450105236 ) ) ;
#8996=AXIS2_PLACEMENT_3D ( 'NONE', #34206, #40851, #30800 ) ;
#9000=CARTESIAN_POINT ( 'NONE',  ( 107.4960827545248350, -2.477300249445798297, -19.15521520033831138 ) ) ;
#9003=CARTESIAN_POINT ( 'NONE',  ( 108.8156921295247912, -9.868328341294093420, -13.39321520033831447 ) ) ;
#9005=EDGE_CURVE ( 'NONE', #6107, #2531, #26192, .T. ) ;
#9011=ORIENTED_EDGE ( 'NONE', *, *, #43495, .F. ) ;
#9013=CARTESIAN_POINT ( 'NONE',  ( 108.0517077545248696, -2.791137627527939813, -18.39754474579286025 ) ) ;
#9016=CARTESIAN_POINT ( 'NONE',  ( 64.17717360238856372, -59.27884951796255564, -42.87418841894955790 ) ) ;
#9018=CARTESIAN_POINT ( 'NONE',  ( 69.35389446611465303, -26.13003040042851666, -5.855554755288591373 ) ) ;
#9024=CARTESIAN_POINT ( 'NONE',  ( 108.5378796295247810, -4.863998795839590272, -8.388885654883775800 ) ) ;
#9028=CARTESIAN_POINT ( 'NONE',  ( 115.2053796295247849, -4.863998795839590272, -8.388885654883775800 ) ) ;
#9033=CARTESIAN_POINT ( 'NONE',  ( 109.5796765045248122, -7.250697342233347165, -19.15521520033831138 ) ) ;
#9035=CARTESIAN_POINT ( 'NONE',  ( 114.0246765045248196, -7.250697342233347165, -19.15521520033831138 ) ) ;
#9038=CARTESIAN_POINT ( 'NONE',  ( 107.4266296295248821, -4.863998795839590272, -19.15521520033831493 ) ) ;
#9049=CARTESIAN_POINT ( 'NONE',  ( 110.0658483795247804, -0.7896495226426338832, -9.318865927141430916 ) ) ;
#9051=CARTESIAN_POINT ( 'NONE',  ( 69.69189222814998175, -41.76310523276723785, -24.39321520033831447 ) ) ;
#9058=CARTESIAN_POINT ( 'NONE',  ( 113.0523327545247838, -6.936859964151250502, -8.388885654883788234 ) ) ;
#9062=DIRECTION ( 'NONE',  ( 0.000000000000000000, -1.000000000000000000, 0.000000000000000000 ) ) ;
#9074=CARTESIAN_POINT ( 'NONE',  ( 115.6220983795247861, -8.402594152722688392, -16.93181055722141792 ) ) ;
#9078=CARTESIAN_POINT ( 'NONE',  ( 115.8999108795247821, -8.938348069036489818, -9.318865927141430916 ) ) ;
#9079=CARTESIAN_POINT ( 'NONE',  ( 110.4825671295247815, 0.1403307496149613920, -13.39321520033831447 ) ) ;
#9085=CARTESIAN_POINT ( 'NONE',  ( 115.7610046295247912, -4.863998795839590272, -18.39754474579285315 ) ) ;
#9093=CARTESIAN_POINT ( 'NONE',  ( 116.6762522984324733, -11.82972831326674168, -21.28207584875485026 ) ) ;
#9101=CARTESIAN_POINT ( 'NONE',  ( 113.1217858795247935, -8.402594152722688392, -9.854619843455216355 ) ) ;
#9112=CARTESIAN_POINT ( 'NONE',  ( 72.75524511225664526, -21.99489077589588604, -18.39321520033831803 ) ) ;
#9113=CARTESIAN_POINT ( 'NONE',  ( 109.6491296295247793, -4.863998795839638234, -8.388885654883775800 ) ) ;
#9131=CARTESIAN_POINT ( 'NONE',  ( 112.3578015045248861, -2.477300249445798297, -7.631215200338321125 ) ) ;
#9132=CARTESIAN_POINT ( 'NONE',  ( 110.1353015045248469, -6.936859964151250502, -18.39754474579286025 ) ) ;
#9133=CARTESIAN_POINT ( 'NONE',  ( 110.2742077545248094, -2.791137627527939813, -18.39754474579286025 ) ) ;
#9137=CARTESIAN_POINT ( 'NONE',  ( 61.76986277844709861, -39.32091226840162079, -4.893215200338314474 ) ) ;
#9141=CARTESIAN_POINT ( 'NONE',  ( 107.7044421295247929, -9.868328341294093420, -13.39321520033831447 ) ) ;
#9143=CARTESIAN_POINT ( 'NONE',  ( 110.6909265045248247, -7.250697342233347165, -19.15521520033831138 ) ) ;
#9144=DIRECTION ( 'NONE',  ( 0.000000000000000000, 0.9284778069183720062, 0.3713878862591650232 ) ) ;
#9145=ORIENTED_EDGE ( 'NONE', *, *, #27260, .T. ) ;
#9157=ADVANCED_FACE ( 'NONE', ( #5432 ), #23927, .F. ) ;
#9165=CARTESIAN_POINT ( 'NONE',  ( 111.3854577545248645, -7.250697342233347165, -7.631215200338321125 ) ) ;
#9167=ORIENTED_EDGE ( 'NONE', *, *, #7185, .F. ) ;
#9168=VERTEX_POINT ( 'NONE', #15936 ) ;
#9187=CARTESIAN_POINT ( 'NONE',  ( 114.3719421295247827, 0.8980012041604618078, -13.39321520033831447 ) ) ;
#9188=CARTESIAN_POINT ( 'NONE',  ( 114.7886608795247696, -1.325403438956436419, -16.93181055722141792 ) ) ;
#9189=CARTESIAN_POINT ( 'NONE',  ( 112.5661608795247872, -8.938348069036489818, -9.318865927141430916 ) ) ;
#9190=AXIS2_PLACEMENT_3D ( 'NONE', #26427, #11848, #1565 ) ;
#9194=DIRECTION ( 'NONE',  ( 0.000000000000000000, 0.000000000000000000, -1.000000000000000000 ) ) ;
#9195=CARTESIAN_POINT ( 'NONE',  ( 106.8015515045248378, -2.477300249445798297, -7.631215200338321125 ) ) ;
#9198=CARTESIAN_POINT ( 'NONE',  ( 63.69189222814998175, -82.08636712479707853, -32.64558696907351987 ) ) ;
#9205=AXIS2_PLACEMENT_3D ( 'NONE', #13580, #109, #27490 ) ;
#9206=CARTESIAN_POINT ( 'NONE',  ( 116.3860827545247787, -2.477300249445798297, -19.15521520033831138 ) ) ;
#9207=CARTESIAN_POINT ( 'NONE',  ( 111.2465515045248168, -6.936859964151250502, -18.39754474579286025 ) ) ;
#9210=CARTESIAN_POINT ( 'NONE',  ( 69.24446145078422887, -25.84570955357843758, -5.871778085103664502 ) ) ;
#9214=EDGE_CURVE ( 'NONE', #30187, #24697, #5654, .T. ) ;
#9226=CARTESIAN_POINT ( 'NONE',  ( 108.6767858795247861, -0.7896495226426338832, -17.46756447353520159 ) ) ;
#9230=CARTESIAN_POINT ( 'NONE',  ( 108.1211608795247798, -1.325403438956436419, -16.93181055722141792 ) ) ;
#9241=LINE ( 'NONE', #24059, #42796 ) ;
#9242=DIRECTION ( 'NONE',  ( 0.3445294493088631449, 0.9387755102040804545, 0.000000000000000000 ) ) ;
#9248=CARTESIAN_POINT ( 'NONE',  ( 110.2047546295247855, -4.863998795839590272, -18.39754474579285315 ) ) ;
#9254=CARTESIAN_POINT ( 'NONE',  ( 112.8439733795247832, -1.325403438956436419, -9.854619843455211026 ) ) ;
#9258=CARTESIAN_POINT ( 'NONE',  ( 110.4825671295247815, -10.62599879583958540, -13.39321520033831447 ) ) ;
#9260=CARTESIAN_POINT ( 'NONE',  ( 114.7192077545248594, -7.250697342233347165, -7.631215200338321125 ) ) ;
#9263=( BOUNDED_CURVE ( )  B_SPLINE_CURVE ( 3, ( #37855, #19687, #38294, #41740 ),
 .UNSPECIFIED., .F., .T. ) 
 B_SPLINE_CURVE_WITH_KNOTS ( ( 4, 4 ),
 ( 3.141592653589795336, 6.283185307179590673 ),
 .UNSPECIFIED. ) 
 CURVE ( )  GEOMETRIC_REPRESENTATION_ITEM ( )  RATIONAL_B_SPLINE_CURVE ( ( 1.000000000000000000, 0.3333333333333335369, 0.3333333333333335369, 1.000000000000000000 ) ) 
 REPRESENTATION_ITEM ( '' )  );
#9273=EDGE_CURVE ( 'NONE', #11473, #6307, #41687, .T. ) ;
#9278=CARTESIAN_POINT ( 'NONE',  ( 107.8433483795247838, -0.7896495226426338832, -9.318865927141430916 ) ) ;
#9280=CARTESIAN_POINT ( 'NONE',  ( 116.8179980013510857, -1.923079332374536099, -17.71147565550795022 ) ) ;
#9281=CARTESIAN_POINT ( 'NONE',  ( 67.69189222814998175, -62.82237896425675672, -47.71602681600972318 ) ) ;
#9290=CARTESIAN_POINT ( 'NONE',  ( 109.3018640045248304, 0.1403307496149616695, -15.46607636864997204 ) ) ;
#9291=CARTESIAN_POINT ( 'NONE',  ( 79.05243529145373316, 4.793396140045460108, -21.04957699274893557 ) ) ;
#9301=CARTESIAN_POINT ( 'NONE',  ( 117.1500671295247713, 0.1403307496149613920, -13.39321520033831447 ) ) ;
#9305=CARTESIAN_POINT ( 'NONE',  ( 106.5931921295248372, -9.868328341294093420, -13.39321520033831447 ) ) ;
#9306=CARTESIAN_POINT ( 'NONE',  ( 109.5796765045248122, -2.791137627527939813, -8.388885654883777576 ) ) ;
#9307=CARTESIAN_POINT ( 'NONE',  ( 83.49267580666517574, -32.76310523276723785, -23.89321520033831803 ) ) ;
#9311=CARTESIAN_POINT ( 'NONE',  ( 112.4967077545247633, -2.791137627527939813, -18.39754474579286025 ) ) ;
#9319=CARTESIAN_POINT ( 'NONE',  ( 117.0649885480837042, -11.39702756529595540, -21.68909395195552392 ) ) ;
#9328=CARTESIAN_POINT ( 'NONE',  ( 110.2742077545248094, -2.791137627527939813, -18.39754474579286025 ) ) ;
#9338=FACE_OUTER_BOUND ( 'NONE', #4869, .T. ) ;
#9344=CARTESIAN_POINT ( 'NONE',  ( 117.2294421295247844, 0.6306099254434621715, -12.14321520033831625 ) ) ;
#9355=CARTESIAN_POINT ( 'NONE',  ( 112.9828796295247884, -4.863998795839590272, -19.15521520033831493 ) ) ;
#9356=CARTESIAN_POINT ( 'NONE',  ( 107.2182702545248105, 0.1403307496149616695, -11.32035403202665336 ) ) ;
#9357=CARTESIAN_POINT ( 'NONE',  ( 110.6909265045248247, -2.791137627527939813, -8.388885654883777576 ) ) ;
#9363=LINE ( 'NONE', #37153, #16540 ) ;
#9365=CARTESIAN_POINT ( 'NONE',  ( 106.5237390045248418, -9.868328341294098749, -11.32035403202665869 ) ) ;
#9367=CARTESIAN_POINT ( 'NONE',  ( 107.6349890045248401, 0.8980012041604421569, -15.77991374673208469 ) ) ;
#9370=CARTESIAN_POINT ( 'NONE',  ( 110.6196051332721879, 0.2334052082820642360, -14.64321520033831447 ) ) ;
#9382=VERTEX_POINT ( 'NONE', #13647 ) ;
#9385=CARTESIAN_POINT ( 'NONE',  ( 114.3719421295247827, 0.8980012041604618078, -13.39321520033831447 ) ) ;
#9395=CARTESIAN_POINT ( 'NONE',  ( 106.5237390045248418, 0.8980012041604421569, -15.77991374673208469 ) ) ;
#9402=ORIENTED_EDGE ( 'NONE', *, *, #38682, .T. ) ;
#9406=CARTESIAN_POINT ( 'NONE',  ( 112.8439733795247832, -8.938348069036489818, -17.46756447353520159 ) ) ;
#9407=CARTESIAN_POINT ( 'NONE',  ( 113.7468640045248236, 0.1403307496149616695, -15.46607636864997204 ) ) ;
#9408=CARTESIAN_POINT ( 'NONE',  ( 111.5243640045248412, -10.62599879583958717, -11.00651665394454604 ) ) ;
#9424=CARTESIAN_POINT ( 'NONE',  ( 107.2877233795247776, -1.325403438956436419, -9.854619843455211026 ) ) ;
#9425=CARTESIAN_POINT ( 'NONE',  ( 111.3160046295247838, -4.863998795839590272, -18.39754474579285315 ) ) ;
#9428=CARTESIAN_POINT ( 'NONE',  ( 70.04692138463070705, -26.21798220612133434, -5.722398249991135444 ) ) ;
#9432=EDGE_CURVE ( 'NONE', #18453, #20584, #11573, .T. ) ;
#9440=EDGE_CURVE ( 'NONE', #25300, #12207, #21778, .T. ) ;
#9444=CARTESIAN_POINT ( 'NONE',  ( 107.7738952545248310, 0.8980012041604421569, -11.00651665394454071 ) ) ;
#9449=CARTESIAN_POINT ( 'NONE',  ( 108.4684265045247997, -2.791137627527939813, -8.388885654883777576 ) ) ;
#9451=DIRECTION ( 'NONE',  ( 1.000000000000000000, 0.000000000000000000, 0.000000000000000000 ) ) ;
#9463=CARTESIAN_POINT ( 'NONE',  ( 67.69189222814998175, -59.27884951796255564, -42.87418841894956500 ) ) ;
#9472=CARTESIAN_POINT ( 'NONE',  ( 106.9404577545248145, -2.791137627527939813, -18.39754474579286025 ) ) ;
#9476=CARTESIAN_POINT ( 'NONE',  ( 112.3578015045248861, -6.936859964151250502, -18.39754474579286025 ) ) ;
#9480=CARTESIAN_POINT ( 'NONE',  ( 111.5243640045248412, -10.62599879583958717, -11.00651665394454604 ) ) ;
#9481=CARTESIAN_POINT ( 'NONE',  ( 111.9410827545248708, -2.477300249445798297, -19.15521520033831138 ) ) ;
#9498=CARTESIAN_POINT ( 'NONE',  ( 108.3295202545248657, -10.62599879583958717, -15.77991374673208469 ) ) ;
#9499=VECTOR ( 'NONE', #39899, 1000.000000000000000 ) ;
#9500=CARTESIAN_POINT ( 'NONE',  ( 109.7880358795247986, -8.402594152722688392, -9.854619843455216355 ) ) ;
#9502=CARTESIAN_POINT ( 'NONE',  ( 116.8928740015602870, 0.2848729546123598966, -14.64321520033831447 ) ) ;
#9507=CARTESIAN_POINT ( 'NONE',  ( 113.4690515045247992, -6.936859964151197211, -18.39754474579287447 ) ) ;
#9509=CARTESIAN_POINT ( 'NONE',  ( 116.6786527946934768, 2.098153082867008745, -6.056648293417564055 ) ) ;
#9511=CARTESIAN_POINT ( 'NONE',  ( 107.4960827545248350, -6.936859964151250502, -8.388885654883777576 ) ) ;
#9522=CARTESIAN_POINT ( 'NONE',  ( 117.0806140045248185, 0.1403307496149616695, -15.46607636864997204 ) ) ;
#9527=CARTESIAN_POINT ( 'NONE',  ( 111.6632702545248605, -10.62599879583958717, -15.77991374673208469 ) ) ;
#9528=CARTESIAN_POINT ( 'NONE',  ( 107.4960827545248350, -6.936859964151250502, -8.388885654883777576 ) ) ;
#9529=CARTESIAN_POINT ( 'NONE',  ( 83.49687201881269516, -32.20436853251904807, -23.72624644355049028 ) ) ;
#9533=CARTESIAN_POINT ( 'NONE',  ( 76.69189222814998175, -40.21211973637274184, -4.893215200338314474 ) ) ;
#9534=CARTESIAN_POINT ( 'NONE',  ( 111.5938171295247940, 0.1403307496149613920, -13.39321520033831447 ) ) ;
#9535=ORIENTED_EDGE ( 'NONE', *, *, #32802, .T. ) ;
#9539=CARTESIAN_POINT ( 'NONE',  ( 79.79010115959992788, 5.106172230548759572, -6.893215200338315363 ) ) ;
#9543=CARTESIAN_POINT ( 'NONE',  ( 114.1635827545248247, -2.477300249445798297, -19.15521520033830427 ) ) ;
#9552=CARTESIAN_POINT ( 'NONE',  ( 111.1076452545248259, -9.868328341294098749, -15.46607636864997204 ) ) ;
#9556=CARTESIAN_POINT ( 'NONE',  ( 112.6609831777918913, -0.01829820670813664396, -14.64321520033831447 ) ) ;
#9557=ORIENTED_EDGE ( 'NONE', *, *, #11734, .F. ) ;
#9562=ORIENTED_EDGE ( 'NONE', *, *, #23937, .F. ) ;
#9565=CARTESIAN_POINT ( 'NONE',  ( 76.69189222814998175, -46.76310523276723785, -4.893215200338314474 ) ) ;
#9566=CARTESIAN_POINT ( 'NONE',  ( 109.9963952545248134, -9.868328341294102302, -15.46607636865003244 ) ) ;
#9572=CARTESIAN_POINT ( 'NONE',  ( 113.1912390045248031, -9.868328341294098749, -11.32035403202665869 ) ) ;
#9574=DIRECTION ( 'NONE',  ( 0.000000000000000000, -1.000000000000000000, 0.000000000000000000 ) ) ;
#9584=CARTESIAN_POINT ( 'NONE',  ( 112.5661608795247872, -8.938348069036489818, -9.318865927141430916 ) ) ;
#9585=CARTESIAN_POINT ( 'NONE',  ( 106.7320983795247855, -8.402594152722688392, -16.93181055722141792 ) ) ;
#9586=CARTESIAN_POINT ( 'NONE',  ( 105.0652233795248378, -1.325403438956436419, -9.854619843455211026 ) ) ;
#9588=CARTESIAN_POINT ( 'NONE',  ( 64.44034106609326784, -36.97598037384660330, -5.426085069519624327 ) ) ;
#9596=CARTESIAN_POINT ( 'NONE',  ( 107.4960827545248350, -2.477300249445798297, -19.15521520033831138 ) ) ;
#9597=DIRECTION ( 'NONE',  ( -1.000000000000000000, 1.214306433183763980E-15, 0.000000000000000000 ) ) ;
#9612=ORIENTED_EDGE ( 'NONE', *, *, #21962, .T. ) ;
#9616=CARTESIAN_POINT ( 'NONE',  ( 111.6632702545248605, -10.62599879583958717, -15.77991374673208469 ) ) ;
#9619=ORIENTED_EDGE ( 'NONE', *, *, #36161, .T. ) ;
#9625=CARTESIAN_POINT ( 'NONE',  ( 108.8851452545248151, 0.8980012041604421569, -11.00651665394454071 ) ) ;
#9635=DIRECTION ( 'NONE',  ( 1.000000000000000000, 0.000000000000000000, 0.000000000000000000 ) ) ;
#9637=CARTESIAN_POINT ( 'NONE',  ( 106.8710046295248759, -4.863998795839590272, -7.631215200338315796 ) ) ;
#9638=CARTESIAN_POINT ( 'NONE',  ( 113.1217858795247935, -8.402594152722688392, -9.854619843455216355 ) ) ;
#9639=CARTESIAN_POINT ( 'NONE',  ( 108.6073327545248048, -2.477300249445798297, -19.15521520033831138 ) ) ;
#9645=CYLINDRICAL_SURFACE ( 'NONE', #40918, 2.000000000000000000 ) ;
#9658=CARTESIAN_POINT ( 'NONE',  ( 109.0935046295247872, -4.863998795839590272, -18.39754474579285315 ) ) ;
#9659=CARTESIAN_POINT ( 'NONE',  ( 112.3578015045248861, -6.936859964151250502, -18.39754474579286025 ) ) ;
#9661=CARTESIAN_POINT ( 'NONE',  ( 68.68839935636917460, -25.95913848132418522, -5.893215200338315363 ) ) ;
#9678=ORIENTED_EDGE ( 'NONE', *, *, #41297, .T. ) ;
#9681=CARTESIAN_POINT ( 'NONE',  ( 110.7603796295247918, -4.863998795839590272, -8.388885654883775800 ) ) ;
#9687=VERTEX_POINT ( 'NONE', #28001 ) ;
#9691=EDGE_CURVE ( 'NONE', #28792, #36696, #3800, .T. ) ;
#9702=CARTESIAN_POINT ( 'NONE',  ( 107.0793640045248196, 0.1403307496149616695, -15.46607636864997204 ) ) ;
#9707=CARTESIAN_POINT ( 'NONE',  ( 105.6208483795248299, -0.7896495226426338832, -9.318865927141430916 ) ) ;
#9709=CARTESIAN_POINT ( 'NONE',  ( 109.2296347500660829, -1.724019187123235541, -17.33431401656127235 ) ) ;
#9711=CARTESIAN_POINT ( 'NONE',  ( 108.8851452545248151, 0.8980012041604421569, -11.00651665394454071 ) ) ;
#9713=CARTESIAN_POINT ( 'NONE',  ( 114.7886608795247696, -8.938348069036489818, -9.318865927141430916 ) ) ;
#9733=CARTESIAN_POINT ( 'NONE',  ( 109.0240515045248202, -6.936859964151250502, -18.39754474579286025 ) ) ;
#9736=CARTESIAN_POINT ( 'NONE',  ( 111.9410827545248708, -2.477300249445798297, -19.15521520033831138 ) ) ;
#9738=CARTESIAN_POINT ( 'NONE',  ( 90.67797751089673852, -17.83979763915464289, -21.89321520033831447 ) ) ;
#9740=CARTESIAN_POINT ( 'NONE',  ( 113.1912390045248031, -9.868328341294150263, -11.32035403202671020 ) ) ;
#9743=CARTESIAN_POINT ( 'NONE',  ( 114.2372320646196897, 0.6269505268395592079, -14.64321520033831447 ) ) ;
#9744=CARTESIAN_POINT ( 'NONE',  ( 108.8156921295247912, -9.868328341294093420, -13.39321520033831447 ) ) ;
#9745=CARTESIAN_POINT ( 'NONE',  ( 111.5497331777918788, -0.01829820670803256055, -14.64321520033831447 ) ) ;
#9748=DIRECTION ( 'NONE',  ( 0.9999995469159186356, 0.0009519285464175526951, 0.000000000000000000 ) ) ;
#9750=DIRECTION ( 'NONE',  ( 1.000000000000000000, 0.000000000000000000, 0.000000000000000000 ) ) ;
#9757=LINE ( 'NONE', #2900, #42308 ) ;
#9760=CARTESIAN_POINT ( 'NONE',  ( 111.1076452545248259, 0.8980012041604421569, -11.00651665394454071 ) ) ;
#9761=EDGE_CURVE ( 'NONE', #21643, #9382, #22047, .T. ) ;
#9762=CARTESIAN_POINT ( 'NONE',  ( 106.9404577545248145, -2.791137627527939813, -18.39754474579286025 ) ) ;
#9763=CARTESIAN_POINT ( 'NONE',  ( 83.21177402427441905, -31.92419490535376170, -23.43773257735213988 ) ) ;
#9767=CARTESIAN_POINT ( 'NONE',  ( 113.1221837908068011, 0.5115630086001619059, -12.14321520033829493 ) ) ;
#9768=CARTESIAN_POINT ( 'NONE',  ( 115.5526452545247622, -9.868328341294098749, -15.46607636864997204 ) ) ;
#9769=ORIENTED_EDGE ( 'NONE', *, *, #28510, .T. ) ;
#9770=DIRECTION ( 'NONE',  ( 1.000000000000000000, 0.000000000000000000, 0.000000000000000000 ) ) ;
#9772=CARTESIAN_POINT ( 'NONE',  ( 79.39048153618716697, 5.042594898335129194, -6.287573381101518422 ) ) ;
#9776=CARTESIAN_POINT ( 'NONE',  ( 113.9552233795247815, -8.938348069036441856, -17.46756447353520514 ) ) ;
#9786=EDGE_CURVE ( 'NONE', #21756, #36673, #3330, .T. ) ;
#9788=CARTESIAN_POINT ( 'NONE',  ( 106.5931921295248372, -9.868328341294093420, -13.39321520033831447 ) ) ;
#9789=EDGE_CURVE ( 'NONE', #16272, #27457, #4931, .T. ) ;
#9799=B_SPLINE_CURVE_WITH_KNOTS ( 'NONE', 3,
 ( #41237, #20025, #33907, #44423, #2677, #12965, #16838, #9767, #13190, #23219 ),
 .UNSPECIFIED., .F., .F.,
 ( 4, 3, 3, 4 ),
 ( 0.000000000000000000, 0.0002476487219222810133, 0.0004952974148303629972, 0.0009534114850261790879 ),
 .UNSPECIFIED. ) ;
#9803=( BOUNDED_CURVE ( )  B_SPLINE_CURVE ( 2, ( #20974, #7277, #28939, #35070, #14352 ),
 .UNSPECIFIED., .F., .F. ) 
 B_SPLINE_CURVE_WITH_KNOTS ( ( 3, 2, 3 ),
 ( 0.6040431156034949955, 0.6125000000000000444, 0.6127876305315190786 ),
 .UNSPECIFIED. ) 
 CURVE ( )  GEOMETRIC_REPRESENTATION_ITEM ( )  RATIONAL_B_SPLINE_CURVE ( ( 0.9666851417651740608, 0.9485006404992010198, 1.000000000000000000, 0.9982484343581399244, 0.9965774773173300405 ) ) 
 REPRESENTATION_ITEM ( '' )  );
#9805=DIRECTION ( 'NONE',  ( 0.000000000000000000, 1.000000000000000000, 0.000000000000000000 ) ) ;
#9818=CARTESIAN_POINT ( 'NONE',  ( 107.8433483795247838, -0.7896495226426338832, -9.318865927141430916 ) ) ;
#9819=CARTESIAN_POINT ( 'NONE',  ( 107.4960827545248350, -6.936859964151250502, -8.388885654883777576 ) ) ;
#9820=CARTESIAN_POINT ( 'NONE',  ( 106.5237390045248418, -9.868328341294098749, -11.32035403202665869 ) ) ;
#9821=CARTESIAN_POINT ( 'NONE',  ( 64.35706024680830240, -36.56378831979270672, -5.594626812820024497 ) ) ;
#9823=ORIENTED_EDGE ( 'NONE', *, *, #98, .F. ) ;
#9830=CARTESIAN_POINT ( 'NONE',  ( 115.7610046295247912, -4.863998795839590272, -18.39754474579285315 ) ) ;
#9832=ORIENTED_EDGE ( 'NONE', *, *, #24371, .F. ) ;
#9841=EDGE_LOOP ( 'NONE', ( #10360, #6865 ) ) ;
#9853=CARTESIAN_POINT ( 'NONE',  ( 111.7327233795247849, -8.938348069036489818, -17.46756447353520159 ) ) ;
#9855=ORIENTED_EDGE ( 'NONE', *, *, #35878, .F. ) ;
#9856=VERTEX_POINT ( 'NONE', #39603 ) ;
#9860=CARTESIAN_POINT ( 'NONE',  ( 78.69189222814998175, -68.13214146720427777, -20.74076566292613677 ) ) ;
#9862=CARTESIAN_POINT ( 'NONE',  ( 64.69189222814998175, -41.76310523276723785, -47.71602681600972318 ) ) ;
#9873=AXIS2_PLACEMENT_3D ( 'NONE', #3769, #3994, #17469 ) ;
#9874=CARTESIAN_POINT ( 'NONE',  ( 107.7738952545248310, 0.8980012041604421569, -11.00651665394454071 ) ) ;
#9875=CARTESIAN_POINT ( 'NONE',  ( 115.2053796295247849, -4.863998795839590272, -8.388885654883775800 ) ) ;
#9876=CARTESIAN_POINT ( 'NONE',  ( 108.8156921295247912, 0.8980012041604618078, -13.39321520033831447 ) ) ;
#9889=CARTESIAN_POINT ( 'NONE',  ( 115.8999108795247821, -1.325403438956436419, -16.93181055722141792 ) ) ;
#9890=ORIENTED_EDGE ( 'NONE', *, *, #1715, .T. ) ;
#9891=DIRECTION ( 'NONE',  ( 0.000000000000000000, 0.000000000000000000, 1.000000000000000000 ) ) ;
#9894=CARTESIAN_POINT ( 'NONE',  ( 106.2459265045248173, -2.791137627527939813, -8.388885654883777576 ) ) ;
#9895=CARTESIAN_POINT ( 'NONE',  ( 111.6632702545248605, 0.1403307496149616695, -11.32035403202665336 ) ) ;
#9915=LINE ( 'NONE', #34060, #6253 ) ;
#9917=CARTESIAN_POINT ( 'NONE',  ( 115.6220983795247861, -0.7896495226426338832, -9.318865927141430916 ) ) ;
#9925=CARTESIAN_POINT ( 'NONE',  ( 112.9134265045247787, -7.250697342233347165, -19.15521520033830427 ) ) ;
#9927=CARTESIAN_POINT ( 'NONE',  ( 64.61935771200890599, -37.86087448816891765, -4.893215200338314474 ) ) ;
#9934=CARTESIAN_POINT ( 'NONE',  ( 114.1635827545248389, -2.477300249445798297, -19.15521520033831138 ) ) ;
#9938=CARTESIAN_POINT ( 'NONE',  ( 114.0941296295247867, -4.863998795839590272, -8.388885654883775800 ) ) ;
#9939=AXIS2_PLACEMENT_3D ( 'NONE', #10201, #2893, #9750 ) ;
#9943=CARTESIAN_POINT ( 'NONE',  ( 108.2600671295247992, -10.62599879583958540, -13.39321520033831447 ) ) ;
#9945=CARTESIAN_POINT ( 'NONE',  ( 113.3301452545248083, 0.8980012041604421569, -11.00651665394454071 ) ) ;
#9951=VERTEX_POINT ( 'NONE', #2176 ) ;
#9966=CARTESIAN_POINT ( 'NONE',  ( 115.1359265045248605, -7.250697342233347165, -19.15521520033831138 ) ) ;
#9972=CARTESIAN_POINT ( 'NONE',  ( 113.7722331777918896, -0.01829820670813664396, -14.64321520033831447 ) ) ;
#9973=CARTESIAN_POINT ( 'NONE',  ( 117.1003875888201406, 1.599829628806384463, -5.419835913930024063 ) ) ;
#9975=CARTESIAN_POINT ( 'NONE',  ( 108.3989733795248753, -1.325403438956436419, -9.854619843455211026 ) ) ;
#9976=CARTESIAN_POINT ( 'NONE',  ( 78.29371559379771384, 3.878430683262073408, -21.89321520033832513 ) ) ;
#9982=EDGE_CURVE ( 'NONE', #3603, #27652, #44167, .T. ) ;
#9989=EDGE_CURVE ( 'NONE', #21089, #24095, #28334, .T. ) ;
#9991=CARTESIAN_POINT ( 'NONE',  ( 109.3018640045248304, -10.62599879583958717, -11.00651665394454604 ) ) ;
#9992=CARTESIAN_POINT ( 'NONE',  ( 106.1764733795248219, -1.325403438956436419, -9.854619843455211026 ) ) ;
#9993=CARTESIAN_POINT ( 'NONE',  ( 82.84913590756312374, -31.80416417093374193, -23.17682243723843527 ) ) ;
#9998=CARTESIAN_POINT ( 'NONE',  ( 108.4684265045247997, -2.791137627527939813, -8.388885654883777576 ) ) ;
#10005=ORIENTED_EDGE ( 'NONE', *, *, #33681, .F. ) ;
#10006=CARTESIAN_POINT ( 'NONE',  ( 114.0246765045248196, -7.250697342233347165, -19.15521520033830427 ) ) ;
#10007=VECTOR ( 'NONE', #44477, 1000.000000000000000 ) ;
#10012=( NAMED_UNIT ( * ) PLANE_ANGLE_UNIT ( ) SI_UNIT ( $, .RADIAN. ) );
#10013=CARTESIAN_POINT ( 'NONE',  ( 85.75809888461174069, -18.45227461768569199, -4.893215200338314474 ) ) ;
#10016=CIRCLE ( 'NONE', #10717, 0.5000000000000004441 ) ;
#10018=CARTESIAN_POINT ( 'NONE',  ( 106.1764733795248219, -1.325403438956436419, -9.854619843455211026 ) ) ;
#10025=EDGE_CURVE ( 'NONE', #23154, #34675, #13675, .T. ) ;
#10027=ORIENTED_EDGE ( 'NONE', *, *, #34863, .T. ) ;
#10036=CARTESIAN_POINT ( 'NONE',  ( 74.69189222814998175, -41.76310523276723785, -6.393215200338315363 ) ) ;
#10049=CARTESIAN_POINT ( 'NONE',  ( 108.8851452545248151, 0.8980012041604421569, -11.00651665394454071 ) ) ;
#10050=CARTESIAN_POINT ( 'NONE',  ( 106.8710046295248759, -4.863998795839590272, -18.39754474579285315 ) ) ;
#10051=CARTESIAN_POINT ( 'NONE',  ( 87.44708369096657918, -23.44614552640564042, -8.393215200338314474 ) ) ;
#10060=CARTESIAN_POINT ( 'NONE',  ( 106.5931921295248372, 0.8980012041604618078, -13.39321520033831447 ) ) ;
#10068=CARTESIAN_POINT ( 'NONE',  ( 82.71771818927497577, -31.37104225293308701, -22.09381113811972597 ) ) ;
#10074=DIRECTION ( 'NONE',  ( 1.000000000000000000, 0.000000000000000000, 0.000000000000000000 ) ) ;
#10081=CARTESIAN_POINT ( 'NONE',  ( 109.9269421295247753, 0.8980012041604618078, -13.39321520033831447 ) ) ;
#10083=EDGE_LOOP ( 'NONE', ( #13664, #37109, #1456, #13469, #42028 ) ) ;
#10092=AXIS2_PLACEMENT_3D ( 'NONE', #33006, #1556, #33237 ) ;
#10099=VERTEX_POINT ( 'NONE', #21699 ) ;
#10102=CARTESIAN_POINT ( 'NONE',  ( 108.3295202545248657, -10.62599879583958717, -15.77991374673208469 ) ) ;
#10103=CARTESIAN_POINT ( 'NONE',  ( 115.0664733795247798, -1.325403438956436419, -9.854619843455211026 ) ) ;
#10104=CARTESIAN_POINT ( 'NONE',  ( 109.3713171295247832, -10.62599879583958540, -13.39321520033831447 ) ) ;
#10107=ORIENTED_EDGE ( 'NONE', *, *, #22836, .F. ) ;
#10109=CARTESIAN_POINT ( 'NONE',  ( 109.6491296295247793, -4.863998795839590272, -19.15521520033831493 ) ) ;
#10117=CARTESIAN_POINT ( 'NONE',  ( 114.0246765045248196, -2.791137627527939813, -8.388885654883777576 ) ) ;
#10118=ORIENTED_EDGE ( 'NONE', *, *, #33114, .T. ) ;
#10119=CARTESIAN_POINT ( 'NONE',  ( 61.69189222814998175, -64.41823023953081417, -19.25521411788945514 ) ) ;
#10122=CARTESIAN_POINT ( 'NONE',  ( 109.6491296295247793, -4.863998795839590272, -8.388885654883775800 ) ) ;
#10123=CARTESIAN_POINT ( 'NONE',  ( 108.8156921295247912, -9.868328341294093420, -13.39321520033831447 ) ) ;
#10141=CARTESIAN_POINT ( 'NONE',  ( 114.6497546295247929, -4.863998795839590272, -7.631215200338315796 ) ) ;
#10147=CARTESIAN_POINT ( 'NONE',  ( 116.5564130180080866, 0.7607806665037644134, -14.64321520033833401 ) ) ;
#10148=CARTESIAN_POINT ( 'NONE',  ( 112.9828796295247884, -4.863998795839590272, -19.15521520033831493 ) ) ;
#10150=FACE_OUTER_BOUND ( 'NONE', #12800, .T. ) ;
#10153=VECTOR ( 'NONE', #22268, 1000.000000000000000 ) ;
#10159=CARTESIAN_POINT ( 'NONE',  ( 107.7738952545248310, -9.868328341294098749, -15.46607636864997204 ) ) ;
#10163=CARTESIAN_POINT ( 'NONE',  ( 110.5520202545248054, 0.1403307496149616695, -11.32035403202665336 ) ) ;
#10164=CARTESIAN_POINT ( 'NONE',  ( 111.8021765045248372, -7.250697342233347165, -19.15521520033830427 ) ) ;
#10169=CARTESIAN_POINT ( 'NONE',  ( 109.6491296295247793, -4.863998795839590272, -19.15521520033831493 ) ) ;
#10172=CARTESIAN_POINT ( 'NONE',  ( 111.9664176093651804, 0.5600166689815611054, -14.64321520033831447 ) ) ;
#10176=ORIENTED_EDGE ( 'NONE', *, *, #4713, .T. ) ;
#10187=CARTESIAN_POINT ( 'NONE',  ( 116.8576166310760556, -0.4515803448876515303, -16.26233397272304870 ) ) ;
#10188=CARTESIAN_POINT ( 'NONE',  ( 113.8857702545248003, -10.62599879583958717, -15.77991374673208469 ) ) ;
#10190=DIRECTION ( 'NONE',  ( 0.000000000000000000, 0.000000000000000000, -1.000000000000000000 ) ) ;
#10197=CARTESIAN_POINT ( 'NONE',  ( 106.4542858795248179, -8.402594152722688392, -9.854619843455216355 ) ) ;
#10200=CARTESIAN_POINT ( 'NONE',  ( 69.91302804934421999, -34.85583393072344194, -5.893215200338315363 ) ) ;
#10201=CARTESIAN_POINT ( 'NONE',  ( 69.69189222814998175, -41.76310523276723785, -6.393215200338315363 ) ) ;
#10204=ORIENTED_EDGE ( 'NONE', *, *, #8323, .T. ) ;
#10210=CARTESIAN_POINT ( 'NONE',  ( 109.8574890045247940, 0.8980012041604421569, -15.77991374673208469 ) ) ;
#10212=CARTESIAN_POINT ( 'NONE',  ( 83.32261893989519308, -31.98912039979894573, -23.53030018102887055 ) ) ;
#10218=CARTESIAN_POINT ( 'NONE',  ( 108.2600671295247992, 0.1403307496149613920, -13.39321520033831447 ) ) ;
#10231=VECTOR ( 'NONE', #23995, 1000.000000000000000 ) ;
#10232=DIRECTION ( 'NONE',  ( -1.000000000000000000, 0.000000000000000000, 0.000000000000000000 ) ) ;
#10235=CARTESIAN_POINT ( 'NONE',  ( 115.8999108795247821, -8.938348069036489818, -9.318865927141430916 ) ) ;
#10238=ORIENTED_EDGE ( 'NONE', *, *, #36629, .F. ) ;
#10240=EDGE_CURVE ( 'NONE', #11904, #33939, #44391, .T. ) ;
#10243=ORIENTED_EDGE ( 'NONE', *, *, #5222, .F. ) ;
#10244=CARTESIAN_POINT ( 'NONE',  ( 114.4413952545248350, 0.8980012041604421569, -11.00651665394454071 ) ) ;
#10260=ORIENTED_EDGE ( 'NONE', *, *, #5598, .T. ) ;
#10262=CARTESIAN_POINT ( 'NONE',  ( 108.0517077545248696, -7.250697342233347165, -7.631215200338321125 ) ) ;
#10264=CARTESIAN_POINT ( 'NONE',  ( 106.3153796295248412, -4.863998795839590272, -8.388885654883775800 ) ) ;
#10265=CARTESIAN_POINT ( 'NONE',  ( 106.0375671295248310, 0.1403307496149613920, -13.39321520033831447 ) ) ;
#10266=DIRECTION ( 'NONE',  ( 0.000000000000000000, 0.000000000000000000, 1.000000000000000000 ) ) ;
#10275=CARTESIAN_POINT ( 'NONE',  ( 107.0793640045248196, -10.62599879583958717, -11.00651665394454604 ) ) ;
#10278=DIRECTION ( 'NONE',  ( 1.000000000000000000, 0.000000000000000000, 0.000000000000000000 ) ) ;
#10281=AXIS2_PLACEMENT_3D ( 'NONE', #35520, #28257, #7056 ) ;
#10289=DIRECTION ( 'NONE',  ( 0.000000000000000000, 0.000000000000000000, -1.000000000000000000 ) ) ;
#10299=EDGE_CURVE ( 'NONE', #38311, #574, #24959, .T. ) ;
#10301=CARTESIAN_POINT ( 'NONE',  ( 108.1211608795247798, -8.938348069036489818, -9.318865927141430916 ) ) ;
#10310=DIRECTION ( 'NONE',  ( 0.000000000000000000, 0.000000000000000000, 1.000000000000000000 ) ) ;
#10317=ORIENTED_EDGE ( 'NONE', *, *, #40402, .F. ) ;
#10320=CARTESIAN_POINT ( 'NONE',  ( 110.4131140045248287, -10.62599879583958717, -11.00651665394454604 ) ) ;
#10321=VECTOR ( 'NONE', #5256, 1000.000000000000227 ) ;
#10322=CARTESIAN_POINT ( 'NONE',  ( 108.2600671295247992, 0.1403307496149613920, -13.39321520033831447 ) ) ;
#10323=CARTESIAN_POINT ( 'NONE',  ( 105.6903015045248253, -2.477300249445798297, -7.631215200338321125 ) ) ;
#10328=CARTESIAN_POINT ( 'NONE',  ( 109.5102233795247884, -8.938348069036489818, -17.46756447353520159 ) ) ;
#10335=CARTESIAN_POINT ( 'NONE',  ( 107.0793640045248196, -10.62599879583958717, -11.00651665394454604 ) ) ;
#10340=CARTESIAN_POINT ( 'NONE',  ( 115.2748327545248657, -2.477300249445798297, -19.15521520033831138 ) ) ;
#10341=CARTESIAN_POINT ( 'NONE',  ( 105.4124890045248293, -9.868328341294098749, -11.32035403202665869 ) ) ;
#10358=DIRECTION ( 'NONE',  ( -1.000000000000000000, 0.000000000000000000, 0.000000000000000000 ) ) ;
#10360=ORIENTED_EDGE ( 'NONE', *, *, #295, .T. ) ;
#10363=CARTESIAN_POINT ( 'NONE',  ( 115.1359265045248605, -7.250697342233347165, -19.15521520033831138 ) ) ;
#10364=CARTESIAN_POINT ( 'NONE',  ( 115.3442858795247759, -8.402594152722736354, -9.854619843455244776 ) ) ;
#10368=ORIENTED_EDGE ( 'NONE', *, *, #43404, .T. ) ;
#10369=DIRECTION ( 'NONE',  ( -1.000000000000000000, 0.000000000000000000, 0.000000000000000000 ) ) ;
#10372=CARTESIAN_POINT ( 'NONE',  ( 67.69189222814998175, -55.76310523276723785, -40.89321520033831092 ) ) ;
#10378=CARTESIAN_POINT ( 'NONE',  ( 106.2459265045248173, -2.791137627527939813, -8.388885654883777576 ) ) ;
#10383=CARTESIAN_POINT ( 'NONE',  ( 109.5796765045248122, -2.791137627527939813, -8.388885654883777576 ) ) ;
#10384=AXIS2_PLACEMENT_3D ( 'NONE', #19366, #33708, #15952 ) ;
#10386=CARTESIAN_POINT ( 'NONE',  ( 109.2295573004754061, -4.817128553740947616, -18.58155556397246500 ) ) ;
#10388=CARTESIAN_POINT ( 'NONE',  ( 106.5237390045248418, 0.8980012041604421569, -15.77991374673208469 ) ) ;
#10389=CARTESIAN_POINT ( 'NONE',  ( 77.22947525540432423, -44.03086066871760096, -4.893215200338314474 ) ) ;
#10390=CARTESIAN_POINT ( 'NONE',  ( 109.0240515045248202, -2.477300249445798297, -7.631215200338321125 ) ) ;
#10397=ORIENTED_EDGE ( 'NONE', *, *, #3274, .F. ) ;
#10408=CARTESIAN_POINT ( 'NONE',  ( 116.8252617111891993, -1.616627641789968317, -17.49395584329565523 ) ) ;
#10409=CARTESIAN_POINT ( 'NONE',  ( 115.7610046295247912, -4.863998795839590272, -7.631215200338315796 ) ) ;
#10410=ORIENTED_EDGE ( 'NONE', *, *, #9789, .T. ) ;
#10415=VECTOR ( 'NONE', #27740, 1000.000000000000000 ) ;
#10421=CARTESIAN_POINT ( 'NONE',  ( 113.5385046295247804, -4.863998795839590272, -18.39754474579285315 ) ) ;
#10425=CARTESIAN_POINT ( 'NONE',  ( 109.2294421295247844, 0.8460904216231607267, -7.393215200338315363 ) ) ;
#10427=VERTEX_POINT ( 'NONE', #336 ) ;
#10434=CARTESIAN_POINT ( 'NONE',  ( 105.0652233795248378, -1.325403438956436419, -9.854619843455211026 ) ) ;
#10435=CARTESIAN_POINT ( 'NONE',  ( 111.5243640045248412, -10.62599879583958717, -11.00651665394454604 ) ) ;
#10442=CARTESIAN_POINT ( 'NONE',  ( 107.3571765045248299, -2.791137627527939813, -8.388885654883777576 ) ) ;
#10443=DIRECTION ( 'NONE',  ( 0.000000000000000000, 0.000000000000000000, -1.000000000000000000 ) ) ;
#10453=B_SPLINE_CURVE_WITH_KNOTS ( 'NONE', 3,
 ( #3673, #31708, #27863, #24217, #41773, #28533, #34451, #21458 ),
 .UNSPECIFIED., .F., .F.,
 ( 4, 2, 2, 4 ),
 ( 0.000000000000000000, 0.5000000000000000000, 0.7500000000000000000, 1.000000000000000000 ),
 .UNSPECIFIED. ) ;
#10457=CARTESIAN_POINT ( 'NONE',  ( 108.8156921295247912, -9.868328341294093420, -13.39321520033831447 ) ) ;
#10460=DIRECTION ( 'NONE',  ( 3.317300593186674996E-33, -1.668003342285379964E-16, -1.000000000000000000 ) ) ;
#10467=ORIENTED_EDGE ( 'NONE', *, *, #9273, .F. ) ;
#10468=CARTESIAN_POINT ( 'NONE',  ( 116.2471765045247594, -7.250697342233347165, -19.15521520033831138 ) ) ;
#10477=VECTOR ( 'NONE', #14003, 1000.000000000000000 ) ;
#10485=CARTESIAN_POINT ( 'NONE',  ( 115.8999108795247821, -1.325403438956436419, -16.93181055722141792 ) ) ;
#10497=CARTESIAN_POINT ( 'NONE',  ( 112.8439733795247832, -1.325403438956436419, -9.854619843455211026 ) ) ;
#10508=ORIENTED_EDGE ( 'NONE', *, *, #6734, .T. ) ;
#10509=CARTESIAN_POINT ( 'NONE',  ( 116.5955426422556940, -9.864956876375439165, -13.35547112582854190 ) ) ;
#10512=ORIENTED_EDGE ( 'NONE', *, *, #12568, .T. ) ;
#10516=CARTESIAN_POINT ( 'NONE',  ( 107.3571765045248299, -7.250697342233347165, -19.15521520033831138 ) ) ;
#10535=ORIENTED_EDGE ( 'NONE', *, *, #1621, .F. ) ;
#10536=CARTESIAN_POINT ( 'NONE',  ( 109.8574890045247940, 0.8980012041604421569, -15.77991374673208469 ) ) ;
#10537=CARTESIAN_POINT ( 'NONE',  ( 107.0793640045248196, 0.1403307496149616695, -15.46607636864997204 ) ) ;
#10538=CARTESIAN_POINT ( 'NONE',  ( 109.1629577545248395, -7.250697342233347165, -7.631215200338321125 ) ) ;
#10543=EDGE_CURVE ( 'NONE', #20305, #24500, #7983, .T. ) ;
#10545=CARTESIAN_POINT ( 'NONE',  ( 110.7603796295247918, -4.863998795839590272, -19.15521520033831493 ) ) ;
#10546=CARTESIAN_POINT ( 'NONE',  ( 61.69189222814998175, -39.81387020377190566, -6.644606968976401795 ) ) ;
#10549=EDGE_CURVE ( 'NONE', #11473, #37481, #18125, .T. ) ;
#10550=FACE_BOUND ( 'NONE', #15336, .T. ) ;
#10553=CARTESIAN_POINT ( 'NONE',  ( 116.1082702545247827, -10.62599879583958717, -15.77991374673208469 ) ) ;
#10554=CARTESIAN_POINT ( 'NONE',  ( 106.0375671295248310, -10.62599879583958540, -13.39321520033831447 ) ) ;
#10560=CARTESIAN_POINT ( 'NONE',  ( 114.0246765045248196, -7.250697342233347165, -19.15521520033831138 ) ) ;
#10561=CARTESIAN_POINT ( 'NONE',  ( 107.9822546295247889, -4.863998795839590272, -18.39754474579285315 ) ) ;
#10571=ORIENTED_EDGE ( 'NONE', *, *, #20585, .T. ) ;
#10573=CARTESIAN_POINT ( 'NONE',  ( 110.0658483795247804, -8.402594152722688392, -16.93181055722141792 ) ) ;
#10575=ORIENTED_EDGE ( 'NONE', *, *, #4937, .T. ) ;
#10585=CARTESIAN_POINT ( 'NONE',  ( 106.8710046295248759, -4.863998795839590272, -18.39754474579285315 ) ) ;
#10591=CARTESIAN_POINT ( 'NONE',  ( 116.7121013948518140, -7.018196182899982816, -18.03571476200153967 ) ) ;
#10597=ORIENTED_EDGE ( 'NONE', *, *, #35586, .F. ) ;
#10600=CARTESIAN_POINT ( 'NONE',  ( 110.2742077545248094, -7.250697342233347165, -7.631215200338321125 ) ) ;
#10606=CARTESIAN_POINT ( 'NONE',  ( 108.0517077545248696, -2.791137627527939813, -18.39754474579286025 ) ) ;
#10608=CARTESIAN_POINT ( 'NONE',  ( 109.2294667191664530, -5.158692816978520668, -18.58770334803330115 ) ) ;
#10611=CARTESIAN_POINT ( 'NONE',  ( 116.3860827545247787, -6.936859964151250502, -8.388885654883777576 ) ) ;
#10612=CARTESIAN_POINT ( 'NONE',  ( 110.0658483795247804, -0.7896495226426338832, -9.318865927141430916 ) ) ;
#10629=CARTESIAN_POINT ( 'NONE',  ( 112.4967077545247633, -7.250697342233347165, -7.631215200338321125 ) ) ;
#10632=CARTESIAN_POINT ( 'NONE',  ( 78.69189222814998175, -41.90950876995110974, -19.14091845747265808 ) ) ;
#10640=CARTESIAN_POINT ( 'NONE',  ( 116.1082702545247827, 0.1403307496149616695, -11.32035403202665336 ) ) ;
#10642=LINE ( 'NONE', #19497, #12210 ) ;
#10647=ORIENTED_EDGE ( 'NONE', *, *, #39550, .T. ) ;
#10650=CARTESIAN_POINT ( 'NONE',  ( 115.4831921295247952, -9.868328341294093420, -13.39321520033831447 ) ) ;
#10653=CARTESIAN_POINT ( 'NONE',  ( 106.6626452545248611, -9.868328341294098749, -15.46607636864997204 ) ) ;
#10654=CARTESIAN_POINT ( 'NONE',  ( 111.8716296295247901, -4.863998795839590272, -19.15521520033831493 ) ) ;
#10660=CARTESIAN_POINT ( 'NONE',  ( 109.2294540793403712, -5.090843144855284663, -7.811289275559451184 ) ) ;
#10662=CARTESIAN_POINT ( 'NONE',  ( 111.0381921295247878, -9.868328341294093420, -13.39321520033831447 ) ) ;
#10664=PRODUCT ( 'Main Bracket', 'Main Bracket', '', ( #32741 ) ) ;
#10668=CARTESIAN_POINT ( 'NONE',  ( 112.3578015045248861, -2.477300249445798297, -7.631215200338321125 ) ) ;
#10679=CARTESIAN_POINT ( 'NONE',  ( 107.8433483795247838, -8.402594152722688392, -16.93181055722141792 ) ) ;
#10681=CARTESIAN_POINT ( 'NONE',  ( 85.31664890835789095, -21.99489077589589314, -11.39321520033831447 ) ) ;
#10684=AXIS2_PLACEMENT_3D ( 'NONE', #44910, #5903, #6372 ) ;
#10687=VERTEX_POINT ( 'NONE', #30828 ) ;
#10688=CARTESIAN_POINT ( 'NONE',  ( 106.9404577545248145, -2.791137627527939813, -18.39754474579286025 ) ) ;
#10692=FACE_OUTER_BOUND ( 'NONE', #15949, .T. ) ;
#10697=AXIS2_PLACEMENT_3D ( 'NONE', #30566, #44268, #10278 ) ;
#10705=CARTESIAN_POINT ( 'NONE',  ( 109.0240515045248202, -2.477300249445798297, -7.631215200338321125 ) ) ;
#10717=AXIS2_PLACEMENT_3D ( 'NONE', #11583, #40296, #22290 ) ;
#10719=CARTESIAN_POINT ( 'NONE',  ( 111.3854577545248645, -2.791137627527939813, -18.39754474579286025 ) ) ;
#10727=DIRECTION ( 'NONE',  ( 1.000000000000000000, 0.000000000000000000, 0.000000000000000000 ) ) ;
#10732=CARTESIAN_POINT ( 'NONE',  ( 62.77916120947350720, -64.70587450232225990, -45.96270195078128751 ) ) ;
#10734=VERTEX_POINT ( 'NONE', #31931 ) ;
#10735=CARTESIAN_POINT ( 'NONE',  ( 107.2294421295247844, -9.051693226400931991, -21.89321520033831447 ) ) ;
#10741=CARTESIAN_POINT ( 'NONE',  ( 105.9681140045248355, -10.62599879583958717, -11.00651665394454604 ) ) ;
#10743=ORIENTED_EDGE ( 'NONE', *, *, #3535, .T. ) ;
#10744=ORIENTED_EDGE ( 'NONE', *, *, #24000, .T. ) ;
#10749=CARTESIAN_POINT ( 'NONE',  ( 109.2294421295247844, -11.83367149576868727, -19.39321520033831447 ) ) ;
#10751=LINE ( 'NONE', #34231, #42983 ) ;
#10752=PLANE ( 'NONE',  #26653 ) ;
#10761=CARTESIAN_POINT ( 'NONE',  ( 105.4819421295248247, 0.8980012041604618078, -13.39321520033831447 ) ) ;
#10762=CARTESIAN_POINT ( 'NONE',  ( 110.6214733795247867, -1.325403438956436419, -9.854619843455211026 ) ) ;
#10763=CARTESIAN_POINT ( 'NONE',  ( 114.3024890045248156, -9.868328341294098749, -11.32035403202665869 ) ) ;
#10769=CARTESIAN_POINT ( 'NONE',  ( 111.9410827545248708, -2.477300249445798297, -19.15521520033831138 ) ) ;
#10775=CARTESIAN_POINT ( 'NONE',  ( 113.3301452545248083, 0.8980012041604421569, -11.00651665394454071 ) ) ;
#10776=CARTESIAN_POINT ( 'NONE',  ( 114.5803015045248117, -6.936859964151250502, -18.39754474579286025 ) ) ;
#10777=ORIENTED_EDGE ( 'NONE', *, *, #22060, .T. ) ;
#10781=CARTESIAN_POINT ( 'NONE',  ( 114.9275671295247889, -10.62599879583958540, -13.39321520033831447 ) ) ;
#10782=CARTESIAN_POINT ( 'NONE',  ( 106.4542858795248179, -8.402594152722688392, -9.854619843455216355 ) ) ;
#10786=ORIENTED_EDGE ( 'NONE', *, *, #29187, .T. ) ;
#10788=DIRECTION ( 'NONE',  ( 0.000000000000000000, 0.000000000000000000, -1.000000000000000000 ) ) ;
#10790=ORIENTED_EDGE ( 'NONE', *, *, #10549, .T. ) ;
#10792=CARTESIAN_POINT ( 'NONE',  ( 106.1764733795248219, -8.938348069036489818, -17.46756447353520159 ) ) ;
#10793=CARTESIAN_POINT ( 'NONE',  ( 108.4684265045247997, -2.791137627527939813, -8.388885654883777576 ) ) ;
#10794=EDGE_LOOP ( 'NONE', ( #21013, #1240, #9167, #3267 ) ) ;
#10803=DIRECTION ( 'NONE',  ( 0.000000000000000000, 0.6161630946014892141, 0.7876185884367612466 ) ) ;
#10804=CARTESIAN_POINT ( 'NONE',  ( 114.5803015045248117, -2.477300249445798297, -7.631215200338321125 ) ) ;
#10812=CARTESIAN_POINT ( 'NONE',  ( 115.4831921295247952, 0.8980012041604618078, -13.39321520033831447 ) ) ;
#10819=CARTESIAN_POINT ( 'NONE',  ( 109.7880358795247986, -0.7896495226426338832, -17.46756447353520159 ) ) ;
#10824=CARTESIAN_POINT ( 'NONE',  ( 109.3018640045248304, 0.1403307496149616695, -15.46607636864997204 ) ) ;
#10828=CARTESIAN_POINT ( 'NONE',  ( 109.2296389617769989, -8.690306221987864177, -17.17721600569922558 ) ) ;
#10830=CARTESIAN_POINT ( 'NONE',  ( 106.8710046295248759, -4.863998795839590272, -7.631215200338315796 ) ) ;
#10832=CARTESIAN_POINT ( 'NONE',  ( 107.5655358795247736, -0.7896495226426338832, -17.46756447353520159 ) ) ;
#10839=EDGE_LOOP ( 'NONE', ( #41284, #4388 ) ) ;
#10850=CARTESIAN_POINT ( 'NONE',  ( 110.1353015045248469, -2.477300249445798297, -7.631215200338321125 ) ) ;
#10852=EDGE_CURVE ( 'NONE', #24453, #20884, #20793, .T. ) ;
#10853=EDGE_CURVE ( 'NONE', #40056, #37700, #10453, .T. ) ;
#10854=CARTESIAN_POINT ( 'NONE',  ( 61.58853448128274266, 6.499901296646661386, -14.64321520033831447 ) ) ;
#10856=CARTESIAN_POINT ( 'NONE',  ( 116.8722546295247895, -4.863998795839590272, -18.39754474579285315 ) ) ;
#10861=CARTESIAN_POINT ( 'NONE',  ( 111.2695311052981708, 0.4930828106259610433, -12.14321520033830026 ) ) ;
#10863=CARTESIAN_POINT ( 'NONE',  ( 113.4690515045247992, -6.936859964151250502, -18.39754474579286025 ) ) ;
#10867=DIRECTION ( 'NONE',  ( 0.000000000000000000, -0.9284778069183718952, -0.3713878862591650232 ) ) ;
#10874=CARTESIAN_POINT ( 'NONE',  ( 115.1359265045248605, -2.791137627527939813, -8.388885654883777576 ) ) ;
#10877=CARTESIAN_POINT ( 'NONE',  ( 85.90559391046389237, -27.46290284877522936, -8.672333233500294725 ) ) ;
#10878=CARTESIAN_POINT ( 'NONE',  ( 111.9410827545248708, -2.477300249445798297, -19.15521520033831138 ) ) ;
#10882=CARTESIAN_POINT ( 'NONE',  ( 109.2294421509997591, -4.671552374252124551, -7.823865419768949891 ) ) ;
#10884=CARTESIAN_POINT ( 'NONE',  ( 110.5520202545248054, 0.1403307496149616695, -11.32035403202665336 ) ) ;
#10885=CARTESIAN_POINT ( 'NONE',  ( 116.8295036813193946, 1.973147266281264578, -20.94028373511954655 ) ) ;
#10888=CARTESIAN_POINT ( 'NONE',  ( 110.2047546295247855, -4.863998795839590272, -7.631215200338315796 ) ) ;
#10900=CARTESIAN_POINT ( 'NONE',  ( 113.5385046295247804, -4.863998795839590272, -7.631215200338315796 ) ) ;
#10908=CARTESIAN_POINT ( 'NONE',  ( 115.2053796295247849, -4.863998795839590272, -19.15521520033831493 ) ) ;
#10910=DIRECTION ( 'NONE',  ( 0.000000000000000000, 0.000000000000000000, -1.000000000000000000 ) ) ;
#10915=DIRECTION ( 'NONE',  ( 0.000000000000000000, 0.000000000000000000, 1.000000000000000000 ) ) ;
#10917=AXIS2_PLACEMENT_3D ( 'NONE', #2454, #19343, #27091 ) ;
#10926=CARTESIAN_POINT ( 'NONE',  ( 112.3578015045248861, -6.936859964151250502, -18.39754474579286025 ) ) ;
#10929=DIRECTION ( 'NONE',  ( 1.000000000000000000, 0.000000000000000000, 0.000000000000000000 ) ) ;
#10937=CARTESIAN_POINT ( 'NONE',  ( 112.5661608795247872, -1.325403438956436419, -16.93181055722141792 ) ) ;
#10948=DIRECTION ( 'NONE',  ( 0.000000000000000000, 0.000000000000000000, -1.000000000000000000 ) ) ;
#10952=EDGE_CURVE ( 'NONE', #7998, #40668, #38564, .T. ) ;
#10959=CARTESIAN_POINT ( 'NONE',  ( 107.6349890045248401, 0.8980012041604421569, -15.77991374673208469 ) ) ;
#10965=DIRECTION ( 'NONE',  ( 0.000000000000000000, -1.000000000000000000, 0.000000000000000000 ) ) ;
#10971=CARTESIAN_POINT ( 'NONE',  ( 61.69189222814998175, -49.76310523276723785, -7.393215200338315363 ) ) ;
#10981=CARTESIAN_POINT ( 'NONE',  ( 113.9552233795247815, -1.325403438956436419, -9.854619843455211026 ) ) ;
#10982=CARTESIAN_POINT ( 'NONE',  ( 106.7320983795247855, -8.402594152722688392, -16.93181055722141792 ) ) ;
#10983=CARTESIAN_POINT ( 'NONE',  ( 115.3442858795247759, -8.402594152722688392, -9.854619843455216355 ) ) ;
#10990=CARTESIAN_POINT ( 'NONE',  ( 111.2465515045248168, -2.477300249445798297, -7.631215200338321125 ) ) ;
#10997=CARTESIAN_POINT ( 'NONE',  ( 115.0664733795247798, -8.938348069036489818, -17.46756447353520159 ) ) ;
#10998=CARTESIAN_POINT ( 'NONE',  ( 111.4549108795247747, -1.325403438956436419, -16.93181055722141792 ) ) ;
#11004=CARTESIAN_POINT ( 'NONE',  ( 108.6767858795247861, -8.402594152722688392, -9.854619843455216355 ) ) ;
#11015=CARTESIAN_POINT ( 'NONE',  ( 106.4542858795248179, -0.7896495226426338832, -17.46756447353520159 ) ) ;
#11016=CARTESIAN_POINT ( 'NONE',  ( 109.8574890045247940, -9.868328341294098749, -11.32035403202665869 ) ) ;
#11027=DIRECTION ( 'NONE',  ( -1.000000000000000000, 0.000000000000000000, 0.000000000000000000 ) ) ;
#11028=CARTESIAN_POINT ( 'NONE',  ( 109.0935046295247872, -4.863998795839590272, -7.631215200338315796 ) ) ;
#11036=CARTESIAN_POINT ( 'NONE',  ( 115.7610046295247912, -4.863998795839590272, -7.631215200338315796 ) ) ;
#11037=CARTESIAN_POINT ( 'NONE',  ( 115.3442858795247759, -0.7896495226426338832, -17.46756447353520159 ) ) ;
#11041=LINE ( 'NONE', #28150, #37069 ) ;
#11042=CARTESIAN_POINT ( 'NONE',  ( 111.5243640045248412, -10.62599879583958717, -11.00651665394454604 ) ) ;
#11047=CARTESIAN_POINT ( 'NONE',  ( 111.8021765045248372, -2.791137627527939813, -8.388885654883777576 ) ) ;
#11050=CARTESIAN_POINT ( 'NONE',  ( 109.2294778858186390, -2.837229698210430140, -18.06364092945466382 ) ) ;
#11054=CARTESIAN_POINT ( 'NONE',  ( 114.7886608795247696, -1.325403438956436419, -16.93181055722141792 ) ) ;
#11055=CARTESIAN_POINT ( 'NONE',  ( 110.2047546295247855, -4.863998795839590272, -7.631215200338315796 ) ) ;
#11062=ORIENTED_EDGE ( 'NONE', *, *, #44306, .F. ) ;
#11071=CARTESIAN_POINT ( 'NONE',  ( 109.8574890045247940, 0.8980012041604421569, -15.77991374673208469 ) ) ;
#11076=CARTESIAN_POINT ( 'NONE',  ( 116.0388171295248014, 0.1403307496149613920, -13.39321520033831447 ) ) ;
#11078=CARTESIAN_POINT ( 'NONE',  ( 117.1872882340475996, 1.416175236645604851, -5.259658493298883464 ) ) ;
#11081=CARTESIAN_POINT ( 'NONE',  ( 111.2212166496844787, 0.5600166689815611054, -12.14321520033830026 ) ) ;
#11083=CARTESIAN_POINT ( 'NONE',  ( 114.2330358795247776, -8.402594152722688392, -9.854619843455216355 ) ) ;
#11085=ADVANCED_FACE ( 'NONE', ( #8226 ), #21903, .T. ) ;
#11088=LINE ( 'NONE', #3349, #28742 ) ;
#11096=CARTESIAN_POINT ( 'NONE',  ( 115.7610046295247912, -4.863998795839590272, -18.39754474579285315 ) ) ;
#11099=CARTESIAN_POINT ( 'NONE',  ( 85.99639782577784786, -27.24303960391588220, -8.592445736787643895 ) ) ;
#11100=CARTESIAN_POINT ( 'NONE',  ( 113.9552233795247815, -8.938348069036489818, -17.46756447353520159 ) ) ;
#11104=CARTESIAN_POINT ( 'NONE',  ( 109.2294582674637269, -1.259376031108396354, -9.372254076597803518 ) ) ;
#11106=CARTESIAN_POINT ( 'NONE',  ( 113.5385046295247804, -4.863998795839590272, -7.631215200338315796 ) ) ;
#11108=CARTESIAN_POINT ( 'NONE',  ( 83.86216108596053687, -31.76310523276723430, -22.89321520033831803 ) ) ;
#11111=CARTESIAN_POINT ( 'NONE',  ( 112.6356140045247827, -10.62599879583958717, -11.00651665394454604 ) ) ;
#11123=CARTESIAN_POINT ( 'NONE',  ( 113.7468640045248236, -10.62599879583958717, -11.00651665394454604 ) ) ;
#11126=DIRECTION ( 'NONE',  ( -1.000000000000000000, 0.000000000000000000, 0.000000000000000000 ) ) ;
#11127=VERTEX_POINT ( 'NONE', #24227 ) ;
#11131=ORIENTED_EDGE ( 'NONE', *, *, #41046, .F. ) ;
#11132=CARTESIAN_POINT ( 'NONE',  ( 115.7610046295247912, -4.863998795839590272, -7.631215200338315796 ) ) ;
#11136=CARTESIAN_POINT ( 'NONE',  ( 65.34289968162609341, -37.75951406093616214, -4.893215200338314474 ) ) ;
#11152=CARTESIAN_POINT ( 'NONE',  ( 115.4831921295247952, -9.868328341294093420, -13.39321520033831447 ) ) ;
#11155=CARTESIAN_POINT ( 'NONE',  ( 114.4413952545248350, -9.868328341294102302, -15.46607636865002355 ) ) ;
#11165=CARTESIAN_POINT ( 'NONE',  ( 111.1770983795247787, -8.402594152722688392, -16.93181055722141792 ) ) ;
#11173=CARTESIAN_POINT ( 'NONE',  ( 68.68839935636917460, -25.95913848132418522, -5.893215200338315363 ) ) ;
#11182=CARTESIAN_POINT ( 'NONE',  ( 115.5526452545247622, -9.868328341294098749, -15.46607636864997204 ) ) ;
#11185=ORIENTED_EDGE ( 'NONE', *, *, #26323, .T. ) ;
#11191=ORIENTED_EDGE ( 'NONE', *, *, #14710, .T. ) ;
#11193=CARTESIAN_POINT ( 'NONE',  ( 117.2294421295247844, 1.035107641088057973, -5.059859068394715109 ) ) ;
#11210=CARTESIAN_POINT ( 'NONE',  ( 115.0664733795247798, -8.938348069036489818, -17.46756447353520159 ) ) ;
#11211=CARTESIAN_POINT ( 'NONE',  ( 113.8857702545248003, 0.1403307496149616695, -11.32035403202665336 ) ) ;
#11212=CARTESIAN_POINT ( 'NONE',  ( 112.1494421295248003, -9.868328341294093420, -13.39321520033831447 ) ) ;
#11215=ORIENTED_EDGE ( 'NONE', *, *, #3272, .T. ) ;
#11217=CARTESIAN_POINT ( 'NONE',  ( 107.1488171295247867, -10.62599879583958540, -13.39321520033831447 ) ) ;
#11223=CARTESIAN_POINT ( 'NONE',  ( 113.4690515045247992, -2.477300249445798297, -7.631215200338321125 ) ) ;
#11224=CARTESIAN_POINT ( 'NONE',  ( 113.1912390045248031, -9.868328341294098749, -11.32035403202665869 ) ) ;
#11226=LINE ( 'NONE', #25133, #39827 ) ;
#11229=FACE_OUTER_BOUND ( 'NONE', #17341, .T. ) ;
#11239=DIRECTION ( 'NONE',  ( -0.9659258262890692004, -0.2588190451025175753, -8.979589471384751973E-16 ) ) ;
#11241=CARTESIAN_POINT ( 'NONE',  ( 115.8999108795247821, -8.938348069036489818, -9.318865927141430916 ) ) ;
#11243=ORIENTED_EDGE ( 'NONE', *, *, #12602, .F. ) ;
#11252=CARTESIAN_POINT ( 'NONE',  ( 111.1076452545248259, 0.8980012041604421569, -11.00651665394454071 ) ) ;
#11261=CARTESIAN_POINT ( 'NONE',  ( 115.6915515045247531, -2.477300249445798297, -7.631215200338321125 ) ) ;
#11262=CARTESIAN_POINT ( 'NONE',  ( 64.43740640915127926, -35.20632691772231482, -5.871463680831255694 ) ) ;
#11267=CARTESIAN_POINT ( 'NONE',  ( 109.6052378519203927, 0.2518737723193609224, -12.14321520033833757 ) ) ;
#11268=CARTESIAN_POINT ( 'NONE',  ( 112.7050671295247923, -10.62599879583958540, -13.39321520033831447 ) ) ;
#11275=CARTESIAN_POINT ( 'NONE',  ( 115.8999108795247821, -8.938348069036489818, -9.318865927141430916 ) ) ;
#11276=CARTESIAN_POINT ( 'NONE',  ( 109.2294308679984596, -7.595023145029839995, -17.96264590402594763 ) ) ;
#11280=CARTESIAN_POINT ( 'NONE',  ( 117.1500671295247713, 0.1403307496149613920, -13.39321520033831447 ) ) ;
#11281=CARTESIAN_POINT ( 'NONE',  ( 114.0246765045248196, -2.791137627527939813, -8.388885654883777576 ) ) ;
#11296=CARTESIAN_POINT ( 'NONE',  ( 111.1076452545248259, 0.8980012041604421569, -11.00651665394454071 ) ) ;
#11297=AXIS2_PLACEMENT_3D ( 'NONE', #45072, #30712, #806 ) ;
#11298=CARTESIAN_POINT ( 'NONE',  ( 116.0070878430555723, -11.05288298065394059, -20.89321520033831447 ) ) ;
#11300=CARTESIAN_POINT ( 'NONE',  ( 112.0799890045248475, -9.868328341294098749, -11.32035403202665869 ) ) ;
#11306=CARTESIAN_POINT ( 'NONE',  ( 110.2742077545248094, -2.791137627527939813, -18.39754474579286025 ) ) ;
#11318=CARTESIAN_POINT ( 'NONE',  ( 116.2471765045247594, -2.791137627527939813, -8.388885654883777576 ) ) ;
#11322=CARTESIAN_POINT ( 'NONE',  ( 112.4272546295247821, -4.863998795839590272, -7.631215200338315796 ) ) ;
#11327=CARTESIAN_POINT ( 'NONE',  ( 109.2294421295831768, -1.052844768949616094, -9.585856251807371109 ) ) ;
#11329=CARTESIAN_POINT ( 'NONE',  ( 106.6626452545248611, -9.868328341294098749, -15.46607636864997204 ) ) ;
#11330=CARTESIAN_POINT ( 'NONE',  ( 116.9575464499618676, 1.831790677941273149, -21.12945952840510344 ) ) ;
#11331=CARTESIAN_POINT ( 'NONE',  ( 83.85919441564438159, -31.77118883039085162, -23.13280229721742742 ) ) ;
#11334=CARTESIAN_POINT ( 'NONE',  ( 112.0105358795247810, -0.7896495226426338832, -17.46756447353520159 ) ) ;
#11337=DIRECTION ( 'NONE',  ( 0.000000000000000000, 1.000000000000000000, 0.000000000000000000 ) ) ;
#11344=CARTESIAN_POINT ( 'NONE',  ( 114.0941296295247867, -4.863998795839590272, -19.15521520033831493 ) ) ;
#11348=DIRECTION ( 'NONE',  ( 0.000000000000000000, 0.000000000000000000, -1.000000000000000000 ) ) ;
#11357=CARTESIAN_POINT ( 'NONE',  ( 70.36267391504962632, -5.685877709920933221, -4.893215200338314474 ) ) ;
#11360=CARTESIAN_POINT ( 'NONE',  ( 77.39250032628930853, -56.65331561251068848, -1.789128725675272369 ) ) ;
#11365=DIRECTION ( 'NONE',  ( 0.000000000000000000, 0.000000000000000000, -1.000000000000000000 ) ) ;
#11378=CARTESIAN_POINT ( 'NONE',  ( 114.5108483795247878, -8.402594152722688392, -16.93181055722141792 ) ) ;
#11379=CARTESIAN_POINT ( 'NONE',  ( 114.5803015045248259, -6.936859964151197211, -18.39754474579287447 ) ) ;
#11383=APPLICATION_CONTEXT ( 'automotive_design' ) ;
#11388=CARTESIAN_POINT ( 'NONE',  ( 107.1488171295248861, 0.1403307496149613920, -13.39321520033831447 ) ) ;
#11391=ORIENTED_EDGE ( 'NONE', *, *, #2358, .F. ) ;
#11394=CARTESIAN_POINT ( 'NONE',  ( 79.05243529145373316, 4.793396140045460108, -21.04957699274893557 ) ) ;
#11402=EDGE_CURVE ( 'NONE', #42526, #30491, #3398, .T. ) ;
#11406=EDGE_CURVE ( 'NONE', #14403, #38773, #38590, .T. ) ;
#11407=CARTESIAN_POINT ( 'NONE',  ( 115.9693640045247776, 0.1403307496149616695, -15.46607636864997204 ) ) ;
#11413=CARTESIAN_POINT ( 'NONE',  ( 105.5513952545248060, 0.8980012041604421569, -11.00651665394454071 ) ) ;
#11417=PLANE ( 'NONE',  #88 ) ;
#11419=CARTESIAN_POINT ( 'NONE',  ( 117.2294421295247844, 0.2335149919452661482, -21.89321520033831447 ) ) ;
#11426=CARTESIAN_POINT ( 'NONE',  ( 77.77634386988383142, 3.254514819260860392, -21.89321520033831447 ) ) ;
#11434=ORIENTED_EDGE ( 'NONE', *, *, #22836, .T. ) ;
#11438=CARTESIAN_POINT ( 'NONE',  ( 106.1070202545248407, -10.62599879583958717, -15.77991374673208469 ) ) ;
#11439=CARTESIAN_POINT ( 'NONE',  ( 111.4549108795247747, -1.325403438956436419, -16.93181055722141792 ) ) ;
#11444=CARTESIAN_POINT ( 'NONE',  ( 117.2294421295247844, 1.035107641088057973, -14.64321520033831447 ) ) ;
#11451=CARTESIAN_POINT ( 'NONE',  ( 112.4272546295247821, -4.863998795839590272, -18.39754474579285315 ) ) ;
#11463=AXIS2_PLACEMENT_3D ( 'NONE', #19545, #33423, #16128 ) ;
#11465=CARTESIAN_POINT ( 'NONE',  ( 113.7722331777918896, -0.01829820670813664396, -14.64321520033831447 ) ) ;
#11471=CARTESIAN_POINT ( 'NONE',  ( 108.0517077545248696, -2.791137627527939813, -18.39754474579286025 ) ) ;
#11473=VERTEX_POINT ( 'NONE', #24172 ) ;
#11479=VERTEX_POINT ( 'NONE', #7494 ) ;
#11482=CARTESIAN_POINT ( 'NONE',  ( 113.1217858795247935, -0.7896495226426338832, -17.46756447353520159 ) ) ;
#11492=CARTESIAN_POINT ( 'NONE',  ( 115.2748327545248657, -2.477300249445798297, -19.15521520033831138 ) ) ;
#11494=ORIENTED_EDGE ( 'NONE', *, *, #38212, .T. ) ;
#11496=CARTESIAN_POINT ( 'NONE',  ( 62.29163388691242886, -36.90296252317118331, -5.462008551790970223 ) ) ;
#11497=CARTESIAN_POINT ( 'NONE',  ( 112.0105358795247810, -0.7896495226426338832, -17.46756447353520159 ) ) ;
#11502=CARTESIAN_POINT ( 'NONE',  ( 111.6869545411902465, -0.3595008806742185925, -10.82052240173743130 ) ) ;
#11505=CARTESIAN_POINT ( 'NONE',  ( 115.5732721536726899, 0.3967854368540359999, -10.50530088663808925 ) ) ;
#11506=CARTESIAN_POINT ( 'NONE',  ( 109.2295713675052298, -10.43732579977344699, -13.23368918432362484 ) ) ;
#11509=CARTESIAN_POINT ( 'NONE',  ( 115.8304577545247582, -2.791137627527939813, -18.39754474579286025 ) ) ;
#11510=CARTESIAN_POINT ( 'NONE',  ( 115.1359265045248605, -2.791137627527939813, -8.388885654883777576 ) ) ;
#11513=CARTESIAN_POINT ( 'NONE',  ( 143.3676850761856940, -49.76310523276723785, -40.89321520033831092 ) ) ;
#11522=EDGE_LOOP ( 'NONE', ( #39728, #35352, #42419, #23312 ) ) ;
#11526=CARTESIAN_POINT ( 'NONE',  ( 110.8992858795247827, -0.7896495226426338832, -17.46756447353520159 ) ) ;
#11527=DIRECTION ( 'NONE',  ( 0.000000000000000000, 0.000000000000000000, -1.000000000000000000 ) ) ;
#11529=CARTESIAN_POINT ( 'NONE',  ( 114.6497546295247929, -4.863998795839590272, -18.39754474579285315 ) ) ;
#11531=ADVANCED_FACE ( 'NONE', ( #3626 ), #21186, .F. ) ;
#11532=PLANE ( 'NONE',  #4769 ) ;
#11536=CARTESIAN_POINT ( 'NONE',  ( 108.6767858795247861, -8.402594152722688392, -9.854619843455216355 ) ) ;
#11547=CARTESIAN_POINT ( 'NONE',  ( 112.7745202545247878, 0.1403307496149616695, -11.32035403202665336 ) ) ;
#11550=CARTESIAN_POINT ( 'NONE',  ( 86.31085725162986932, -26.48153815035164627, -8.422460282204015769 ) ) ;
#11551=CARTESIAN_POINT ( 'NONE',  ( 109.4407702545248355, -10.62599879583958717, -15.77991374673208469 ) ) ;
#11558=CARTESIAN_POINT ( 'NONE',  ( 115.6915515045247531, -2.477300249445798297, -7.631215200338321125 ) ) ;
#11559=CARTESIAN_POINT ( 'NONE',  ( 116.8677062910727074, 1.935364965237992285, -20.99533717236457164 ) ) ;
#11560=CARTESIAN_POINT ( 'NONE',  ( 83.96184352754465863, -31.49149003370463262, -22.09312770924474734 ) ) ;
#11563=CARTESIAN_POINT ( 'NONE',  ( 109.5102233795247884, -8.938348069036489818, -17.46756447353520159 ) ) ;
#11572=CARTESIAN_POINT ( 'NONE',  ( 113.8163171295247764, -10.62599879583958540, -13.39321520033831447 ) ) ;
#11573=CIRCLE ( 'NONE', #35563, 1.999999999999997558 ) ;
#11581=CARTESIAN_POINT ( 'NONE',  ( 74.69189222814998175, -41.76310523276723785, -20.39321520033831447 ) ) ;
#11583=CARTESIAN_POINT ( 'NONE',  ( 72.87572422742091760, -11.86958442233774313, -21.89321520033831447 ) ) ;
#11599=CARTESIAN_POINT ( 'NONE',  ( 113.1217858795247935, -8.402594152722688392, -9.854619843455216355 ) ) ;
#11600=CARTESIAN_POINT ( 'NONE',  ( 82.45431455551781141, -31.76310523276724140, -22.91043087769159214 ) ) ;
#11603=CARTESIAN_POINT ( 'NONE',  ( 116.1777233795247781, -1.325403438956436419, -9.854619843455211026 ) ) ;
#11605=VECTOR ( 'NONE', #37728, 1000.000000000000000 ) ;
#11610=CARTESIAN_POINT ( 'NONE',  ( 108.3989733795248753, -1.325403438956436419, -9.854619843455211026 ) ) ;
#11621=EDGE_CURVE ( 'NONE', #12207, #18915, #4368, .T. ) ;
#11622=CARTESIAN_POINT ( 'NONE',  ( 116.6638952545248031, -9.868328341294098749, -15.46607636864997204 ) ) ;
#11628=CARTESIAN_POINT ( 'NONE',  ( 110.6909265045248247, -2.791137627527939813, -8.388885654883745602 ) ) ;
#11630=VERTEX_POINT ( 'NONE', #654 ) ;
#11635=CARTESIAN_POINT ( 'NONE',  ( 64.61650192636965073, -34.86087584742114132, -0.8932152003383146965 ) ) ;
#11651=CARTESIAN_POINT ( 'NONE',  ( 114.7905291257774820, 0.2334052082820642360, -12.14321520033831625 ) ) ;
#11653=FACE_OUTER_BOUND ( 'NONE', #18797, .T. ) ;
#11654=CARTESIAN_POINT ( 'NONE',  ( 115.8999108795247821, -1.325403438956436419, -16.93181055722141792 ) ) ;
#11655=CARTESIAN_POINT ( 'NONE',  ( 115.2748327545248657, -6.936859964151250502, -8.388885654883777576 ) ) ;
#11667=CARTESIAN_POINT ( 'NONE',  ( 110.6214733795247867, -8.938348069036489818, -17.46756447353520159 ) ) ;
#11668=CARTESIAN_POINT ( 'NONE',  ( 111.7327233795247849, -1.325403438956436419, -9.854619843455211026 ) ) ;
#11680=EDGE_CURVE ( 'NONE', #30574, #28223, #36276, .T. ) ;
#11682=AXIS2_PLACEMENT_3D ( 'NONE', #8466, #8012, #21919 ) ;
#11688=CARTESIAN_POINT ( 'NONE',  ( 106.8015515045248378, -6.936859964151250502, -18.39754474579286025 ) ) ;
#11696=CARTESIAN_POINT ( 'NONE',  ( 110.5266510812576826, -0.01829820670803256055, -12.14321520033831625 ) ) ;
#11697=CARTESIAN_POINT ( 'NONE',  ( 62.51159666141266058, -64.93666976841245742, -45.57438496592644128 ) ) ;
#11698=CARTESIAN_POINT ( 'NONE',  ( 109.9963952545248134, 0.8980012041604421569, -11.00651665394454071 ) ) ;
#11709=CARTESIAN_POINT ( 'NONE',  ( 116.9417077545247992, -2.791137627527939813, -18.39754474579286025 ) ) ;
#11710=CARTESIAN_POINT ( 'NONE',  ( 116.1082702545247827, -10.62599879583958717, -15.77991374673208469 ) ) ;
#11713=CIRCLE ( 'NONE', #26293, 4.500000000000003553 ) ;
#11716=CARTESIAN_POINT ( 'NONE',  ( 109.3713171295247832, -10.62599879583958540, -13.39321520033831447 ) ) ;
#11720=CARTESIAN_POINT ( 'NONE',  ( 116.6689336878302043, -11.83255234646479082, -6.347766163431310282 ) ) ;
#11721=CARTESIAN_POINT ( 'NONE',  ( 106.8015515045248378, -6.936859964151250502, -18.39754474579286025 ) ) ;
#11723=CARTESIAN_POINT ( 'NONE',  ( 116.1777233795247781, -8.938348069036489818, -17.46756447353520159 ) ) ;
#11724=CARTESIAN_POINT ( 'NONE',  ( 109.2294641300314595, -10.43693616051014139, -13.09401194842305038 ) ) ;
#11726=CARTESIAN_POINT ( 'NONE',  ( 111.3854577545248645, -2.791137627527939813, -18.39754474579286025 ) ) ;
#11727=CARTESIAN_POINT ( 'NONE',  ( 106.3153796295248412, -4.863998795839590272, -19.15521520033831493 ) ) ;
#11733=ORIENTED_EDGE ( 'NONE', *, *, #3745, .T. ) ;
#11734=EDGE_CURVE ( 'NONE', #22330, #24453, #30576, .T. ) ;
#11737=VECTOR ( 'NONE', #29599, 1000.000000000000000 ) ;
#11748=DIRECTION ( 'NONE',  ( -1.000000000000000000, 0.000000000000000000, 0.000000000000000000 ) ) ;
#11750=CARTESIAN_POINT ( 'NONE',  ( 114.0246765045248196, -2.791137627527939813, -8.388885654883777576 ) ) ;
#11751=CARTESIAN_POINT ( 'NONE',  ( 73.47343079648352671, -1.934511955536642791, -12.14321520033831625 ) ) ;
#11756=CARTESIAN_POINT ( 'NONE',  ( 109.1629577545248395, -2.791137627527939813, -18.39754474579286025 ) ) ;
#11766=B_SPLINE_CURVE_WITH_KNOTS ( 'NONE', 3,
 ( #4866, #40207, #36317, #26073, #32889, #1664, #1442, #5087, #15139, #8740, #36095, #11949, #32674, #15365, #29269, #12400, #29713, #43184, #5536, #26300, #2110, #25846, #16038, #39977, #33118, #15588, #11720, #1225, #19453, #29946, #19003, #29491, #22648, #12171, #39536 ),
 .UNSPECIFIED., .F., .F.,
 ( 4, 2, 2, 1, 1, 2, 2, 2, 2, 1, 1, 2, 2, 2, 2, 1, 1, 1, 2, 2, 4 ),
 ( 0.000000000000000000, 0.1249999999999536482, 0.1874999999999301670, 0.2187499999999181211, 0.2343749999999113487, 0.2421874999999079625, 0.2499999999999046041, 0.3749999999998828160, 0.4374999999998722688, 0.4687499999998676059, 0.4843749999998684386, 0.4921874999998683831, 0.4999999999998683275, 0.6249999999999567013, 0.6875000000000006661, 0.7187500000000220934, 0.7343750000000325295, 0.7421875000000374145, 0.7460937500000398570, 0.7500000000000422995, 1.000000000000000000 ),
 .UNSPECIFIED. ) ;
#11767=CARTESIAN_POINT ( 'NONE',  ( 110.8992858795247827, -8.402594152722688392, -9.854619843455216355 ) ) ;
#11773=CARTESIAN_POINT ( 'NONE',  ( 107.5655358795247736, -0.7896495226426338832, -17.46756447353520159 ) ) ;
#11777=CARTESIAN_POINT ( 'NONE',  ( 108.7294421295247844, -9.051693226400931991, -21.39321520033831447 ) ) ;
#11780=CARTESIAN_POINT ( 'NONE',  ( 113.7468640045248236, -10.62599879583958717, -11.00651665394454604 ) ) ;
#11782=CARTESIAN_POINT ( 'NONE',  ( 83.87387534288872359, -31.73118616881930620, -23.27653720400033066 ) ) ;
#11785=CARTESIAN_POINT ( 'NONE',  ( 106.6626452545248611, 0.8980012041604421569, -11.00651665394454071 ) ) ;
#11796=CARTESIAN_POINT ( 'NONE',  ( 112.4272546295247821, -4.863998795839590272, -7.631215200338315796 ) ) ;
#11797=VECTOR ( 'NONE', #37643, 1000.000000000000000 ) ;
#11799=DIRECTION ( 'NONE',  ( -1.000000000000000000, 0.000000000000000000, 0.000000000000000000 ) ) ;
#11806=AXIS2_PLACEMENT_3D ( 'NONE', #13691, #7497, #24614 ) ;
#11811=CARTESIAN_POINT ( 'NONE',  ( 64.21004395737219284, -35.06008033345069919, -5.893215200338315363 ) ) ;
#11824=AXIS2_PLACEMENT_3D ( 'NONE', #16268, #29712, #26299 ) ;
#11826=CARTESIAN_POINT ( 'NONE',  ( 115.7610046295247912, -4.863998795839590272, -7.631215200338315796 ) ) ;
#11827=CARTESIAN_POINT ( 'NONE',  ( 114.2330358795247776, -8.402594152722688392, -9.854619843455216355 ) ) ;
#11830=AXIS2_PLACEMENT_3D ( 'NONE', #30159, #1872, #27195 ) ;
#11838=CARTESIAN_POINT ( 'NONE',  ( 107.4960827545248350, -6.936859964151250502, -8.388885654883777576 ) ) ;
#11848=DIRECTION ( 'NONE',  ( 1.000000000000000000, 0.000000000000000000, 0.000000000000000000 ) ) ;
#11863=DIRECTION ( 'NONE',  ( 1.000000000000000000, 0.000000000000000000, 0.000000000000000000 ) ) ;
#11865=CARTESIAN_POINT ( 'NONE',  ( 115.2035566399283795, 0.4261359969231631739, -14.64321520033831447 ) ) ;
#11880=CARTESIAN_POINT ( 'NONE',  ( 115.8304577545247582, -7.250697342233347165, -7.631215200338321125 ) ) ;
#11881=CARTESIAN_POINT ( 'NONE',  ( 108.9545983795247821, -8.402594152722688392, -16.93181055722141792 ) ) ;
#11882=CARTESIAN_POINT ( 'NONE',  ( 109.7880358795247986, -8.402594152722688392, -9.854619843455216355 ) ) ;
#11887=CARTESIAN_POINT ( 'NONE',  ( 107.9822546295247889, -4.863998795839590272, -7.631215200338315796 ) ) ;
#11888=CYLINDRICAL_SURFACE ( 'NONE', #41643, 15.90000000000000036 ) ;
#11893=CARTESIAN_POINT ( 'NONE',  ( 112.2883483795247770, -0.7896495226426338832, -9.318865927141430916 ) ) ;
#11894=CARTESIAN_POINT ( 'NONE',  ( 111.9410827545248708, -6.936859964151250502, -8.388885654883777576 ) ) ;
#11898=VECTOR ( 'NONE', #41685, 1000.000000000000000 ) ;
#11904=VERTEX_POINT ( 'NONE', #19116 ) ;
#11910=ORIENTED_EDGE ( 'NONE', *, *, #15956, .T. ) ;
#11913=ADVANCED_FACE ( 'NONE', ( #16609 ), #13417, .T. ) ;
#11914=CARTESIAN_POINT ( 'NONE',  ( 108.1211608795247798, -1.325403438956436419, -16.93181055722141792 ) ) ;
#11923=CARTESIAN_POINT ( 'NONE',  ( 61.80744621386338622, -65.84115252037693722, -43.66573742411122083 ) ) ;
#11924=CARTESIAN_POINT ( 'NONE',  ( 110.5520202545248054, -10.62599879583958717, -15.77991374673208469 ) ) ;
#11934=VERTEX_POINT ( 'NONE', #6105 ) ;
#11937=CARTESIAN_POINT ( 'NONE',  ( 111.9410827545248708, -2.477300249445798297, -19.15521520033831138 ) ) ;
#11938=AXIS2_PLACEMENT_3D ( 'NONE', #11982, #32924, #1258 ) ;
#11939=CARTESIAN_POINT ( 'NONE',  ( 116.5249890045247980, -9.868328341294098749, -11.32035403202665869 ) ) ;
#11940=CARTESIAN_POINT ( 'NONE',  ( 111.2465515045248168, -2.477300249445798297, -7.631215200338321125 ) ) ;
#11942=VERTEX_POINT ( 'NONE', #43970 ) ;
#11944=CARTESIAN_POINT ( 'NONE',  ( 62.50008149197554275, -37.25231330516801620, -5.285959774307153580 ) ) ;
#11945=CARTESIAN_POINT ( 'NONE',  ( 108.1906140045248463, -10.62599879583958717, -11.00651665394454604 ) ) ;
#11949=CARTESIAN_POINT ( 'NONE',  ( 117.1139656878117563, -11.30305607403721879, -5.600395450087082949 ) ) ;
#11952=CARTESIAN_POINT ( 'NONE',  ( 109.2294401191927165, -10.32848583145956844, -14.25478553988458685 ) ) ;
#11954=CARTESIAN_POINT ( 'NONE',  ( 113.0523327545247838, -6.936859964151250502, -8.388885654883777576 ) ) ;
#11955=CARTESIAN_POINT ( 'NONE',  ( 115.8999108795247821, -1.325403438956436419, -16.93181055722141792 ) ) ;
#11958=CARTESIAN_POINT ( 'NONE',  ( 69.81869296892593013, -25.88089094749368613, -5.787280954910575481 ) ) ;
#11961=ORIENTED_EDGE ( 'NONE', *, *, #20393, .F. ) ;
#11967=VERTEX_POINT ( 'NONE', #40776 ) ;
#11969=EDGE_CURVE ( 'NONE', #19575, #12207, #9799, .T. ) ;
#11970=EDGE_CURVE ( 'NONE', #38354, #14378, #37334, .T. ) ;
#11977=CARTESIAN_POINT ( 'NONE',  ( 113.7468640045248236, 0.1403307496149616695, -15.46607636864997204 ) ) ;
#11982=CARTESIAN_POINT ( 'NONE',  ( 117.2294421295247844, -4.863998795839590272, -13.39321520033831447 ) ) ;
#11984=FACE_OUTER_BOUND ( 'NONE', #19609, .T. ) ;
#11985=CARTESIAN_POINT ( 'NONE',  ( 112.6356140045247827, 0.1403307496149616695, -15.46607636864997204 ) ) ;
#11992=EDGE_LOOP ( 'NONE', ( #2881, #1461, #20339, #34702, #31543, #7825, #40094, #12369, #37061, #19538, #15018, #25291, #39262, #8591, #14216, #17624, #13425, #8245, #34653, #16234, #32883, #12028, #23987 ) ) ;
#11995=CARTESIAN_POINT ( 'NONE',  ( 109.8574890045247940, -9.868328341294098749, -11.32035403202665869 ) ) ;
#12000=CARTESIAN_POINT ( 'NONE',  ( 109.9963952545248134, 0.8980012041604421569, -11.00651665394454071 ) ) ;
#12003=CARTESIAN_POINT ( 'NONE',  ( 61.76986277844709861, -39.32091226840162079, -4.893215200338314474 ) ) ;
#12006=CARTESIAN_POINT ( 'NONE',  ( 114.8581140045248361, -10.62599879583958717, -11.00651665394454604 ) ) ;
#12007=( BOUNDED_SURFACE ( )  B_SPLINE_SURFACE ( 1, 2, ( 
 ( #990, #28816, #18549, #11709, #15352, #25619, #22189, #1654, #18774, #11939, #32663, #29480, #25835, #1431, #29259, #43170, #39742, #36307, #5075, #18992, #43393, #12160, #5308, #13064, #2557, #20358, #23094, #27425, #9875, #2789, #10103, #23317, #5523, #19443, #9188, #33326, #30161, #2100, #34244, #6213, #37203, #16027, #29935, #27198, #3017, #16939, #2330, #23785, #16486, #9407, #30834, #44757, #26963, #36976, #43849, #16260, #16716, #41346, #9638, #44080, #12618, #5744, #13516, #37674, #36755, #40884, #20134, #30609, #6450, #26519, #44309, #40428, #13290, #30386, #19664, #34020, #33552, #23560, #12844, #26745, #37441, #41116, #40652, #5975, #44527, #19901, #33786, #18042, #43059, #7320, #21241, #17164, #24007, #38330, #10762, #13957, #44981, #703, #24886, #3464, #13739, #485, #35118, #20799, #28090, #14398, #6889, #7550, #38779, #27648, #7106, #34890, #3679, #31270, #31937, #15237, #29146, #17381, #17600, #38115, #35348, #3901, #31052, #31493, #37894, #17819, #264, #41562, #10322, #4123, #24225, #34679, #6673, #14173, #43, #21016, #24659, #41999, #38545, #21465, #27868, #20580, #42221, #31716, #34459, #10537, #3238, #41782, #24439, #28309, #10982, #22308, #9305, #26404, #1546, #26631, #1769, #23213, #36870, #5193, #40544 ),
 ( #22528, #43738, #18881, #8628, #22981, #39863, #2217, #5866, #30273, #40314, #9078, #4971, #11826, #26179, #12508, #15695, #32772, #33672, #12728, #36424, #15467, #33438, #5640, #19111, #15925, #16147, #32995, #37092, #19788, #29373, #40087, #22748, #36649, #29597, #2450, #16370, #25733, #43514, #5422, #25956, #39640, #19561, #43284, #19339, #8404, #30051, #33224, #12055, #12283, #36204, #8848, #1999, #29822, #43964, #44417, #16832, #6556, #27313, #30725, #6787, #2672, #31168, #41452, #3134, #13845, #20248, #12960, #26856, #33902, #40769, #41007, #9527, #20696, #20473, #6099, #38012, #37562, #34574, #17057, #9760, #3358, #13410, #23443, #44873, #6331, #37328, #20019, #44198, #37783, #13183, #27086, #45089, #16604, #30497, #34354, #23672, #17276, #10210, #34134, #2903, #44648, #30949, #13629, #24118, #41231, #9991, #23900, #27540, #5112, #26096, #37242, #26783, #30424, #43885, #9226, #33591, #40691, #19937, #2134, #16525, #16297, #19481, #8766, #23135, #15610, #33362, #19261, #9444, #5561, #30197, #29517, #9000, #29738, #6013, #22897, #37013, #22672, #23357, #5783, #44116, #16064, #12656, #29970, #44343, #13102, #36568, #1913, #1691, #26552, #40465, #19703, #43649, #40233, #12883, #36340, #26326, #19028, #36792, #12425, #39777, #32914 ) ),
 .UNSPECIFIED., .F., .F., .T. ) 
 B_SPLINE_SURFACE_WITH_KNOTS ( ( 2, 2 ),
 ( 3, 2, 2, 2, 2, 2, 2, 2, 2, 2, 2, 2, 2, 2, 2, 2, 2, 2, 2, 2, 2, 2, 2, 2, 2, 2, 2, 2, 2, 2, 2, 2, 2, 2, 2, 2, 2, 2, 2, 2, 2, 2, 2, 2, 2, 2, 2, 2, 2, 2, 2, 2, 2, 2, 2, 2, 2, 2, 2, 2, 2, 2, 2, 2, 2, 2, 2, 2, 2, 2, 2, 2, 2, 2, 2, 2, 2, 2, 2, 2, 3 ),
 ( 0.000000000000000000, 1.000000000000000000 ),
 ( 0.000000000000000000, 0.01250000000000000069, 0.02500000000000000139, 0.03749999999999999861, 0.05000000000000000278, 0.06250000000000000000, 0.07499999999999999722, 0.08749999999999999445, 0.1000000000000000056, 0.1125000000000000028, 0.1250000000000000000, 0.1375000000000000111, 0.1499999999999999944, 0.1625000000000000056, 0.1749999999999999889, 0.1875000000000000000, 0.2000000000000000111, 0.2124999999999999944, 0.2250000000000000056, 0.2374999999999999889, 0.2500000000000000000, 0.2625000000000000111, 0.2750000000000000222, 0.2874999999999999778, 0.2999999999999999889, 0.3125000000000000000, 0.3250000000000000111, 0.3375000000000000222, 0.3499999999999999778, 0.3624999999999999889, 0.3750000000000000000, 0.3875000000000000111, 0.4000000000000000222, 0.4124999999999999778, 0.4249999999999999889, 0.4375000000000000000, 0.4500000000000000111, 0.4625000000000000222, 0.4749999999999999778, 0.4874999999999999889, 0.5000000000000000000, 0.5124999999999999556, 0.5250000000000000222, 0.5374999999999999778, 0.5500000000000000444, 0.5625000000000000000, 0.5749999999999999556, 0.5875000000000000222, 0.5999999999999999778, 0.6125000000000000444, 0.6250000000000000000, 0.6374999999999999556, 0.6500000000000000222, 0.6624999999999999778, 0.6750000000000000444, 0.6875000000000000000, 0.6999999999999999556, 0.7125000000000000222, 0.7249999999999999778, 0.7375000000000000444, 0.7500000000000000000, 0.7624999999999999556, 0.7750000000000000222, 0.7874999999999999778, 0.8000000000000000444, 0.8125000000000000000, 0.8249999999999999556, 0.8375000000000000222, 0.8499999999999999778, 0.8625000000000000444, 0.8750000000000000000, 0.8874999999999999556, 0.9000000000000000222, 0.9124999999999999778, 0.9250000000000000444, 0.9375000000000000000, 0.9499999999999999556, 0.9625000000000000222, 0.9749999999999999778, 0.9875000000000000444, 1.000000000000000000 ),
 .UNSPECIFIED. ) 
 GEOMETRIC_REPRESENTATION_ITEM ( )  RATIONAL_B_SPLINE_SURFACE ( (
 ( 1.000000000000000000, 0.9238795325112869605, 1.000000000000000000, 0.9238795325112869605, 1.000000000000000000, 0.9238795325112869605, 1.000000000000000000, 0.9238795325112869605, 1.000000000000000000, 0.9238795325112869605, 1.000000000000000000, 0.9238795325112869605, 1.000000000000000000, 0.9238795325112869605, 1.000000000000000000, 0.9238795325112869605, 1.000000000000000000, 0.9238795325112869605, 1.000000000000000000, 0.9238795325112869605, 1.000000000000000000, 0.9238795325112869605, 1.000000000000000000, 0.9238795325112869605, 1.000000000000000000, 0.9238795325112869605, 1.000000000000000000, 0.9238795325112869605, 1.000000000000000000, 0.9238795325112869605, 1.000000000000000000, 0.9238795325112869605, 1.000000000000000000, 0.9238795325112869605, 1.000000000000000000, 0.9238795325112869605, 1.000000000000000000, 0.9238795325112869605, 1.000000000000000000, 0.9238795325112869605, 1.000000000000000000, 0.9238795325112869605, 1.000000000000000000, 0.9238795325112869605, 1.000000000000000000, 0.9238795325112869605, 1.000000000000000000, 0.9238795325112869605, 1.000000000000000000, 0.9238795325112869605, 1.000000000000000000, 0.9238795325112869605, 1.000000000000000000, 0.9238795325112869605, 1.000000000000000000, 0.9238795325112869605, 1.000000000000000000, 0.9238795325112869605, 1.000000000000000000, 0.9238795325112869605, 1.000000000000000000, 0.9238795325112869605, 1.000000000000000000, 0.9238795325112869605, 1.000000000000000000, 0.9238795325112869605, 1.000000000000000000, 0.9238795325112869605, 1.000000000000000000, 0.9238795325112869605, 1.000000000000000000, 0.9238795325112869605, 1.000000000000000000, 0.9238795325112869605, 1.000000000000000000, 0.9238795325112869605, 1.000000000000000000, 0.9238795325112869605, 1.000000000000000000, 0.9238795325112869605, 1.000000000000000000, 0.9238795325112869605, 1.000000000000000000, 0.9238795325112869605, 1.000000000000000000, 0.9238795325112869605, 1.000000000000000000, 0.9238795325112869605, 1.000000000000000000, 0.9238795325112869605, 1.000000000000000000, 0.9238795325112869605, 1.000000000000000000, 0.9238795325112869605, 1.000000000000000000, 0.9238795325112869605, 1.000000000000000000, 0.9238795325112869605, 1.000000000000000000, 0.9238795325112869605, 1.000000000000000000, 0.9238795325112869605, 1.000000000000000000, 0.9238795325112869605, 1.000000000000000000, 0.9238795325112869605, 1.000000000000000000, 0.9238795325112869605, 1.000000000000000000, 0.9238795325112869605, 1.000000000000000000, 0.9238795325112869605, 1.000000000000000000, 0.9238795325112869605, 1.000000000000000000, 0.9238795325112869605, 1.000000000000000000, 0.9238795325112869605, 1.000000000000000000, 0.9238795325112869605, 1.000000000000000000, 0.9238795325112869605, 1.000000000000000000, 0.9238795325112869605, 1.000000000000000000, 0.9238795325112869605, 1.000000000000000000, 0.9238795325112869605, 1.000000000000000000, 0.9238795325112869605, 1.000000000000000000, 0.9238795325112869605, 1.000000000000000000, 0.9238795325112869605, 1.000000000000000000, 0.9238795325112869605, 1.000000000000000000, 0.9238795325112869605, 1.000000000000000000, 0.9238795325112869605, 1.000000000000000000, 0.9238795325112869605, 1.000000000000000000, 0.9238795325112869605, 1.000000000000000000, 0.9238795325112869605, 1.000000000000000000, 0.9238795325112869605, 1.000000000000000000, 0.9238795325112869605, 1.000000000000000000, 0.9238795325112869605, 1.000000000000000000, 0.9238795325112869605, 1.000000000000000000, 0.9238795325112869605, 1.000000000000000000, 0.9238795325112869605, 1.000000000000000000, 0.9238795325112869605, 1.000000000000000000),
 ( 1.000000000000000000, 0.9238795325112869605, 1.000000000000000000, 0.9238795325112869605, 1.000000000000000000, 0.9238795325112869605, 1.000000000000000000, 0.9238795325112869605, 1.000000000000000000, 0.9238795325112869605, 1.000000000000000000, 0.9238795325112869605, 1.000000000000000000, 0.9238795325112869605, 1.000000000000000000, 0.9238795325112869605, 1.000000000000000000, 0.9238795325112869605, 1.000000000000000000, 0.9238795325112869605, 1.000000000000000000, 0.9238795325112869605, 1.000000000000000000, 0.9238795325112869605, 1.000000000000000000, 0.9238795325112869605, 1.000000000000000000, 0.9238795325112869605, 1.000000000000000000, 0.9238795325112869605, 1.000000000000000000, 0.9238795325112869605, 1.000000000000000000, 0.9238795325112869605, 1.000000000000000000, 0.9238795325112869605, 1.000000000000000000, 0.9238795325112869605, 1.000000000000000000, 0.9238795325112869605, 1.000000000000000000, 0.9238795325112869605, 1.000000000000000000, 0.9238795325112869605, 1.000000000000000000, 0.9238795325112869605, 1.000000000000000000, 0.9238795325112869605, 1.000000000000000000, 0.9238795325112869605, 1.000000000000000000, 0.9238795325112869605, 1.000000000000000000, 0.9238795325112869605, 1.000000000000000000, 0.9238795325112869605, 1.000000000000000000, 0.9238795325112869605, 1.000000000000000000, 0.9238795325112869605, 1.000000000000000000, 0.9238795325112869605, 1.000000000000000000, 0.9238795325112869605, 1.000000000000000000, 0.9238795325112869605, 1.000000000000000000, 0.9238795325112869605, 1.000000000000000000, 0.9238795325112869605, 1.000000000000000000, 0.9238795325112869605, 1.000000000000000000, 0.9238795325112869605, 1.000000000000000000, 0.9238795325112869605, 1.000000000000000000, 0.9238795325112869605, 1.000000000000000000, 0.9238795325112869605, 1.000000000000000000, 0.9238795325112869605, 1.000000000000000000, 0.9238795325112869605, 1.000000000000000000, 0.9238795325112869605, 1.000000000000000000, 0.9238795325112869605, 1.000000000000000000, 0.9238795325112869605, 1.000000000000000000, 0.9238795325112869605, 1.000000000000000000, 0.9238795325112869605, 1.000000000000000000, 0.9238795325112869605, 1.000000000000000000, 0.9238795325112869605, 1.000000000000000000, 0.9238795325112869605, 1.000000000000000000, 0.9238795325112869605, 1.000000000000000000, 0.9238795325112869605, 1.000000000000000000, 0.9238795325112869605, 1.000000000000000000, 0.9238795325112869605, 1.000000000000000000, 0.9238795325112869605, 1.000000000000000000, 0.9238795325112869605, 1.000000000000000000, 0.9238795325112869605, 1.000000000000000000, 0.9238795325112869605, 1.000000000000000000, 0.9238795325112869605, 1.000000000000000000, 0.9238795325112869605, 1.000000000000000000, 0.9238795325112869605, 1.000000000000000000, 0.9238795325112869605, 1.000000000000000000, 0.9238795325112869605, 1.000000000000000000, 0.9238795325112869605, 1.000000000000000000, 0.9238795325112869605, 1.000000000000000000, 0.9238795325112869605, 1.000000000000000000, 0.9238795325112869605, 1.000000000000000000, 0.9238795325112869605, 1.000000000000000000, 0.9238795325112869605, 1.000000000000000000, 0.9238795325112869605, 1.000000000000000000, 0.9238795325112869605, 1.000000000000000000, 0.9238795325112869605, 1.000000000000000000, 0.9238795325112869605, 1.000000000000000000, 0.9238795325112869605, 1.000000000000000000, 0.9238795325112869605, 1.000000000000000000, 0.9238795325112869605, 1.000000000000000000, 0.9238795325112869605, 1.000000000000000000, 0.9238795325112869605, 1.000000000000000000, 0.9238795325112869605, 1.000000000000000000, 0.9238795325112869605, 1.000000000000000000) ) ) 
 REPRESENTATION_ITEM ( '' )  SURFACE ( )  );
#12009=CARTESIAN_POINT ( 'NONE',  ( 83.51226282631382958, -32.71650970335249298, -21.69069357203322213 ) ) ;
#12012=CARTESIAN_POINT ( 'NONE',  ( 107.9128015045248219, -2.477300249445798297, -7.631215200338321125 ) ) ;
#12014=DIRECTION ( 'NONE',  ( -1.000000000000000000, 1.091021054073464066E-15, 0.000000000000000000 ) ) ;
#12016=CARTESIAN_POINT ( 'NONE',  ( 112.4235952706805790, 0.3193521225029610777, -14.64321520033830026 ) ) ;
#12024=CARTESIAN_POINT ( 'NONE',  ( 109.4407702545248355, -10.62599879583958717, -15.77991374673208469 ) ) ;
#12026=CARTESIAN_POINT ( 'NONE',  ( 110.7603796295247918, -4.863998795839590272, -19.15521520033831493 ) ) ;
#12027=FACE_OUTER_BOUND ( 'NONE', #4193, .T. ) ;
#12028=ORIENTED_EDGE ( 'NONE', *, *, #38977, .F. ) ;
#12032=ORIENTED_EDGE ( 'NONE', *, *, #24000, .F. ) ;
#12035=CARTESIAN_POINT ( 'NONE',  ( 77.77634386988368931, 3.254514819260763581, -14.64321520033831447 ) ) ;
#12038=CARTESIAN_POINT ( 'NONE',  ( 64.18133890301322708, -35.39523410098156120, -5.871648730333205890 ) ) ;
#12050=CARTESIAN_POINT ( 'NONE',  ( 113.1217858795247935, -8.402594152722688392, -9.854619843455216355 ) ) ;
#12055=CARTESIAN_POINT ( 'NONE',  ( 113.3301452545248083, 0.8980012041604421569, -11.00651665394454071 ) ) ;
#12056=CARTESIAN_POINT ( 'NONE',  ( 110.6214733795247867, -1.325403438956436419, -9.854619843455211026 ) ) ;
#12061=CARTESIAN_POINT ( 'NONE',  ( 116.8028015045247940, -6.936859964151250502, -18.39754474579286025 ) ) ;
#12062=ORIENTED_EDGE ( 'NONE', *, *, #41297, .F. ) ;
#12067=CARTESIAN_POINT ( 'NONE',  ( 106.1764733795248219, -1.325403438956436419, -9.854619843455211026 ) ) ;
#12070=DIRECTION ( 'NONE',  ( 0.9387755102040816757, -0.3445294493088600918, 0.000000000000000000 ) ) ;
#12074=CARTESIAN_POINT ( 'NONE',  ( 71.77086717554882966, -26.54201219542348511, -4.893215200338314474 ) ) ;
#12077=CARTESIAN_POINT ( 'NONE',  ( 71.37572422742091760, -11.86958442233774313, -21.89321520033831447 ) ) ;
#12080=ORIENTED_EDGE ( 'NONE', *, *, #7456, .T. ) ;
#12086=ORIENTED_EDGE ( 'NONE', *, *, #33114, .F. ) ;
#12091=CARTESIAN_POINT ( 'NONE',  ( 109.9649712410415816, 0.7607806665038616689, -12.14321520033831625 ) ) ;
#12095=EDGE_CURVE ( 'NONE', #22775, #5648, #16152, .T. ) ;
#12100=CARTESIAN_POINT ( 'NONE',  ( 116.6348121297881733, -9.548805560831048922, -15.25421616637334488 ) ) ;
#12106=CARTESIAN_POINT ( 'NONE',  ( 114.9716510812576757, -0.01829820670803256055, -12.14321520033831625 ) ) ;
#12107=CARTESIAN_POINT ( 'NONE',  ( 110.8992858795247827, -0.7896495226426338832, -17.46756447353520159 ) ) ;
#12109=CARTESIAN_POINT ( 'NONE',  ( 109.5796765045248122, -2.791137627527939813, -8.388885654883777576 ) ) ;
#12110=CARTESIAN_POINT ( 'NONE',  ( 108.5378796295247810, -4.863998795839590272, -8.388885654883775800 ) ) ;
#12113=VERTEX_POINT ( 'NONE', #2223 ) ;
#12114=CARTESIAN_POINT ( 'NONE',  ( 105.9681140045248355, -10.62599879583958717, -11.00651665394454604 ) ) ;
#12118=CIRCLE ( 'NONE', #12839, 5.132259260909266985 ) ;
#12120=CARTESIAN_POINT ( 'NONE',  ( 111.6632702545248605, -10.62599879583958717, -15.77991374673208469 ) ) ;
#12121=CARTESIAN_POINT ( 'NONE',  ( 117.2294421295247844, 1.035107641088057973, -21.72657133228191739 ) ) ;
#12127=CARTESIAN_POINT ( 'NONE',  ( 61.27778620743471549, -25.99489077589588604, -13.39321520033831447 ) ) ;
#12138=CARTESIAN_POINT ( 'NONE',  ( 107.3571765045248299, -2.791137627527939813, -8.388885654883777576 ) ) ;
#12141=ORIENTED_EDGE ( 'NONE', *, *, #15267, .T. ) ;
#12142=EDGE_LOOP ( 'NONE', ( #3094, #5776, #699, #18358 ) ) ;
#12145=DIRECTION ( 'NONE',  ( 0.000000000000000000, 0.000000000000000000, 1.000000000000000000 ) ) ;
#12150=CARTESIAN_POINT ( 'NONE',  ( 107.4266296295248821, -4.863998795839590272, -19.15521520033831493 ) ) ;
#12156=ORIENTED_EDGE ( 'NONE', *, *, #36779, .F. ) ;
#12159=CARTESIAN_POINT ( 'NONE',  ( 113.1912390045248031, 0.8980012041604421569, -15.77991374673208469 ) ) ;
#12160=CARTESIAN_POINT ( 'NONE',  ( 115.6915515045247531, -6.936859964151250502, -18.39754474579286025 ) ) ;
#12161=CARTESIAN_POINT ( 'NONE',  ( 111.6632702545248605, -10.62599879583958717, -15.77991374673208469 ) ) ;
#12171=CARTESIAN_POINT ( 'NONE',  ( 116.4298796982476318, -11.97487242489886761, -6.682657204922437089 ) ) ;
#12175=CARTESIAN_POINT ( 'NONE',  ( 109.2294431053738464, -10.03736769325571032, -11.07138121511321316 ) ) ;
#12177=CARTESIAN_POINT ( 'NONE',  ( 110.2047546295247855, -4.863998795839590272, -18.39754474579285315 ) ) ;
#12178=CARTESIAN_POINT ( 'NONE',  ( 105.4819421295248247, 0.8980012041604618078, -13.39321520033831447 ) ) ;
#12181=CARTESIAN_POINT ( 'NONE',  ( 70.09935913692072518, -25.95240877518153511, -5.724109476187205559 ) ) ;
#12195=CARTESIAN_POINT ( 'NONE',  ( 70.19189222814998175, -63.93370346063255738, -42.00736267657491396 ) ) ;
#12196=EDGE_CURVE ( 'NONE', #22388, #25605, #26636, .T. ) ;
#12201=CARTESIAN_POINT ( 'NONE',  ( 111.0381921295247878, -9.868328341294093420, -13.39321520033831447 ) ) ;
#12202=DIRECTION ( 'NONE',  ( 3.183628217498455203E-14, 1.000000000000000000, 0.000000000000000000 ) ) ;
#12206=FACE_OUTER_BOUND ( 'NONE', #2551, .T. ) ;
#12207=VERTEX_POINT ( 'NONE', #5872 ) ;
#12209=CARTESIAN_POINT ( 'NONE',  ( 110.3436608795247764, -1.325403438956436419, -16.93181055722141792 ) ) ;
#12210=VECTOR ( 'NONE', #32488, 999.9999999999998863 ) ;
#12215=DIRECTION ( 'NONE',  ( 1.000000000000000000, 0.000000000000000000, 0.000000000000000000 ) ) ;
#12220=DIRECTION ( 'NONE',  ( 0.000000000000000000, 0.000000000000000000, 1.000000000000000000 ) ) ;
#12221=CARTESIAN_POINT ( 'NONE',  ( 111.0381921295247878, -9.868328341294093420, -13.39321520033831447 ) ) ;
#12228=CARTESIAN_POINT ( 'NONE',  ( 107.0793640045248196, -10.62599879583958717, -11.00651665394454604 ) ) ;
#12229=DIRECTION ( 'NONE',  ( 1.000000000000000000, 0.000000000000000000, 0.000000000000000000 ) ) ;
#12231=LINE ( 'NONE', #5145, #6644 ) ;
#12233=CARTESIAN_POINT ( 'NONE',  ( 110.8298327545248299, -2.477300249445798297, -19.15521520033831138 ) ) ;
#12235=CARTESIAN_POINT ( 'NONE',  ( 117.2294421295247844, 1.035107641088057973, -21.72657133228191739 ) ) ;
#12238=CARTESIAN_POINT ( 'NONE',  ( 107.0099108795247815, -8.938348069036489818, -9.318865927141430916 ) ) ;
#12240=CARTESIAN_POINT ( 'NONE',  ( 78.69189222814998175, -69.76310523276724496, -16.89321520033831447 ) ) ;
#12254=CARTESIAN_POINT ( 'NONE',  ( 110.4825671295247815, -10.62599879583958540, -13.39321520033831447 ) ) ;
#12256=CARTESIAN_POINT ( 'NONE',  ( 110.6214733795247867, -8.938348069036441856, -17.46756447353520869 ) ) ;
#12267=CARTESIAN_POINT ( 'NONE',  ( 79.79010115959992788, 5.106172230548759572, -4.893215200338314474 ) ) ;
#12279=CARTESIAN_POINT ( 'NONE',  ( 113.6774108795247997, -1.325403438956436419, -16.93181055722141792 ) ) ;
#12283=CARTESIAN_POINT ( 'NONE',  ( 113.2606921295247702, 0.8980012041604618078, -13.39321520033831447 ) ) ;
#12284=CARTESIAN_POINT ( 'NONE',  ( 107.9128015045248219, -6.936859964151250502, -18.39754474579286025 ) ) ;
#12287=CARTESIAN_POINT ( 'NONE',  ( 115.4137390045248566, -9.868328341294098749, -11.32035403202665869 ) ) ;
#12293=CARTESIAN_POINT ( 'NONE',  ( 108.0517077545248696, -2.791137627527939813, -18.39754474579286025 ) ) ;
#12304=CARTESIAN_POINT ( 'NONE',  ( 112.7050671295247923, 0.1403307496149613920, -13.39321520033831447 ) ) ;
#12325=AXIS2_PLACEMENT_3D ( 'NONE', #13573, #24066, #21071 ) ;
#12330=ORIENTED_EDGE ( 'NONE', *, *, #2358, .T. ) ;
#12332=CARTESIAN_POINT ( 'NONE',  ( 110.1353015045248469, -2.477300249445798297, -7.631215200338321125 ) ) ;
#12333=CARTESIAN_POINT ( 'NONE',  ( 111.4549108795247747, -1.325403438956436419, -16.93181055722141792 ) ) ;
#12334=CARTESIAN_POINT ( 'NONE',  ( 107.3571765045248299, -2.791137627527939813, -8.388885654883777576 ) ) ;
#12337=EDGE_LOOP ( 'NONE', ( #27396, #29829, #4098, #38717, #35825, #35250, #41670, #27463, #17682, #9145, #16580 ) ) ;
#12340=DIRECTION ( 'NONE',  ( 0.000000000000000000, 0.000000000000000000, 1.000000000000000000 ) ) ;
#12343=EDGE_CURVE ( 'NONE', #21853, #40407, #15340, .T. ) ;
#12345=CARTESIAN_POINT ( 'NONE',  ( 110.8298327545248299, -2.477300249445798297, -19.15521520033831138 ) ) ;
#12348=CARTESIAN_POINT ( 'NONE',  ( 110.8068531537514758, 0.4930828106259610433, -14.64321520033834645 ) ) ;
#12366=CARTESIAN_POINT ( 'NONE',  ( 110.2047546295247855, -4.863998795839590272, -7.631215200338315796 ) ) ;
#12368=ORIENTED_EDGE ( 'NONE', *, *, #15250, .T. ) ;
#12369=ORIENTED_EDGE ( 'NONE', *, *, #1596, .F. ) ;
#12372=VECTOR ( 'NONE', #25165, 1000.000000000000000 ) ;
#12374=CARTESIAN_POINT ( 'NONE',  ( 62.33173950417162246, -36.13435100893377694, -5.771259754798731656 ) ) ;
#12375=AXIS2_PLACEMENT_3D ( 'NONE', #42185, #21649, #10727 ) ;
#12379=CARTESIAN_POINT ( 'NONE',  ( 107.2182702545248105, -10.62599879583958717, -15.77991374673208469 ) ) ;
#12389=CARTESIAN_POINT ( 'NONE',  ( 113.7468640045248236, -10.62599879583958717, -11.00651665394454604 ) ) ;
#12391=CARTESIAN_POINT ( 'NONE',  ( 113.3995983795247895, -0.7896495226426338832, -9.318865927141430916 ) ) ;
#12395=CARTESIAN_POINT ( 'NONE',  ( 62.81996251504057227, -37.57851814417504954, -5.091777875131382913 ) ) ;
#12396=CARTESIAN_POINT ( 'NONE',  ( 108.7462390045248242, 0.8980012041604421569, -15.77991374673208469 ) ) ;
#12400=CARTESIAN_POINT ( 'NONE',  ( 116.9757267558744047, -11.53487629098437317, -5.866158325263667095 ) ) ;
#12401=ORIENTED_EDGE ( 'NONE', *, *, #527, .T. ) ;
#12403=CARTESIAN_POINT ( 'NONE',  ( 109.2294499582155396, -8.941328865127285752, -16.92711395088718263 ) ) ;
#12405=CARTESIAN_POINT ( 'NONE',  ( 110.5520202545248054, 0.1403307496149616695, -11.32035403202665336 ) ) ;
#12406=CARTESIAN_POINT ( 'NONE',  ( 110.2742077545248094, -2.791137627527939813, -18.39754474579286025 ) ) ;
#12409=FACE_OUTER_BOUND ( 'NONE', #24854, .T. ) ;
#12410=CARTESIAN_POINT ( 'NONE',  ( 68.94757123365556595, -25.85038639872388799, -5.893215200338315363 ) ) ;
#12425=CARTESIAN_POINT ( 'NONE',  ( 105.6208483795248299, -0.7896495226426338832, -9.318865927141430916 ) ) ;
#12428=CARTESIAN_POINT ( 'NONE',  ( 110.8298327545248299, -6.936859964151250502, -8.388885654883777576 ) ) ;
#12431=AXIS2_PLACEMENT_3D ( 'NONE', #1723, #8579, #39367 ) ;
#12435=CARTESIAN_POINT ( 'NONE',  ( 61.69189222814998175, -49.76310523276723785, -4.893215200338314474 ) ) ;
#12436=ORIENTED_EDGE ( 'NONE', *, *, #24741, .T. ) ;
#12438=CARTESIAN_POINT ( 'NONE',  ( 107.8433483795247838, -8.402594152722688392, -16.93181055722141792 ) ) ;
#12443=CARTESIAN_POINT ( 'NONE',  ( 113.9552388068194801, 0.1168444861213632779, -12.14321520033831625 ) ) ;
#12446=ORIENTED_EDGE ( 'NONE', *, *, #1366, .F. ) ;
#12447=CARTESIAN_POINT ( 'NONE',  ( 110.2961459279789835, 0.1843591316377651834, -14.64321520033833934 ) ) ;
#12449=CARTESIAN_POINT ( 'NONE',  ( 109.0240515045248202, -6.936859964151250502, -18.39754474579286025 ) ) ;
#12453=CARTESIAN_POINT ( 'NONE',  ( 110.4131140045248287, -10.62599879583958717, -11.00651665394454604 ) ) ;
#12458=CARTESIAN_POINT ( 'NONE',  ( 112.7745202545247878, -10.62599879583958717, -15.77991374673208469 ) ) ;
#12460=CARTESIAN_POINT ( 'NONE',  ( 115.8999108795247821, -8.938348069036489818, -9.318865927141430916 ) ) ;
#12477=CARTESIAN_POINT ( 'NONE',  ( 108.6767858795247861, -0.7896495226426338832, -17.46756447353520159 ) ) ;
#12479=FACE_BOUND ( 'NONE', #901, .T. ) ;
#12481=ORIENTED_EDGE ( 'NONE', *, *, #6978, .F. ) ;
#12483=ADVANCED_FACE ( 'NONE', ( #28321 ), #3131, .T. ) ;
#12486=CIRCLE ( 'NONE', #37231, 0.8718221387495408425 ) ;
#12490=CARTESIAN_POINT ( 'NONE',  ( 114.2855644685027698, 0.6938714319018670640, -14.64321520033829493 ) ) ;
#12500=VERTEX_POINT ( 'NONE', #40559 ) ;
#12503=CARTESIAN_POINT ( 'NONE',  ( 117.0111608795247946, -1.325403438956436419, -16.93181055722141792 ) ) ;
#12508=CARTESIAN_POINT ( 'NONE',  ( 115.6220983795247861, -0.7896495226426338832, -9.318865927141430916 ) ) ;
#12509=CARTESIAN_POINT ( 'NONE',  ( 111.2465515045248168, -6.936859964151250502, -18.39754474579286025 ) ) ;
#12513=CARTESIAN_POINT ( 'NONE',  ( 111.7327233795247849, -1.325403438956436419, -9.854619843455211026 ) ) ;
#12520=CARTESIAN_POINT ( 'NONE',  ( 116.5028905619397079, -11.93022180958501544, -21.11349849701261050 ) ) ;
#12521=ORIENTED_EDGE ( 'NONE', *, *, #30606, .F. ) ;
#12523=AXIS2_PLACEMENT_3D ( 'NONE', #12077, #7518, #35547 ) ;
#12529=CARTESIAN_POINT ( 'NONE',  ( 114.0941296295247867, -4.863998795839590272, -8.388885654883775800 ) ) ;
#12538=ORIENTED_EDGE ( 'NONE', *, *, #295, .F. ) ;
#12556=ORIENTED_EDGE ( 'NONE', *, *, #39550, .F. ) ;
#12558=CARTESIAN_POINT ( 'NONE',  ( 111.8021765045248372, -7.250697342233347165, -19.15521520033831138 ) ) ;
#12559=CARTESIAN_POINT ( 'NONE',  ( 108.7462390045248242, -9.868328341294098749, -11.32035403202665869 ) ) ;
#12561=CARTESIAN_POINT ( 'NONE',  ( 109.2324108795247923, -1.325403438956436419, -16.93181055722141792 ) ) ;
#12565=CARTESIAN_POINT ( 'NONE',  ( 117.2294421295247844, -10.76310523276723785, -4.893215200338314474 ) ) ;
#12568=EDGE_CURVE ( 'NONE', #42269, #20890, #1615, .T. ) ;
#12570=CARTESIAN_POINT ( 'NONE',  ( 107.4266296295248821, -4.863998795839590272, -8.388885654883775800 ) ) ;
#12573=CARTESIAN_POINT ( 'NONE',  ( 109.3018640045248304, -10.62599879583958717, -11.00651665394454604 ) ) ;
#12574=CARTESIAN_POINT ( 'NONE',  ( 63.69189222814998175, -64.02637234200076932, -46.77412892735921446 ) ) ;
#12581=CARTESIAN_POINT ( 'NONE',  ( 143.3676850761856940, -50.16718729050181480, -4.893215200338314474 ) ) ;
#12594=CARTESIAN_POINT ( 'NONE',  ( 111.5243640045248412, -10.62599879583958717, -11.00651665394454604 ) ) ;
#12596=EDGE_LOOP ( 'NONE', ( #44834, #5726 ) ) ;
#12602=EDGE_CURVE ( 'NONE', #20584, #26785, #8051, .T. ) ;
#12603=CARTESIAN_POINT ( 'NONE',  ( 62.55594166779781773, -34.86283735444163767, -5.893215200338315363 ) ) ;
#12605=CARTESIAN_POINT ( 'NONE',  ( 106.4542858795248179, -0.7896495226426338832, -17.46756447353520159 ) ) ;
#12616=CARTESIAN_POINT ( 'NONE',  ( 112.3578015045248861, -2.477300249445798297, -7.631215200338321125 ) ) ;
#12618=CARTESIAN_POINT ( 'NONE',  ( 112.9828796295247884, -4.863998795839590272, -8.388885654883775800 ) ) ;
#12619=CARTESIAN_POINT ( 'NONE',  ( 110.8992858795247827, -0.7896495226426338832, -17.46756447353520159 ) ) ;
#12627=CARTESIAN_POINT ( 'NONE',  ( 106.7320983795247855, -0.7896495226426338832, -9.318865927141430916 ) ) ;
#12632=ORIENTED_EDGE ( 'NONE', *, *, #5077, .F. ) ;
#12638=CARTESIAN_POINT ( 'NONE',  ( 114.1635827545248389, -6.936859964151250502, -8.388885654883777576 ) ) ;
#12639=CARTESIAN_POINT ( 'NONE',  ( 109.3018640045248304, 0.1403307496149616695, -15.46607636864997204 ) ) ;
#12642=CARTESIAN_POINT ( 'NONE',  ( 69.25460375973102600, -25.92061903028353953, -5.871778085103695588 ) ) ;
#12656=CARTESIAN_POINT ( 'NONE',  ( 106.8015515045248378, -2.477300249445798297, -7.631215200338321125 ) ) ;
#12657=DIRECTION ( 'NONE',  ( 0.000000000000000000, -1.000000000000000000, 0.000000000000000000 ) ) ;
#12659=CARTESIAN_POINT ( 'NONE',  ( 110.6909265045248247, -2.791137627527939813, -8.388885654883777576 ) ) ;
#12660=DIRECTION ( 'NONE',  ( 3.332709719099110404E-30, -9.283845114648369353E-44, 1.000000000000000000 ) ) ;
#12665=CARTESIAN_POINT ( 'NONE',  ( 116.3892577545247349, -6.935066607705044461, -8.393215200338321580 ) ) ;
#12667=CARTESIAN_POINT ( 'NONE',  ( 117.2294421295247844, -9.690077956319688823, -4.893215200338314474 ) ) ;
#12670=CARTESIAN_POINT ( 'NONE',  ( 70.27992438911469719, -26.36696139213632506, -5.630764001613508540 ) ) ;
#12675=CARTESIAN_POINT ( 'NONE',  ( 110.3910934012278773, 0.04929351793716424401, -14.64321520033829493 ) ) ;
#12677=CARTESIAN_POINT ( 'NONE',  ( 111.3854577545248645, -2.791137627527939813, -18.39754474579286025 ) ) ;
#12681=CARTESIAN_POINT ( 'NONE',  ( 105.8986608795248401, -8.938348069036489818, -9.318865927141430916 ) ) ;
#12685=CARTESIAN_POINT ( 'NONE',  ( 112.0799890045248475, 0.8980012041604421569, -15.77991374673208469 ) ) ;
#12687=CARTESIAN_POINT ( 'NONE',  ( 115.2053796295247849, -4.863998795839590272, -19.15521520033831493 ) ) ;
#12702=CARTESIAN_POINT ( 'NONE',  ( 111.0381921295247878, 0.8980012041604618078, -13.39321520033831447 ) ) ;
#12704=CARTESIAN_POINT ( 'NONE',  ( 116.7875679639338244, -3.298653660685034961, -18.34516049763993450 ) ) ;
#12705=CARTESIAN_POINT ( 'NONE',  ( 116.5249890045247980, 0.8980012041604421569, -15.77991374673208469 ) ) ;
#12714=CARTESIAN_POINT ( 'NONE',  ( 104.9957702545248566, 0.1403307496149616695, -11.32035403202665336 ) ) ;
#12720=VERTEX_POINT ( 'NONE', #40306 ) ;
#12723=CARTESIAN_POINT ( 'NONE',  ( 116.4555358795247884, -8.402594152722688392, -9.854619843455216355 ) ) ;
#12728=CARTESIAN_POINT ( 'NONE',  ( 115.3442858795247759, -0.7896495226426338832, -17.46756447353520159 ) ) ;
#12729=CARTESIAN_POINT ( 'NONE',  ( 109.9269421295247753, -9.868328341294093420, -13.39321520033831447 ) ) ;
#12730=CARTESIAN_POINT ( 'NONE',  ( 83.14901522432917602, -31.89413582345784803, -23.38874658933293560 ) ) ;
#12735=CARTESIAN_POINT ( 'NONE',  ( 114.2330358795247776, -8.402594152722688392, -9.854619843455216355 ) ) ;
#12744=CARTESIAN_POINT ( 'NONE',  ( 116.9654664325269238, -11.55218184020096395, -21.57977077210596306 ) ) ;
#12753=CARTESIAN_POINT ( 'NONE',  ( 110.8298327545248299, -6.936859964151250502, -8.388885654883777576 ) ) ;
#12767=CARTESIAN_POINT ( 'NONE',  ( 110.3436608795247764, -1.325403438956436419, -16.93181055722137174 ) ) ;
#12783=CARTESIAN_POINT ( 'NONE',  ( 110.4825671295247815, -10.62599879583958540, -13.39321520033831447 ) ) ;
#12785=CARTESIAN_POINT ( 'NONE',  ( 105.9681140045248355, 0.1403307496149616695, -15.46607636864997204 ) ) ;
#12786=CARTESIAN_POINT ( 'NONE',  ( 107.6349890045248401, -9.868328341294098749, -11.32035403202665869 ) ) ;
#12789=ORIENTED_EDGE ( 'NONE', *, *, #20009, .T. ) ;
#12790=CARTESIAN_POINT ( 'NONE',  ( 77.77634386988383142, 3.254514819260860392, -4.893215200338314474 ) ) ;
#12794=CARTESIAN_POINT ( 'NONE',  ( 107.0099108795247815, -1.325403438956436419, -16.93181055722141792 ) ) ;
#12797=CARTESIAN_POINT ( 'NONE',  ( 107.8433483795247838, -0.7896495226426338832, -9.318865927141430916 ) ) ;
#12799=AXIS2_PLACEMENT_3D ( 'NONE', #1697, #14946, #29523 ) ;
#12800=EDGE_LOOP ( 'NONE', ( #17293, #17160, #29262 ) ) ;
#12811=ADVANCED_FACE ( 'NONE', ( #7836 ), #21516, .T. ) ;
#12821=CARTESIAN_POINT ( 'NONE',  ( 112.9828796295247884, -4.863998795839590272, -19.15521520033831493 ) ) ;
#12824=VERTEX_POINT ( 'NONE', #4408 ) ;
#12832=CARTESIAN_POINT ( 'NONE',  ( 108.7462390045248242, 0.8980012041604421569, -15.77991374673208469 ) ) ;
#12839=AXIS2_PLACEMENT_3D ( 'NONE', #35163, #28581, #7826 ) ;
#12843=CARTESIAN_POINT ( 'NONE',  ( 114.5108483795247878, -0.7896495226426338832, -9.318865927141430916 ) ) ;
#12844=CARTESIAN_POINT ( 'NONE',  ( 111.7327233795247849, -1.325403438956436419, -9.854619843455211026 ) ) ;
#12845=CARTESIAN_POINT ( 'NONE',  ( 111.5938171295247940, -10.62599879583958540, -13.39321520033831447 ) ) ;
#12846=AXIS2_PLACEMENT_3D ( 'NONE', #26201, #4766, #36225 ) ;
#12848=VERTEX_POINT ( 'NONE', #18323 ) ;
#12850=DIRECTION ( 'NONE',  ( 1.000000000000000000, 0.000000000000000000, 0.000000000000000000 ) ) ;
#12851=CARTESIAN_POINT ( 'NONE',  ( 65.08556096878474762, -20.51665340220043277, -5.893215200338312698 ) ) ;
#12863=CARTESIAN_POINT ( 'NONE',  ( 109.3713171295247832, 0.1403307496149613920, -13.39321520033831447 ) ) ;
#12864=CARTESIAN_POINT ( 'NONE',  ( 112.0799890045248475, -9.868328341294098749, -11.32035403202665869 ) ) ;
#12866=CARTESIAN_POINT ( 'NONE',  ( 64.17717360238856372, -55.76310523276723075, -40.89321520033833224 ) ) ;
#12867=CARTESIAN_POINT ( 'NONE',  ( 68.68839935636917460, -25.95913848132418522, -5.893215200338315363 ) ) ;
#12870=ADVANCED_FACE ( 'NONE', ( #24707 ), #23521, .T. ) ;
#12882=ADVANCED_FACE ( 'NONE', ( #16657 ), #37836, .F. ) ;
#12883=CARTESIAN_POINT ( 'NONE',  ( 105.9681140045248355, -10.62599879583958717, -11.00651665394454604 ) ) ;
#12886=DIRECTION ( 'NONE',  ( 0.000000000000000000, 0.000000000000000000, 1.000000000000000000 ) ) ;
#12887=CARTESIAN_POINT ( 'NONE',  ( 108.2600671295247992, 0.1403307496149613920, -13.39321520033831447 ) ) ;
#12894=CARTESIAN_POINT ( 'NONE',  ( 63.69189222814998175, -62.82237896425675672, -47.71602681600972318 ) ) ;
#12904=LINE ( 'NONE', #1938, #22240 ) ;
#12906=CARTESIAN_POINT ( 'NONE',  ( 106.3848327545248651, -6.936859964151250502, -8.388885654883777576 ) ) ;
#12908=AXIS2_PLACEMENT_3D ( 'NONE', #23424, #37074, #2886 ) ;
#12911=CARTESIAN_POINT ( 'NONE',  ( 114.3719421295247827, -9.868328341294093420, -13.39321520033831447 ) ) ;
#12913=CARTESIAN_POINT ( 'NONE',  ( 63.10250807381770244, -31.76310523276724140, -23.47900163796522222 ) ) ;
#12915=CARTESIAN_POINT ( 'NONE',  ( 112.3578015045248861, -2.477300249445798297, -7.631215200338321125 ) ) ;
#12917=CARTESIAN_POINT ( 'NONE',  ( 112.4272546295247821, -4.863998795839590272, -7.631215200338315796 ) ) ;
#12932=CARTESIAN_POINT ( 'NONE',  ( 111.1076452545248259, 0.8980012041604421569, -11.00651665394454071 ) ) ;
#12935=CARTESIAN_POINT ( 'NONE',  ( 116.8512505633842835, -0.6435572107194698077, -16.52836391485888612 ) ) ;
#12942=CARTESIAN_POINT ( 'NONE',  ( 116.4006440670287219, 2.246832347042422739, -6.423500348738977017 ) ) ;
#12944=CARTESIAN_POINT ( 'NONE',  ( 108.5378796295247810, -4.863998795839590272, -8.388885654883775800 ) ) ;
#12948=EDGE_CURVE ( 'NONE', #7488, #44558, #7322, .T. ) ;
#12956=CARTESIAN_POINT ( 'NONE',  ( 114.5803015045248117, -6.936859964151250502, -18.39754474579286025 ) ) ;
#12960=CARTESIAN_POINT ( 'NONE',  ( 112.0105358795247810, -0.7896495226426338832, -17.46756447353520159 ) ) ;
#12961=CARTESIAN_POINT ( 'NONE',  ( 107.7738952545248310, -9.868328341294098749, -15.46607636864997204 ) ) ;
#12965=CARTESIAN_POINT ( 'NONE',  ( 112.9865389883689915, 0.3193521225029610777, -12.14321520033829493 ) ) ;
#12966=CARTESIAN_POINT ( 'NONE',  ( 112.5661608795247872, -1.325403438956436419, -16.93181055722141792 ) ) ;
#12968=CARTESIAN_POINT ( 'NONE',  ( 109.2295115170851716, -0.2778941975186199898, -15.60097546659909540 ) ) ;
#12975=CARTESIAN_POINT ( 'NONE',  ( 105.4124890045248293, -9.868328341294098749, -11.32035403202665869 ) ) ;
#12984=CARTESIAN_POINT ( 'NONE',  ( 112.1494421295248003, -9.868328341294093420, -13.39321520033831447 ) ) ;
#12991=ORIENTED_EDGE ( 'NONE', *, *, #1868, .F. ) ;
#13010=CARTESIAN_POINT ( 'NONE',  ( 111.8716296295247901, -4.863998795839590272, -19.15521520033831493 ) ) ;
#13016=LINE ( 'NONE', #34191, #10007 ) ;
#13022=CARTESIAN_POINT ( 'NONE',  ( 115.0664733795247798, -1.325403438956436419, -9.854619843455211026 ) ) ;
#13031=CARTESIAN_POINT ( 'NONE',  ( 78.69189222814998175, -46.76310523276723785, -23.89321520033831803 ) ) ;
#13033=ORIENTED_EDGE ( 'NONE', *, *, #36601, .T. ) ;
#13040=CARTESIAN_POINT ( 'NONE',  ( 114.2330358795247776, -0.7896495226426338832, -17.46756447353520159 ) ) ;
#13043=VERTEX_POINT ( 'NONE', #28709 ) ;
#13052=CARTESIAN_POINT ( 'NONE',  ( 108.6073327545248048, -2.477300249445798297, -19.15521520033831138 ) ) ;
#13060=CARTESIAN_POINT ( 'NONE',  ( 78.69189222814998175, -49.76310523276723785, -13.39321520033831447 ) ) ;
#13063=CARTESIAN_POINT ( 'NONE',  ( 108.6767858795247861, -0.7896495226426338832, -17.46756447353520159 ) ) ;
#13064=CARTESIAN_POINT ( 'NONE',  ( 115.5526452545247622, -9.868328341294098749, -15.46607636864997204 ) ) ;
#13065=CARTESIAN_POINT ( 'NONE',  ( 107.4266296295248821, -4.863998795839590272, -19.15521520033831493 ) ) ;
#13072=CARTESIAN_POINT ( 'NONE',  ( 65.31031011413875831, -19.24203766017952333, -5.548074201837920327 ) ) ;
#13075=EDGE_CURVE ( 'NONE', #4322, #26462, #29923, .T. ) ;
#13080=DIRECTION ( 'NONE',  ( 0.000000000000000000, 0.000000000000000000, 1.000000000000000000 ) ) ;
#13086=CARTESIAN_POINT ( 'NONE',  ( 109.5102233795247884, -1.325403438956436419, -9.854619843455211026 ) ) ;
#13087=CARTESIAN_POINT ( 'NONE',  ( 113.3995983795247895, -8.402594152722688392, -16.93181055722141792 ) ) ;
#13102=CARTESIAN_POINT ( 'NONE',  ( 106.5931921295248372, 0.8980012041604618078, -13.39321520033831447 ) ) ;
#13106=CARTESIAN_POINT ( 'NONE',  ( 111.1770983795247787, -8.402594152722688392, -16.93181055722141792 ) ) ;
#13112=ORIENTED_EDGE ( 'NONE', *, *, #39257, .T. ) ;
#13123=VECTOR ( 'NONE', #15219, 1000.000000000000000 ) ;
#13126=CARTESIAN_POINT ( 'NONE',  ( 114.5108483795247878, -0.7896495226426338832, -9.318865927141430916 ) ) ;
#13131=CARTESIAN_POINT ( 'NONE',  ( 105.4819421295248247, 0.8980012041604618078, -13.39321520033831447 ) ) ;
#13133=CARTESIAN_POINT ( 'NONE',  ( 63.10250807381770244, -31.76310523276723430, -22.89321520033831803 ) ) ;
#13135=CARTESIAN_POINT ( 'NONE',  ( 108.9545983795247821, -0.7896495226426338832, -9.318865927141430916 ) ) ;
#13137=CARTESIAN_POINT ( 'NONE',  ( 113.1912390045248031, 0.8980012041604421569, -15.77991374673208469 ) ) ;
#13140=PLANE ( 'NONE',  #21173 ) ;
#13154=VECTOR ( 'NONE', #18167, 1000.000000000000000 ) ;
#13155=CARTESIAN_POINT ( 'NONE',  ( 109.0935046295247872, -4.863998795839590272, -18.39754474579285315 ) ) ;
#13158=CARTESIAN_POINT ( 'NONE',  ( 112.0799890045248475, 0.8980012041604421569, -15.77991374673208469 ) ) ;
#13160=VECTOR ( 'NONE', #31811, 1000.000000000000114 ) ;
#13163=CARTESIAN_POINT ( 'NONE',  ( 113.1217858795247935, -8.402594152722736354, -9.854619843455244776 ) ) ;
#13165=CARTESIAN_POINT ( 'NONE',  ( 116.5169474460644494, 2.197673667592547453, -6.272794238025070079 ) ) ;
#13167=CARTESIAN_POINT ( 'NONE',  ( 107.7738952545248310, -9.868328341294098749, -15.46607636864997204 ) ) ;
#13177=ORIENTED_EDGE ( 'NONE', *, *, #27960, .F. ) ;
#13183=CARTESIAN_POINT ( 'NONE',  ( 110.4131140045248287, -10.62599879583958717, -11.00651665394454604 ) ) ;
#13184=CARTESIAN_POINT ( 'NONE',  ( 105.3430358795248338, -8.402594152722688392, -9.854619843455216355 ) ) ;
#13185=CARTESIAN_POINT ( 'NONE',  ( 116.5944421295247793, 0.8980012041604618078, -13.39321520033831447 ) ) ;
#13187=VECTOR ( 'NONE', #37511, 1000.000000000000000 ) ;
#13190=CARTESIAN_POINT ( 'NONE',  ( 113.2103884760652761, 0.6362173239733635022, -12.14321520033831625 ) ) ;
#13191=CARTESIAN_POINT ( 'NONE',  ( 113.3301452545248083, -9.868328341294098749, -15.46607636864997204 ) ) ;
#13200=CARTESIAN_POINT ( 'NONE',  ( 114.3339130180080616, 0.7607806665038616689, -14.64321520033833757 ) ) ;
#13206=B_SPLINE_CURVE_WITH_KNOTS ( 'NONE', 3,
 ( #35633, #25170, #21968, #39526 ),
 .UNSPECIFIED., .F., .F.,
 ( 4, 4 ),
 ( 0.003793286375430135211, 0.004704238447046320444 ),
 .UNSPECIFIED. ) ;
#13207=( NAMED_UNIT ( * ) SI_UNIT ( $, .STERADIAN. ) SOLID_ANGLE_UNIT ( ) );
#13211=CARTESIAN_POINT ( 'NONE',  ( 111.2465515045248168, -6.936859964151250502, -18.39754474579286025 ) ) ;
#13236=CARTESIAN_POINT ( 'NONE',  ( 105.8986608795248401, -8.938348069036489818, -9.318865927141430916 ) ) ;
#13237=CARTESIAN_POINT ( 'NONE',  ( 105.1346765045248475, -2.791137627527939813, -8.388885654883777576 ) ) ;
#13238=CARTESIAN_POINT ( 'NONE',  ( 106.4542858795248179, -8.402594152722688392, -9.854619843455216355 ) ) ;
#13249=CARTESIAN_POINT ( 'NONE',  ( 105.8292077545248446, -7.250697342233347165, -7.631215200338321125 ) ) ;
#13267=CARTESIAN_POINT ( 'NONE',  ( 111.1076452545248259, 0.8980012041604421569, -11.00651665394454071 ) ) ;
#13269=EDGE_LOOP ( 'NONE', ( #1886, #1904, #35980, #16428 ) ) ;
#13277=CARTESIAN_POINT ( 'NONE',  ( 109.2294421295247844, 0.1210096558822565393, -14.64321520034217805 ) ) ;
#13284=DIRECTION ( 'NONE',  ( -1.000000000000000000, 0.000000000000000000, 0.000000000000000000 ) ) ;
#13289=CARTESIAN_POINT ( 'NONE',  ( 108.8851452545248151, 0.8980012041604421569, -11.00651665394454071 ) ) ;
#13290=CARTESIAN_POINT ( 'NONE',  ( 112.1494421295248003, -9.868328341294093420, -13.39321520033831447 ) ) ;
#13291=CARTESIAN_POINT ( 'NONE',  ( 106.3153796295248412, -4.863998795839590272, -19.15521520033831493 ) ) ;
#13304=CARTESIAN_POINT ( 'NONE',  ( 105.4819421295248247, 0.8980012041604618078, -13.39321520033831447 ) ) ;
#13310=CARTESIAN_POINT ( 'NONE',  ( 107.5655358795247736, -8.402594152722688392, -9.854619843455216355 ) ) ;
#13311=CARTESIAN_POINT ( 'NONE',  ( 109.5796765045248122, -2.791137627527939813, -8.388885654883777576 ) ) ;
#13331=EDGE_CURVE ( 'NONE', #9856, #44074, #40873, .T. ) ;
#13334=ORIENTED_EDGE ( 'NONE', *, *, #30046, .F. ) ;
#13337=CARTESIAN_POINT ( 'NONE',  ( 116.3166296295247832, -4.863998795839590272, -19.15521520033831493 ) ) ;
#13339=CARTESIAN_POINT ( 'NONE',  ( 70.19189222814998175, -49.76310523276723785, -29.87698278062876511 ) ) ;
#13343=VERTEX_POINT ( 'NONE', #1104 ) ;
#13345=DIRECTION ( 'NONE',  ( 0.000000000000000000, 0.000000000000000000, -1.000000000000000000 ) ) ;
#13346=VECTOR ( 'NONE', #1466, 1000.000000000000114 ) ;
#13349=CARTESIAN_POINT ( 'NONE',  ( 61.27778620743471549, -25.99489077589588604, -11.39321520033831447 ) ) ;
#13355=CARTESIAN_POINT ( 'NONE',  ( 114.9970202545248412, -10.62599879583958717, -15.77991374673208469 ) ) ;
#13359=CARTESIAN_POINT ( 'NONE',  ( 114.5108483795247878, -8.402594152722688392, -16.93181055722141792 ) ) ;
#13364=CARTESIAN_POINT ( 'NONE',  ( 108.3295202545248657, -10.62599879583958717, -15.77991374673208469 ) ) ;
#13366=CARTESIAN_POINT ( 'NONE',  ( 113.7468640045248236, -10.62599879583958717, -11.00651665394454604 ) ) ;
#13369=FACE_OUTER_BOUND ( 'NONE', #21438, .T. ) ;
#13370=EDGE_CURVE ( 'NONE', #14709, #22330, #39415, .T. ) ;
#13375=AXIS2_PLACEMENT_3D ( 'NONE', #19401, #33288, #43807 ) ;
#13385=CIRCLE ( 'NONE', #25736, 5.000000000000004441 ) ;
#13387=CARTESIAN_POINT ( 'NONE',  ( 116.8455752247359953, -0.8306836925769603974, -16.75873294673692726 ) ) ;
#13388=CARTESIAN_POINT ( 'NONE',  ( 113.4690515045247992, -2.477300249445798297, -7.631215200338321125 ) ) ;
#13391=FACE_OUTER_BOUND ( 'NONE', #44259, .T. ) ;
#13395=CARTESIAN_POINT ( 'NONE',  ( 116.7494664628001004, 2.044003616876136853, -5.959107281052824057 ) ) ;
#13398=CARTESIAN_POINT ( 'NONE',  ( 105.8292077545248446, -2.791137627527939813, -18.39754474579286025 ) ) ;
#13410=CARTESIAN_POINT ( 'NONE',  ( 110.9687390045248350, 0.8980012041604421569, -15.77991374673208469 ) ) ;
#13412=CARTESIAN_POINT ( 'NONE',  ( 82.69078301141780685, -31.77851515411413885, -23.07115788542655821 ) ) ;
#13417=CYLINDRICAL_SURFACE ( 'NONE', #10917, 5.132259260909280307 ) ;
#13418=CARTESIAN_POINT ( 'NONE',  ( 109.2324108795247923, -1.325403438956436419, -16.93181055722141792 ) ) ;
#13420=CARTESIAN_POINT ( 'NONE',  ( 109.2294467943806353, -0.4195948248842314432, -15.84472584932758821 ) ) ;
#13425=ORIENTED_EDGE ( 'NONE', *, *, #41032, .F. ) ;
#13426=DIRECTION ( 'NONE',  ( 0.000000000000000000, 0.6161630946014901022, 0.7876185884367606915 ) ) ;
#13427=CARTESIAN_POINT ( 'NONE',  ( 116.8640794598117907, -11.66681915340833520, -21.47304352488360379 ) ) ;
#13436=CARTESIAN_POINT ( 'NONE',  ( 107.4266296295248821, -4.863998795839590272, -8.388885654883775800 ) ) ;
#13446=DIRECTION ( 'NONE',  ( 0.000000000000000000, 0.000000000000000000, -1.000000000000000000 ) ) ;
#13460=AXIS2_PLACEMENT_3D ( 'NONE', #11635, #42877, #35333 ) ;
#13464=CARTESIAN_POINT ( 'NONE',  ( 107.4266296295248821, -4.863998795839590272, -19.15521520033831493 ) ) ;
#13465=CARTESIAN_POINT ( 'NONE',  ( 106.1070202545248407, 0.1403307496149616695, -11.32035403202665336 ) ) ;
#13469=ORIENTED_EDGE ( 'NONE', *, *, #39772, .T. ) ;
#13470=CARTESIAN_POINT ( 'NONE',  ( 115.7097481608379894, 0.3867979994853637526, -14.64321520033831447 ) ) ;
#13475=CARTESIAN_POINT ( 'NONE',  ( 107.7044421295247929, 0.8980012041604618078, -13.39321520033831447 ) ) ;
#13488=CARTESIAN_POINT ( 'NONE',  ( 116.5960802213312775, -9.865703544234238009, -13.38317263089577480 ) ) ;
#13495=CARTESIAN_POINT ( 'NONE',  ( 108.1906140045248463, -10.62599879583958717, -11.00651665394454604 ) ) ;
#13505=CARTESIAN_POINT ( 'NONE',  ( 109.2946629278414861, 0.02815652521716283108, -14.64321520033829493 ) ) ;
#13512=ORIENTED_EDGE ( 'NONE', *, *, #16225, .T. ) ;
#13515=CARTESIAN_POINT ( 'NONE',  ( 110.1353015045248469, -2.477300249445798297, -7.631215200338321125 ) ) ;
#13516=CARTESIAN_POINT ( 'NONE',  ( 112.8439733795247832, -1.325403438956436419, -9.854619843455211026 ) ) ;
#13517=CARTESIAN_POINT ( 'NONE',  ( 107.4960827545248350, -2.477300249445798297, -19.15521520033831138 ) ) ;
#13520=ORIENTED_EDGE ( 'NONE', *, *, #34184, .F. ) ;
#13522=CARTESIAN_POINT ( 'NONE',  ( 110.8992858795247827, -0.7896495226426338832, -17.46756447353520159 ) ) ;
#13531=CARTESIAN_POINT ( 'NONE',  ( 114.1635827545248389, -6.936859964151250502, -8.388885654883777576 ) ) ;
#13536=CARTESIAN_POINT ( 'NONE',  ( 106.0375671295248310, 0.1403307496149613920, -13.39321520033831447 ) ) ;
#13537=CARTESIAN_POINT ( 'NONE',  ( 108.7462390045248242, -9.868328341294098749, -11.32035403202665869 ) ) ;
#13544=CARTESIAN_POINT ( 'NONE',  ( 61.69189222814998175, -48.76310523276723785, -23.89321520033831803 ) ) ;
#13547=ORIENTED_EDGE ( 'NONE', *, *, #37268, .F. ) ;
#13556=CARTESIAN_POINT ( 'NONE',  ( 113.9552233795247815, -8.938348069036489818, -17.46756447353520159 ) ) ;
#13565=CARTESIAN_POINT ( 'NONE',  ( 112.1874712410415924, 0.7607806665037644134, -12.14321520033829493 ) ) ;
#13567=CARTESIAN_POINT ( 'NONE',  ( 64.93843452746739331, -36.87240490544534310, -5.472084168854524755 ) ) ;
#13569=AXIS2_PLACEMENT_3D ( 'NONE', #25359, #38794, #15089 ) ;
#13571=VERTEX_POINT ( 'NONE', #43516 ) ;
#13573=CARTESIAN_POINT ( 'NONE',  ( 71.37572422742091760, -11.86958442233774313, -21.89321520033831447 ) ) ;
#13574=CARTESIAN_POINT ( 'NONE',  ( 115.5526452545247622, 0.8980012041604421569, -11.00651665394454071 ) ) ;
#13578=CARTESIAN_POINT ( 'NONE',  ( 108.8851452545248151, -9.868328341294098749, -15.46607636864997204 ) ) ;
#13580=CARTESIAN_POINT ( 'NONE',  ( 117.2294421295247844, -4.863998795839590272, -13.39321520033831447 ) ) ;
#13585=CARTESIAN_POINT ( 'NONE',  ( 110.3436608795247764, -8.938348069036489818, -9.318865927141430916 ) ) ;
#13598=ORIENTED_EDGE ( 'NONE', *, *, #19193, .T. ) ;
#13602=CARTESIAN_POINT ( 'NONE',  ( 116.8348670993032528, -1.227467558651016644, -17.16727754148226026 ) ) ;
#13603=AXIS2_PLACEMENT_3D ( 'NONE', #34199, #41303, #19860 ) ;
#13604=CARTESIAN_POINT ( 'NONE',  ( 114.5108483795247878, -0.7896495226426338832, -9.318865927141430916 ) ) ;
#13606=DIRECTION ( 'NONE',  ( 0.000000000000000000, 0.000000000000000000, -1.000000000000000000 ) ) ;
#13607=CARTESIAN_POINT ( 'NONE',  ( 113.0293531537514866, 0.4930828106260651267, -14.64321520033833579 ) ) ;
#13614=CARTESIAN_POINT ( 'NONE',  ( 107.0793640045248196, 0.1403307496149616695, -15.46607636864997204 ) ) ;
#13615=CARTESIAN_POINT ( 'NONE',  ( 77.77634386988383142, 3.254514819260860392, -21.89321520033831447 ) ) ;
#13618=EDGE_CURVE ( 'NONE', #32081, #15763, #34712, .T. ) ;
#13619=CARTESIAN_POINT ( 'NONE',  ( 115.9017791257774803, 0.2334052082820642360, -12.14321520033831625 ) ) ;
#13622=ORIENTED_EDGE ( 'NONE', *, *, #27842, .T. ) ;
#13629=CARTESIAN_POINT ( 'NONE',  ( 109.5102233795247884, -8.938348069036489818, -17.46756447353520159 ) ) ;
#13631=CARTESIAN_POINT ( 'NONE',  ( 115.1359265045248605, -7.250697342233347165, -19.15521520033831138 ) ) ;
#13637=CARTESIAN_POINT ( 'NONE',  ( 108.9545983795247821, -8.402594152722688392, -16.93181055722141792 ) ) ;
#13639=CARTESIAN_POINT ( 'NONE',  ( 78.69189222814998175, -49.76310523276723785, -40.89321520033831092 ) ) ;
#13644=EDGE_CURVE ( 'NONE', #11630, #32081, #45078, .T. ) ;
#13646=ORIENTED_EDGE ( 'NONE', *, *, #18171, .F. ) ;
#13647=CARTESIAN_POINT ( 'NONE',  ( 87.44708369096657918, -25.99489077589583630, -8.393215200338314474 ) ) ;
#13656=CARTESIAN_POINT ( 'NONE',  ( 108.4684265045247997, -2.791137627527939813, -8.388885654883777576 ) ) ;
#13658=CARTESIAN_POINT ( 'NONE',  ( 116.5944421295247793, -0.02276961308034231024, -12.14321520033831625 ) ) ;
#13664=ORIENTED_EDGE ( 'NONE', *, *, #22270, .T. ) ;
#13665=CARTESIAN_POINT ( 'NONE',  ( 114.8581140045248361, -10.62599879583958717, -11.00651665394454604 ) ) ;
#13667=CIRCLE ( 'NONE', #22404, 1.500000000000001332 ) ;
#13670=CARTESIAN_POINT ( 'NONE',  ( 78.01305443124351768, -57.59686644005601863, -1.019253850192035404 ) ) ;
#13674=CARTESIAN_POINT ( 'NONE',  ( 105.7294421295247844, -9.051693226400931991, -21.89321520033831447 ) ) ;
#13675=B_SPLINE_CURVE_WITH_KNOTS ( 'NONE', 3,
 ( #40275, #19525, #16107, #6292 ),
 .UNSPECIFIED., .F., .F.,
 ( 4, 4 ),
 ( 0.0006421114935806760109, 0.0009604418836934789901 ),
 .UNSPECIFIED. ) ;
#13680=CIRCLE ( 'NONE', #41372, 5.132259260909280307 ) ;
#13685=CARTESIAN_POINT ( 'NONE',  ( 107.4960827545248350, -2.477300249445798297, -19.15521520033831138 ) ) ;
#13687=CARTESIAN_POINT ( 'NONE',  ( 106.5931921295248372, -9.868328341294093420, -13.39321520033831447 ) ) ;
#13688=CARTESIAN_POINT ( 'NONE',  ( 69.69189222814998175, -41.76310523276723785, -47.71602681600972318 ) ) ;
#13691=CARTESIAN_POINT ( 'NONE',  ( 70.19189222814998175, -65.04786711941002864, -39.22192925581976652 ) ) ;
#13694=ADVANCED_FACE ( 'NONE', ( #2905 ), #38934, .T. ) ;
#13696=CARTESIAN_POINT ( 'NONE',  ( 115.5526452545247622, -9.868328341294098749, -15.46607636864997204 ) ) ;
#13698=VERTEX_POINT ( 'NONE', #14689 ) ;
#13704=CARTESIAN_POINT ( 'NONE',  ( 82.57348731610973402, -31.56754274340543986, -22.29195438618578606 ) ) ;
#13709=ORIENTED_EDGE ( 'NONE', *, *, #8890, .F. ) ;
#13713=ORIENTED_EDGE ( 'NONE', *, *, #22220, .F. ) ;
#13717=CARTESIAN_POINT ( 'NONE',  ( 109.2324108795247923, -8.938348069036489818, -9.318865927141430916 ) ) ;
#13727=CARTESIAN_POINT ( 'NONE',  ( 109.2620651800721845, 0.07459198820006229802, -14.64321520033832691 ) ) ;
#13728=DIRECTION ( 'NONE',  ( -1.000000000000000000, 0.000000000000000000, 0.000000000000000000 ) ) ;
#13732=DIRECTION ( 'NONE',  ( 0.000000000000000000, 0.000000000000000000, 1.000000000000000000 ) ) ;
#13738=CARTESIAN_POINT ( 'NONE',  ( 109.3018640045248304, -10.62599879583958717, -11.00651665394454604 ) ) ;
#13739=CARTESIAN_POINT ( 'NONE',  ( 110.2047546295247855, -4.863998795839590272, -18.39754474579285315 ) ) ;
#13740=CARTESIAN_POINT ( 'NONE',  ( 105.9681140045248355, -10.62599879583958717, -11.00651665394454604 ) ) ;
#13746=CARTESIAN_POINT ( 'NONE',  ( 110.4131140045248287, -10.62599879583958717, -11.00651665394454604 ) ) ;
#13753=CARTESIAN_POINT ( 'NONE',  ( 105.9681140045248355, -10.62599879583958717, -11.00651665394454604 ) ) ;
#13755=DIRECTION ( 'NONE',  ( -1.000000000000000000, 1.040834085586084059E-15, 0.000000000000000000 ) ) ;
#13758=EDGE_CURVE ( 'NONE', #10099, #37706, #32229, .T. ) ;
#13759=CARTESIAN_POINT ( 'NONE',  ( 109.1629577545248395, -2.791137627527939813, -18.39754474579286025 ) ) ;
#13760=CARTESIAN_POINT ( 'NONE',  ( 108.6073327545248048, -6.936859964151250502, -8.388885654883777576 ) ) ;
#13767=CARTESIAN_POINT ( 'NONE',  ( 115.9294421295247872, 1.035107641088057973, -4.893215200338314474 ) ) ;
#13779=CARTESIAN_POINT ( 'NONE',  ( 114.0941296295247867, -4.863998795839590272, -19.15521520033831493 ) ) ;
#13787=CARTESIAN_POINT ( 'NONE',  ( 86.51169734173754478, -25.99489077589583630, -8.393215200338314474 ) ) ;
#13790=VECTOR ( 'NONE', #33182, 1000.000000000000000 ) ;
#13796=CARTESIAN_POINT ( 'NONE',  ( 116.5944421295247793, 0.8980012041604618078, -13.39321520033831447 ) ) ;
#13801=CARTESIAN_POINT ( 'NONE',  ( 109.5102233795247884, -1.325403438956436419, -9.854619843455211026 ) ) ;
#13806=CARTESIAN_POINT ( 'NONE',  ( 108.3989733795248753, -8.938348069036489818, -17.46756447353520159 ) ) ;
#13808=CARTESIAN_POINT ( 'NONE',  ( 110.4825671295247815, -10.62599879583958540, -13.39321520033831447 ) ) ;
#13822=CARTESIAN_POINT ( 'NONE',  ( 114.5803015045248117, -2.477300249445798297, -7.631215200338321125 ) ) ;
#13824=CARTESIAN_POINT ( 'NONE',  ( 65.82164714941100669, 4.169909004287361221, -19.39321520033831447 ) ) ;
#13825=CARTESIAN_POINT ( 'NONE',  ( 55.39394582045726168, -26.25884925591183716, -19.39321520033831447 ) ) ;
#13826=LINE ( 'NONE', #37767, #36432 ) ;
#13827=CIRCLE ( 'NONE', #31296, 1.500000000000001332 ) ;
#13833=CARTESIAN_POINT ( 'NONE',  ( 114.0941296295247867, -4.863998795839590272, -8.388885654883775800 ) ) ;
#13845=CARTESIAN_POINT ( 'NONE',  ( 112.1494421295248003, 0.8980012041604618078, -13.39321520033831447 ) ) ;
#13846=CARTESIAN_POINT ( 'NONE',  ( 105.9681140045248355, 0.1403307496149616695, -15.46607636864997204 ) ) ;
#13847=CARTESIAN_POINT ( 'NONE',  ( 112.2188952545247531, 0.8980012041604421569, -11.00651665394454071 ) ) ;
#13851=FACE_OUTER_BOUND ( 'NONE', #39464, .T. ) ;
#13853=CARTESIAN_POINT ( 'NONE',  ( 107.6349890045248401, -9.868328341294098749, -11.32035403202665869 ) ) ;
#13857=CARTESIAN_POINT ( 'NONE',  ( 143.3676850761856940, -62.82237896425675672, -47.71602681600972318 ) ) ;
#13861=VERTEX_POINT ( 'NONE', #241 ) ;
#13870=ADVANCED_FACE ( 'NONE', ( #40839 ), #2244, .T. ) ;
#13871=CARTESIAN_POINT ( 'NONE',  ( 106.8015515045248378, -6.936859964151250502, -18.39754474579286025 ) ) ;
#13876=CARTESIAN_POINT ( 'NONE',  ( 64.69189222814998175, -41.76310523276723785, -19.39321520033831447 ) ) ;
#13879=CARTESIAN_POINT ( 'NONE',  ( 106.5931921295248372, -9.868328341294093420, -13.39321520033831447 ) ) ;
#13883=CYLINDRICAL_SURFACE ( 'NONE', #727, 5.000000000000006217 ) ;
#13894=AXIS2_PLACEMENT_3D ( 'NONE', #8418, #1117, #12070 ) ;
#13900=CARTESIAN_POINT ( 'NONE',  ( 116.0388171295248014, 0.1403307496149613920, -13.39321520033831447 ) ) ;
#13907=DIRECTION ( 'NONE',  ( 0.000000000000000000, 0.3713878862591638574, -0.9284778069183724503 ) ) ;
#13908=DIRECTION ( 'NONE',  ( 0.000000000000000000, 1.000000000000000000, 1.069961080215129965E-32 ) ) ;
#13910=CARTESIAN_POINT ( 'NONE',  ( 111.5938171295247940, 0.1403307496149613920, -13.39321520033831447 ) ) ;
#13925=CARTESIAN_POINT ( 'NONE',  ( 69.69189222814998175, -41.76310523276723785, -24.39321520033831447 ) ) ;
#13934=CARTESIAN_POINT ( 'NONE',  ( 109.1629577545248395, -7.250697342233347165, -7.631215200338321125 ) ) ;
#13940=FACE_OUTER_BOUND ( 'NONE', #3547, .T. ) ;
#13941=EDGE_CURVE ( 'NONE', #35613, #4412, #27066, .T. ) ;
#13951=CARTESIAN_POINT ( 'NONE',  ( 61.69189222814998175, -49.76310523276723785, -6.893215200338315363 ) ) ;
#13954=CARTESIAN_POINT ( 'NONE',  ( 116.0837272357735941, -0.01944715230183663435, -12.14321520033831625 ) ) ;
#13955=CARTESIAN_POINT ( 'NONE',  ( 109.9963952545248134, 0.8980012041604421569, -11.00651665394454071 ) ) ;
#13957=CARTESIAN_POINT ( 'NONE',  ( 110.5520202545248054, 0.1403307496149616695, -11.32035403202665336 ) ) ;
#13958=CARTESIAN_POINT ( 'NONE',  ( 106.5931921295248372, 0.8980012041604618078, -13.39321520033831447 ) ) ;
#13963=CARTESIAN_POINT ( 'NONE',  ( 113.6079577545248043, -7.250697342233347165, -7.631215200338321125 ) ) ;
#13969=CARTESIAN_POINT ( 'NONE',  ( 115.2053796295247849, -4.863998795839590272, -19.15521520033831493 ) ) ;
#13970=CARTESIAN_POINT ( 'NONE',  ( 106.8015515045248378, -2.477300249445798297, -7.631215200338321125 ) ) ;
#13971=ORIENTED_EDGE ( 'NONE', *, *, #23345, .T. ) ;
#13975=CARTESIAN_POINT ( 'NONE',  ( 114.6497546295247929, -4.863998795839590272, -7.631215200338315796 ) ) ;
#13976=CARTESIAN_POINT ( 'NONE',  ( 108.0517077545248696, -2.791137627527939813, -18.39754474579286025 ) ) ;
#13987=CARTESIAN_POINT ( 'NONE',  ( 112.0799890045248475, -9.868328341294098749, -11.32035403202665869 ) ) ;
#13989=ORIENTED_EDGE ( 'NONE', *, *, #15376, .F. ) ;
#13997=CARTESIAN_POINT ( 'NONE',  ( 114.5108483795247878, -0.7896495226426338832, -9.318865927141430916 ) ) ;
#13999=EDGE_CURVE ( 'NONE', #38298, #7297, #9803, .T. ) ;
#14003=DIRECTION ( 'NONE',  ( -1.156482317317869950E-15, -1.000000000000000000, 0.000000000000000000 ) ) ;
#14010=CARTESIAN_POINT ( 'NONE',  ( 72.75524511225664526, -29.99489077589588959, -18.39321520033831803 ) ) ;
#14013=ORIENTED_EDGE ( 'NONE', *, *, #41209, .T. ) ;
#14016=CARTESIAN_POINT ( 'NONE',  ( 110.5520202545248054, -10.62599879583958717, -15.77991374673208469 ) ) ;
#14021=CARTESIAN_POINT ( 'NONE',  ( 108.6073327545248048, -6.936859964151250502, -8.388885654883777576 ) ) ;
#14024=CARTESIAN_POINT ( 'NONE',  ( 109.2294377395977989, -7.996724596857648137, -17.72013350706484047 ) ) ;
#14026=CARTESIAN_POINT ( 'NONE',  ( 105.6903015045248253, -2.477300249445798297, -7.631215200338321125 ) ) ;
#14027=CARTESIAN_POINT ( 'NONE',  ( 115.0664733795247798, -1.325403438956436419, -9.854619843455211026 ) ) ;
#14028=CARTESIAN_POINT ( 'NONE',  ( 108.6073327545248048, -2.477300249445798297, -19.15521520033831138 ) ) ;
#14044=CARTESIAN_POINT ( 'NONE',  ( 114.2330358795247776, -0.7896495226426338832, -17.46756447353520159 ) ) ;
#14054=CARTESIAN_POINT ( 'NONE',  ( 111.3661041094426878, 0.3591747506842615789, -12.14321520033830026 ) ) ;
#14056=CARTESIAN_POINT ( 'NONE',  ( 112.9828796295247884, -4.863998795839590272, -8.388885654883775800 ) ) ;
#14069=CARTESIAN_POINT ( 'NONE',  ( 62.01216987384223955, -37.94672044352281404, -5.762757384007758610 ) ) ;
#14070=CARTESIAN_POINT ( 'NONE',  ( 112.1494421295248003, 0.8980012041604618078, -13.39321520033831447 ) ) ;
#14072=AXIS2_PLACEMENT_3D ( 'NONE', #7727, #1333, #4979 ) ;
#14074=CARTESIAN_POINT ( 'NONE',  ( 109.2293787433446539, -7.236786641593805136, -8.226045299710833092 ) ) ;
#14076=CARTESIAN_POINT ( 'NONE',  ( 109.7185827545247889, -6.936859964151250502, -8.388885654883777576 ) ) ;
#14080=CARTESIAN_POINT ( 'NONE',  ( 112.9828796295247884, -4.863998795839590272, -19.15521520033831493 ) ) ;
#14084=AXIS2_PLACEMENT_3D ( 'NONE', #23702, #27783, #37591 ) ;
#14090=CARTESIAN_POINT ( 'NONE',  ( 108.6073327545248048, -6.936859964151250502, -8.388885654883777576 ) ) ;
#14092=FACE_OUTER_BOUND ( 'NONE', #42663, .T. ) ;
#14095=B_SPLINE_CURVE_WITH_KNOTS ( 'NONE', 3,
 ( #43906, #12675, #5580, #12447, #5134, #19283, #2155, #8788, #29989, #19504 ),
 .UNSPECIFIED., .F., .F.,
 ( 4, 3, 3, 4 ),
 ( 0.000000000000000000, 0.0002476487219222810133, 0.0004952974148303710203, 0.0009534114850261840753 ),
 .UNSPECIFIED. ) ;
#14100=CARTESIAN_POINT ( 'NONE',  ( 114.3719421295247827, 0.8980012041604618078, -13.39321520033831447 ) ) ;
#14118=CARTESIAN_POINT ( 'NONE',  ( 106.5931921295248372, 0.8980012041604618078, -13.39321520033831447 ) ) ;
#14121=CARTESIAN_POINT ( 'NONE',  ( 113.2987212410415765, 0.7607806665037644134, -12.14321520033829493 ) ) ;
#14130=CARTESIAN_POINT ( 'NONE',  ( 113.6079577545248043, -2.791137627527939813, -18.39754474579286025 ) ) ;
#14132=ORIENTED_EDGE ( 'NONE', *, *, #35159, .T. ) ;
#14137=CARTESIAN_POINT ( 'NONE',  ( 83.16394245587648015, -30.76310523276723785, -21.89321520033831447 ) ) ;
#14141=CARTESIAN_POINT ( 'NONE',  ( 110.0133197905468734, 0.6938714319018670640, -12.14321520033834823 ) ) ;
#14151=CARTESIAN_POINT ( 'NONE',  ( 109.3018640045248304, -10.62599879583958717, -11.00651665394454604 ) ) ;
#14157=CARTESIAN_POINT ( 'NONE',  ( 79.40884336804893451, 5.049947642532015557, -20.47066126174475897 ) ) ;
#14160=DIRECTION ( 'NONE',  ( -1.899192652838769965E-30, -3.023161660021630136E-44, -1.000000000000000000 ) ) ;
#14172=CARTESIAN_POINT ( 'NONE',  ( 105.6903015045248253, -2.477300249445798297, -7.631215200338321125 ) ) ;
#14173=CARTESIAN_POINT ( 'NONE',  ( 107.9128015045248219, -6.936859964151250502, -18.39754474579286025 ) ) ;
#14174=CARTESIAN_POINT ( 'NONE',  ( 115.5526452545247622, -9.868328341294098749, -15.46607636864997204 ) ) ;
#14179=CARTESIAN_POINT ( 'NONE',  ( 110.1353015045248469, -2.477300249445798297, -7.631215200338321125 ) ) ;
#14186=EDGE_CURVE ( 'NONE', #13861, #9687, #26558, .T. ) ;
#14187=CARTESIAN_POINT ( 'NONE',  ( 114.8581140045248361, -10.62599879583958717, -11.00651665394454604 ) ) ;
#14188=CARTESIAN_POINT ( 'NONE',  ( 114.7192077545248594, -2.791137627527939813, -18.39754474579286025 ) ) ;
#14191=CARTESIAN_POINT ( 'NONE',  ( 109.8889130180080826, 0.7607806665037644134, -14.64321520033833579 ) ) ;
#14194=CARTESIAN_POINT ( 'NONE',  ( 113.3301452545248083, 0.8980012041604421569, -11.00651665394454071 ) ) ;
#14195=CARTESIAN_POINT ( 'NONE',  ( 105.5513952545248060, -9.868328341294098749, -15.46607636864997204 ) ) ;
#14202=EDGE_CURVE ( 'NONE', #37055, #36801, #12486, .T. ) ;
#14207=ORIENTED_EDGE ( 'NONE', *, *, #22779, .T. ) ;
#14208=CARTESIAN_POINT ( 'NONE',  ( 78.75330084444991030, 4.432659906640646241, -5.197052112444285221 ) ) ;
#14209=CARTESIAN_POINT ( 'NONE',  ( 106.1070202545248407, -10.62599879583958717, -15.77991374673208469 ) ) ;
#14210=CARTESIAN_POINT ( 'NONE',  ( 108.5378796295247810, -4.863998795839590272, -8.388885654883775800 ) ) ;
#14216=ORIENTED_EDGE ( 'NONE', *, *, #3272, .F. ) ;
#14220=CARTESIAN_POINT ( 'NONE',  ( 106.1764733795248219, -1.325403438956436419, -9.854619843455211026 ) ) ;
#14234=CARTESIAN_POINT ( 'NONE',  ( 109.9649712410415816, 0.7607806665038616689, -12.14321520033831625 ) ) ;
#14235=CARTESIAN_POINT ( 'NONE',  ( 111.1770983795247787, -0.7896495226426338832, -9.318865927141430916 ) ) ;
#14240=CARTESIAN_POINT ( 'NONE',  ( 109.7880358795247986, -8.402594152722688392, -9.854619843455216355 ) ) ;
#14243=CARTESIAN_POINT ( 'NONE',  ( 112.0593621053768771, 0.3967854368540359999, -16.28112951403851483 ) ) ;
#14244=CARTESIAN_POINT ( 'NONE',  ( 109.2294467825805526, -3.015950756132280475, -18.14724175160803554 ) ) ;
#14246=CARTESIAN_POINT ( 'NONE',  ( 108.6073327545248048, -2.477300249445798297, -19.15521520033831138 ) ) ;
#14247=CARTESIAN_POINT ( 'NONE',  ( 114.3719421295247827, -9.868328341294093420, -13.39321520033831447 ) ) ;
#14248=CARTESIAN_POINT ( 'NONE',  ( 107.6349890045248401, 0.8980012041604421569, -15.77991374673208469 ) ) ;
#14260=ORIENTED_EDGE ( 'NONE', *, *, #40083, .T. ) ;
#14266=CARTESIAN_POINT ( 'NONE',  ( 107.8433483795247838, -0.7896495226426338832, -9.318865927141430916 ) ) ;
#14267=PLANE ( 'NONE',  #42472 ) ;
#14275=CARTESIAN_POINT ( 'NONE',  ( 114.0246765045248196, -2.791137627527939813, -8.388885654883777576 ) ) ;
#14277=CARTESIAN_POINT ( 'NONE',  ( 74.69189222814998175, -41.76310523276723785, -47.71602681600972318 ) ) ;
#14287=CARTESIAN_POINT ( 'NONE',  ( 114.5803015045248117, -6.936859964151250502, -18.39754474579286025 ) ) ;
#14291=CARTESIAN_POINT ( 'NONE',  ( 85.37568467414497775, -28.74641635718726462, -9.489634795554785285 ) ) ;
#14292=CARTESIAN_POINT ( 'NONE',  ( 113.6774108795247997, -8.938348069036489818, -9.318865927141430916 ) ) ;
#14296=CARTESIAN_POINT ( 'NONE',  ( 109.2293722400885230, -3.002006214096174297, -8.219031836063955154 ) ) ;
#14298=CARTESIAN_POINT ( 'NONE',  ( 110.2047546295247855, -4.863998795839590272, -18.39754474579285315 ) ) ;
#14300=CARTESIAN_POINT ( 'NONE',  ( 116.4509667848042369, 2.225913487521071321, -20.42810828536804379 ) ) ;
#14303=CARTESIAN_POINT ( 'NONE',  ( 110.2742077545248094, -7.250697342233347165, -7.631215200338321125 ) ) ;
#14312=B_SPLINE_CURVE_WITH_KNOTS ( 'NONE', 3,
 ( #24426, #13505, #13727, #13277 ),
 .UNSPECIFIED., .F., .F.,
 ( 4, 4 ),
 ( 0.000000000000000000, 0.0001702050758941620089 ),
 .UNSPECIFIED. ) ;
#14316=CARTESIAN_POINT ( 'NONE',  ( 114.9970202545248412, -10.62599879583958717, -15.77991374673208469 ) ) ;
#14325=CARTESIAN_POINT ( 'NONE',  ( 106.2459265045248173, -2.791137627527939813, -8.388885654883777576 ) ) ;
#14327=ADVANCED_FACE ( 'NONE', ( #23141 ), #5791, .T. ) ;
#14328=CARTESIAN_POINT ( 'NONE',  ( 62.55594166779781773, -34.86283735444163767, -5.893215200338315363 ) ) ;
#14338=DIRECTION ( 'NONE',  ( -0.3445294493088594256, -0.9387755102040817867, 0.000000000000000000 ) ) ;
#14342=CARTESIAN_POINT ( 'NONE',  ( 115.2053796295247849, -4.863998795839590272, -8.388885654883775800 ) ) ;
#14352=CARTESIAN_POINT ( 'NONE',  ( 109.2294421295247844, -1.388378309844742642, -16.99368411936019641 ) ) ;
#14355=CARTESIAN_POINT ( 'NONE',  ( 113.3995983795247895, -8.402594152722688392, -16.93181055722141792 ) ) ;
#14357=ORIENTED_EDGE ( 'NONE', *, *, #18088, .F. ) ;
#14365=CARTESIAN_POINT ( 'NONE',  ( 76.69189222814998175, -49.76310523276720232, -7.393215200338315363 ) ) ;
#14366=CARTESIAN_POINT ( 'NONE',  ( 116.8928740015602870, 0.2848729546123598966, -14.64321520033831447 ) ) ;
#14369=CARTESIAN_POINT ( 'NONE',  ( 116.5966151941218811, -9.866217395151686276, -13.41088139521056988 ) ) ;
#14370=AXIS2_PLACEMENT_3D ( 'NONE', #42699, #36509, #4605 ) ;
#14376=CARTESIAN_POINT ( 'NONE',  ( 110.0658483795247804, -0.7896495226426338832, -9.318865927141430916 ) ) ;
#14378=VERTEX_POINT ( 'NONE', #36345 ) ;
#14380=CARTESIAN_POINT ( 'NONE',  ( 117.2294421295248270, 0.7813447578650477565, -4.949553853523854130 ) ) ;
#14381=CARTESIAN_POINT ( 'NONE',  ( 79.70219085298357697, 5.112903692279886947, -20.02675517807873362 ) ) ;
#14382=CIRCLE ( 'NONE', #6388, 7.132259260909282084 ) ;
#14383=LINE ( 'NONE', #10749, #2471 ) ;
#14393=ADVANCED_FACE ( 'NONE', ( #19033 ), #1696, .F. ) ;
#14394=ORIENTED_EDGE ( 'NONE', *, *, #31902, .F. ) ;
#14397=CARTESIAN_POINT ( 'NONE',  ( 112.6356140045247827, 0.1403307496149616695, -15.46607636864997204 ) ) ;
#14398=CARTESIAN_POINT ( 'NONE',  ( 109.8574890045247940, -9.868328341294098749, -11.32035403202665869 ) ) ;
#14399=CARTESIAN_POINT ( 'NONE',  ( 115.4137390045248566, -9.868328341294098749, -11.32035403202665869 ) ) ;
#14403=VERTEX_POINT ( 'NONE', #40006 ) ;
#14405=CARTESIAN_POINT ( 'NONE',  ( 111.8021765045248372, -7.250697342233347165, -19.15521520033831138 ) ) ;
#14409=CARTESIAN_POINT ( 'NONE',  ( 79.09431155867233088, 4.843896131125965177, -5.812420978032302621 ) ) ;
#14411=CARTESIAN_POINT ( 'NONE',  ( 115.7610046295247912, -4.863998795839590272, -7.631215200338315796 ) ) ;
#14412=CARTESIAN_POINT ( 'NONE',  ( 112.7745202545247878, 0.1403307496149616695, -11.32035403202665336 ) ) ;
#14417=CARTESIAN_POINT ( 'NONE',  ( 114.4413952545248350, 0.8980012041604421569, -11.00651665394454071 ) ) ;
#14422=ORIENTED_EDGE ( 'NONE', *, *, #13758, .T. ) ;
#14432=CARTESIAN_POINT ( 'NONE',  ( 108.6767858795247861, -8.402594152722688392, -9.854619843455216355 ) ) ;
#14440=ORIENTED_EDGE ( 'NONE', *, *, #30730, .T. ) ;
#14443=CARTESIAN_POINT ( 'NONE',  ( 109.5102233795247884, -8.938348069036489818, -17.46756447353520159 ) ) ;
#14454=CARTESIAN_POINT ( 'NONE',  ( 86.07942216836008242, -27.04188231690493538, -8.497324495144606971 ) ) ;
#14457=ORIENTED_EDGE ( 'NONE', *, *, #45139, .F. ) ;
#14460=CARTESIAN_POINT ( 'NONE',  ( 113.1217858795247935, -0.7896495226426338832, -17.46756447353520159 ) ) ;
#14463=PLANE ( 'NONE',  #41749 ) ;
#14465=CARTESIAN_POINT ( 'NONE',  ( 110.2742077545248094, -2.791137627527939813, -18.39754474579286025 ) ) ;
#14468=CARTESIAN_POINT ( 'NONE',  ( 109.2294421130689130, -4.116351054653907049, -18.49425727697660804 ) ) ;
#14472=CARTESIAN_POINT ( 'NONE',  ( 111.7327233795247849, -8.938348069036489818, -17.46756447353520159 ) ) ;
#14480=DIRECTION ( 'NONE',  ( 0.000000000000000000, 0.000000000000000000, 1.000000000000000000 ) ) ;
#14483=ORIENTED_EDGE ( 'NONE', *, *, #24720, .T. ) ;
#14485=EDGE_CURVE ( 'NONE', #25316, #38354, #33067, .T. ) ;
#14488=CARTESIAN_POINT ( 'NONE',  ( 108.1906140045248463, -10.62599879583958717, -11.00651665394454604 ) ) ;
#14491=CARTESIAN_POINT ( 'NONE',  ( 76.69189222814998175, -46.76310523276723785, -6.893215200338315363 ) ) ;
#14493=AXIS2_PLACEMENT_3D ( 'NONE', #43925, #29109, #43476 ) ;
#14497=EDGE_CURVE ( 'NONE', #34165, #10687, #2276, .T. ) ;
#14498=CARTESIAN_POINT ( 'NONE',  ( 112.7491510812576934, -0.01829820670803256055, -12.14321520033831625 ) ) ;
#14499=CARTESIAN_POINT ( 'NONE',  ( 115.7610046295247912, -4.863998795839590272, -18.39754474579285315 ) ) ;
#14501=EDGE_CURVE ( 'NONE', #34659, #40637, #37759, .T. ) ;
#14502=DIRECTION ( 'NONE',  ( 9.108669703179767173E-16, 0.7876185884367603585, -0.6161630946014904353 ) ) ;
#14512=CARTESIAN_POINT ( 'NONE',  ( 115.2748327545248657, -6.936859964151250502, -8.388885654883777576 ) ) ;
#14516=CARTESIAN_POINT ( 'NONE',  ( 114.9970202545248412, -10.62599879583958717, -15.77991374673208469 ) ) ;
#14519=CARTESIAN_POINT ( 'NONE',  ( 115.9947331777918862, -0.01829820670803256055, -14.64321520033831447 ) ) ;
#14520=CARTESIAN_POINT ( 'NONE',  ( 109.2294422733754828, -3.494069591452107382, -8.049094117091842193 ) ) ;
#14522=CARTESIAN_POINT ( 'NONE',  ( 113.8857702545248003, -10.62599879583958717, -15.77991374673208469 ) ) ;
#14526=CARTESIAN_POINT ( 'NONE',  ( 113.1912390045248031, 0.8980012041604421569, -15.77991374673208469 ) ) ;
#14532=VECTOR ( 'NONE', #35656, 1000.000000000000114 ) ;
#14537=CARTESIAN_POINT ( 'NONE',  ( 112.6356140045247827, -10.62599879583958717, -11.00651665394454604 ) ) ;
#14540=ORIENTED_EDGE ( 'NONE', *, *, #27375, .F. ) ;
#14546=CARTESIAN_POINT ( 'NONE',  ( 107.4266296295248821, -4.863998795839590272, -8.388885654883775800 ) ) ;
#14565=CARTESIAN_POINT ( 'NONE',  ( 115.0664733795247798, -1.325403438956436419, -9.854619843455211026 ) ) ;
#14567=CARTESIAN_POINT ( 'NONE',  ( 114.8834831777918879, -0.01829820670803256055, -14.64321520033831447 ) ) ;
#14572=AXIS2_PLACEMENT_3D ( 'NONE', #14491, #6985, #45067 ) ;
#14578=CARTESIAN_POINT ( 'NONE',  ( 111.3160046295247838, -4.863998795839590272, -18.39754474579285315 ) ) ;
#14589=CARTESIAN_POINT ( 'NONE',  ( 62.77214489637164263, -64.71164127777572617, -45.95359936387812638 ) ) ;
#14591=ORIENTED_EDGE ( 'NONE', *, *, #16104, .T. ) ;
#14592=FACE_OUTER_BOUND ( 'NONE', #7543, .T. ) ;
#14599=CARTESIAN_POINT ( 'NONE',  ( 105.4819421295248247, 0.8980012041604618078, -13.39321520033831447 ) ) ;
#14601=ORIENTED_EDGE ( 'NONE', *, *, #18077, .F. ) ;
#14602=VECTOR ( 'NONE', #39090, 1000.000000000000000 ) ;
#14620=CARTESIAN_POINT ( 'NONE',  ( 112.0991384760652920, 0.6362173239733635022, -12.14321520033831625 ) ) ;
#14621=CARTESIAN_POINT ( 'NONE',  ( 115.4137390045248566, 0.8980012041604421569, -15.77991374673208469 ) ) ;
#14622=CARTESIAN_POINT ( 'NONE',  ( 114.3024890045248156, -9.868328341294098749, -11.32035403202665869 ) ) ;
#14623=CARTESIAN_POINT ( 'NONE',  ( 112.2188952545247531, -9.868328341294098749, -15.46607636864997204 ) ) ;
#14629=CARTESIAN_POINT ( 'NONE',  ( 108.8156921295247912, 0.8980012041604618078, -13.39321520033831447 ) ) ;
#14630=DIRECTION ( 'NONE',  ( 0.000000000000000000, -1.000000000000000000, 0.000000000000000000 ) ) ;
#14635=CARTESIAN_POINT ( 'NONE',  ( 114.5108483795247878, -0.7896495226426338832, -9.318865927141430916 ) ) ;
#14636=CARTESIAN_POINT ( 'NONE',  ( 112.7050671295247923, 0.1403307496149613920, -13.39321520033831447 ) ) ;
#14650=LINE ( 'NONE', #4602, #1099 ) ;
#14653=CARTESIAN_POINT ( 'NONE',  ( 79.05243529145373316, 4.793396140045460108, -5.736853407927685389 ) ) ;
#14655=CARTESIAN_POINT ( 'NONE',  ( 110.6214733795247867, -1.325403438956436419, -9.854619843455211026 ) ) ;
#14664=VERTEX_POINT ( 'NONE', #29102 ) ;
#14667=CARTESIAN_POINT ( 'NONE',  ( 112.7050671295247923, -10.62599879583958540, -13.39321520033831447 ) ) ;
#14668=VECTOR ( 'NONE', #28098, 1000.000000000000000 ) ;
#14676=CARTESIAN_POINT ( 'NONE',  ( 115.0664733795247798, -8.938348069036489818, -17.46756447353520159 ) ) ;
#14683=CARTESIAN_POINT ( 'NONE',  ( 110.8298327545248299, -2.477300249445798297, -19.15521520033831138 ) ) ;
#14687=ADVANCED_FACE ( 'NONE', ( #28887 ), #42153, .T. ) ;
#14688=DIRECTION ( 'NONE',  ( 0.000000000000000000, 0.000000000000000000, -1.000000000000000000 ) ) ;
#14689=CARTESIAN_POINT ( 'NONE',  ( 70.19189222814998175, -66.20485342690169261, -45.06987807991856698 ) ) ;
#14692=CARTESIAN_POINT ( 'NONE',  ( 109.2294433289797126, -3.066010384757168250, -18.16908882001265368 ) ) ;
#14693=AXIS2_PLACEMENT_3D ( 'NONE', #10735, #37862, #17135 ) ;
#14696=CARTESIAN_POINT ( 'NONE',  ( 116.1777233795247781, -1.325403438956436419, -9.854619843455211026 ) ) ;
#14697=CARTESIAN_POINT ( 'NONE',  ( 106.1764733795248219, -8.938348069036489818, -17.46756447353520159 ) ) ;
#14703=VERTEX_POINT ( 'NONE', #39816 ) ;
#14705=AXIS2_PLACEMENT_3D ( 'NONE', #37438, #9635, #6209 ) ;
#14706=CARTESIAN_POINT ( 'NONE',  ( 61.69189222814998175, -49.76310523276723785, -19.39321520033831447 ) ) ;
#14709=VERTEX_POINT ( 'NONE', #43469 ) ;
#14710=EDGE_CURVE ( 'NONE', #36696, #20709, #15922, .T. ) ;
#14713=ADVANCED_FACE ( 'NONE', ( #25467 ), #20590, .T. ) ;
#14716=CARTESIAN_POINT ( 'NONE',  ( 110.3436608795247764, -8.938348069036489818, -9.318865927141430916 ) ) ;
#14718=CARTESIAN_POINT ( 'NONE',  ( 116.8449686807541781, 0.3528313838059640717, -14.64321520033831447 ) ) ;
#14719=CARTESIAN_POINT ( 'NONE',  ( 112.9828796295247884, -4.863998795839590272, -8.388885654883775800 ) ) ;
#14725=CARTESIAN_POINT ( 'NONE',  ( 112.2883483795247770, -8.402594152722688392, -16.93181055722141792 ) ) ;
#14729=VECTOR ( 'NONE', #29627, 1000.000000000000000 ) ;
#14730=LINE ( 'NONE', #7652, #35474 ) ;
#14735=VERTEX_POINT ( 'NONE', #28559 ) ;
#14738=CARTESIAN_POINT ( 'NONE',  ( 112.9828796295247884, -4.863998795839590272, -8.388885654883775800 ) ) ;
#14742=ADVANCED_FACE ( 'NONE', ( #11229 ), #32407, .F. ) ;
#14743=CARTESIAN_POINT ( 'NONE',  ( 85.09674465308115998, -29.42238801905354251, -10.32662417038046954 ) ) ;
#14744=CARTESIAN_POINT ( 'NONE',  ( 113.5385046295247804, -4.863998795839590272, -7.631215200338315796 ) ) ;
#14748=CARTESIAN_POINT ( 'NONE',  ( 109.2294401788930998, -1.084644456222203290, -9.551446960330030933 ) ) ;
#14750=CARTESIAN_POINT ( 'NONE',  ( 106.8015515045248378, -6.936859964151250502, -18.39754474579286025 ) ) ;
#14751=DIRECTION ( 'NONE',  ( 0.9659258262890689783, 0.2588190451025180194, 0.000000000000000000 ) ) ;
#14754=CARTESIAN_POINT ( 'NONE',  ( 110.0658483795247804, -0.7896495226426338832, -9.318865927141430916 ) ) ;
#14761=EDGE_CURVE ( 'NONE', #30697, #11967, #29900, .T. ) ;
#14767=CARTESIAN_POINT ( 'NONE',  ( 115.2748327545248657, -2.477300249445798297, -19.15521520033831138 ) ) ;
#14782=AXIS2_PLACEMENT_3D ( 'NONE', #2288, #16442, #44266 ) ;
#14790=DIRECTION ( 'NONE',  ( 1.000000000000000000, 0.000000000000000000, 0.000000000000000000 ) ) ;
#14794=CARTESIAN_POINT ( 'NONE',  ( 113.9552233795247815, -1.325403438956436419, -9.854619843455211026 ) ) ;
#14796=AXIS2_PLACEMENT_3D ( 'NONE', #13824, #30930, #13606 ) ;
#14806=CARTESIAN_POINT ( 'NONE',  ( 70.19189222814998175, -49.76310523276723785, -36.33917278160906505 ) ) ;
#14807=CARTESIAN_POINT ( 'NONE',  ( 114.3024890045248156, -9.868328341294098749, -11.32035403202665869 ) ) ;
#14818=CARTESIAN_POINT ( 'NONE',  ( 63.38258667102197563, -64.24438017783141674, -46.60357888607674681 ) ) ;
#14835=CARTESIAN_POINT ( 'NONE',  ( 69.69189222814998175, -41.76310523276723785, -24.89321520033831447 ) ) ;
#14839=FACE_OUTER_BOUND ( 'NONE', #7353, .T. ) ;
#14840=CARTESIAN_POINT ( 'NONE',  ( 70.19189222814998175, -49.76310523276723785, -29.87698278062876511 ) ) ;
#14844=CARTESIAN_POINT ( 'NONE',  ( 116.6769462226555163, -8.438241265790122014, -17.00663296034464267 ) ) ;
#14853=CARTESIAN_POINT ( 'NONE',  ( 105.5513952545248060, 0.8980012041604421569, -11.00651665394454071 ) ) ;
#14854=CARTESIAN_POINT ( 'NONE',  ( 111.5243640045248412, 0.1403307496149616695, -15.46607636864997204 ) ) ;
#14857=EDGE_LOOP ( 'NONE', ( #26723, #38142 ) ) ;
#14859=CARTESIAN_POINT ( 'NONE',  ( 105.6208483795248299, -0.7896495226426338832, -9.318865927141430916 ) ) ;
#14861=DIRECTION ( 'NONE',  ( 0.000000000000000000, 0.000000000000000000, -1.000000000000000000 ) ) ;
#14865=CARTESIAN_POINT ( 'NONE',  ( 113.8857702545248003, -10.62599879583958717, -15.77991374673208469 ) ) ;
#14866=CARTESIAN_POINT ( 'NONE',  ( 111.1770983795247787, -8.402594152722688392, -16.93181055722141792 ) ) ;
#14867=ORIENTED_EDGE ( 'NONE', *, *, #8324, .F. ) ;
#14880=ORIENTED_EDGE ( 'NONE', *, *, #7203, .F. ) ;
#14884=CARTESIAN_POINT ( 'NONE',  ( 116.3860827545247787, -2.477300249445798297, -19.15521520033831138 ) ) ;
#14895=CARTESIAN_POINT ( 'NONE',  ( 110.8298327545248299, -2.477300249445798297, -19.15521520033831138 ) ) ;
#14897=DIRECTION ( 'NONE',  ( 0.000000000000000000, 0.000000000000000000, -1.000000000000000000 ) ) ;
#14900=CARTESIAN_POINT ( 'NONE',  ( 143.3676850761856940, -55.76310523276723785, -40.89321520033831092 ) ) ;
#14906=CARTESIAN_POINT ( 'NONE',  ( 115.6220983795247861, -0.7896495226426338832, -9.318865927141430916 ) ) ;
#14911=CARTESIAN_POINT ( 'NONE',  ( 112.5661608795247872, -8.938348069036489818, -9.318865927141430916 ) ) ;
#14917=DIRECTION ( 'NONE',  ( 0.000000000000000000, 0.000000000000000000, -1.000000000000000000 ) ) ;
#14918=VERTEX_POINT ( 'NONE', #15998 ) ;
#14919=CARTESIAN_POINT ( 'NONE',  ( 116.3166296295247832, -4.863998795839590272, -19.15521520033831493 ) ) ;
#14920=CARTESIAN_POINT ( 'NONE',  ( 109.2295328744424125, -6.711379979716183719, -18.33685733204155355 ) ) ;
#14923=CARTESIAN_POINT ( 'NONE',  ( 114.9275671295247889, 0.1403307496149613920, -13.39321520033831447 ) ) ;
#14924=CARTESIAN_POINT ( 'NONE',  ( 106.6626452545248611, 0.8980012041604421569, -11.00651665394454071 ) ) ;
#14937=VECTOR ( 'NONE', #15502, 1000.000000000000000 ) ;
#14940=CARTESIAN_POINT ( 'NONE',  ( 108.0517077545248696, -7.250697342233347165, -7.631215200338321125 ) ) ;
#14943=CARTESIAN_POINT ( 'NONE',  ( 116.5564130180080866, 0.7607806665037644134, -14.64321520033833401 ) ) ;
#14944=CARTESIAN_POINT ( 'NONE',  ( 114.4413952545248350, -9.868328341294098749, -15.46607636864997204 ) ) ;
#14946=DIRECTION ( 'NONE',  ( 1.000000000000000000, 0.000000000000000000, 0.000000000000000000 ) ) ;
#14949=CARTESIAN_POINT ( 'NONE',  ( 112.1874712410415924, 0.7607806665037644134, -12.14321520033829493 ) ) ;
#14950=CARTESIAN_POINT ( 'NONE',  ( 108.7462390045248242, -9.868328341294098749, -11.32035403202665869 ) ) ;
#14959=CARTESIAN_POINT ( 'NONE',  ( 78.69189222814998175, -69.76310523276724496, -32.79321520033831661 ) ) ;
#14961=CARTESIAN_POINT ( 'NONE',  ( 113.9552233795247815, -1.325403438956436419, -9.854619843455211026 ) ) ;
#14964=CARTESIAN_POINT ( 'NONE',  ( 85.35964865273379587, -28.78522156022691547, -9.527126118789240650 ) ) ;
#14965=CARTESIAN_POINT ( 'NONE',  ( 109.3713171295247832, -10.62599879583958540, -13.39321520033831447 ) ) ;
#14970=CARTESIAN_POINT ( 'NONE',  ( 109.2294452810045300, -4.985890647812309062, -7.812765507842175161 ) ) ;
#14972=CARTESIAN_POINT ( 'NONE',  ( 106.3848327545248651, -6.936859964151250502, -8.388885654883777576 ) ) ;
#14973=CARTESIAN_POINT ( 'NONE',  ( 117.0710753504221060, 1.661863614013754153, -21.31253633978158035 ) ) ;
#14974=CARTESIAN_POINT ( 'NONE',  ( 82.66491059565053945, -31.44298744622023989, -22.15403020929251454 ) ) ;
#14977=CARTESIAN_POINT ( 'NONE',  ( 110.3436608795247764, -8.938348069036489818, -9.318865927141430916 ) ) ;
#14986=EDGE_CURVE ( 'NONE', #24500, #408, #23062, .T. ) ;
#14987=CARTESIAN_POINT ( 'NONE',  ( 112.7050671295247923, -10.62599879583958540, -13.39321520033831447 ) ) ;
#14990=CARTESIAN_POINT ( 'NONE',  ( 83.84865386347668448, -25.99489077589588604, -11.39321520033831447 ) ) ;
#14991=ORIENTED_EDGE ( 'NONE', *, *, #30873, .T. ) ;
#15002=CARTESIAN_POINT ( 'NONE',  ( 64.09723185476896390, -35.12832872366021775, -5.893215200338315363 ) ) ;
#15010=EDGE_CURVE ( 'NONE', #38595, #10687, #5237, .T. ) ;
#15014=LINE ( 'NONE', #35283, #8907 ) ;
#15015=EDGE_CURVE ( 'NONE', #28999, #8854, #42391, .T. ) ;
#15018=ORIENTED_EDGE ( 'NONE', *, *, #1715, .F. ) ;
#15020=CARTESIAN_POINT ( 'NONE',  ( 115.1359265045248605, -2.791137627527939813, -8.388885654883777576 ) ) ;
#15025=CARTESIAN_POINT ( 'NONE',  ( 117.0111608795247946, -1.325403438956436419, -16.93181055722141792 ) ) ;
#15026=ORIENTED_EDGE ( 'NONE', *, *, #7534, .F. ) ;
#15031=CARTESIAN_POINT ( 'NONE',  ( 106.5237390045248418, -9.868328341294098749, -11.32035403202665869 ) ) ;
#15053=EDGE_CURVE ( 'NONE', #8854, #28999, #35063, .T. ) ;
#15062=FACE_BOUND ( 'NONE', #32230, .T. ) ;
#15065=CARTESIAN_POINT ( 'NONE',  ( 116.6776094670037622, -8.413751147702754452, -17.03160569075142305 ) ) ;
#15067=CARTESIAN_POINT ( 'NONE',  ( 86.50830818076254047, -21.65036132658698520, -20.89321520033831447 ) ) ;
#15072=CARTESIAN_POINT ( 'NONE',  ( 115.7610046295247912, -4.863998795839590272, -7.631215200338315796 ) ) ;
#15073=CARTESIAN_POINT ( 'NONE',  ( 114.2330358795247776, -8.402594152722688392, -9.854619843455216355 ) ) ;
#15074=CARTESIAN_POINT ( 'NONE',  ( 115.2053796295247849, -4.863998795839590272, -8.388885654883775800 ) ) ;
#15079=CARTESIAN_POINT ( 'NONE',  ( 106.5931921295248372, 0.8980012041604618078, -13.39321520033831447 ) ) ;
#15081=EDGE_CURVE ( 'NONE', #3603, #7036, #22216, .T. ) ;
#15086=CARTESIAN_POINT ( 'NONE',  ( 110.4131140045248287, -10.62599879583958717, -11.00651665394454604 ) ) ;
#15087=CARTESIAN_POINT ( 'NONE',  ( 109.9963952545248134, -9.868328341294098749, -15.46607636864997204 ) ) ;
#15089=DIRECTION ( 'NONE',  ( 1.000000000000000000, 0.000000000000000000, 0.000000000000000000 ) ) ;
#15106=CARTESIAN_POINT ( 'NONE',  ( 116.1777233795247781, -8.938348069036489818, -17.46756447353520159 ) ) ;
#15113=CARTESIAN_POINT ( 'NONE',  ( 74.69189222814998175, -41.76310523276723785, -23.89321520033831803 ) ) ;
#15116=ORIENTED_EDGE ( 'NONE', *, *, #19193, .F. ) ;
#15118=CARTESIAN_POINT ( 'NONE',  ( 62.08082402252009757, -65.39425684394153393, -44.66980955559895961 ) ) ;
#15119=CARTESIAN_POINT ( 'NONE',  ( 110.9687390045248350, 0.8980012041604421569, -15.77991374673208469 ) ) ;
#15127=CARTESIAN_POINT ( 'NONE',  ( 116.3166296295247832, -4.863998795839590272, -19.15521520033831493 ) ) ;
#15129=CARTESIAN_POINT ( 'NONE',  ( 114.5108483795247878, -0.7896495226426338832, -9.318865927141430916 ) ) ;
#15135=CARTESIAN_POINT ( 'NONE',  ( 105.6903015045248253, -2.477300249445798297, -7.631215200338321125 ) ) ;
#15139=CARTESIAN_POINT ( 'NONE',  ( 117.1464118195297601, -11.22028320508336563, -5.522660250078516242 ) ) ;
#15143=CARTESIAN_POINT ( 'NONE',  ( 109.2292946956953159, -9.680038410784433722, -10.31160768788000937 ) ) ;
#15145=CARTESIAN_POINT ( 'NONE',  ( 112.9828796295247884, -4.863998795839590272, -8.388885654883775800 ) ) ;
#15146=CARTESIAN_POINT ( 'NONE',  ( 106.4542858795248179, -0.7896495226426338832, -17.46756447353520159 ) ) ;
#15162=DIRECTION ( 'NONE',  ( 0.000000000000000000, 0.000000000000000000, 1.000000000000000000 ) ) ;
#15164=CARTESIAN_POINT ( 'NONE',  ( 113.9552233795247815, -1.325403438956436419, -9.854619843455211026 ) ) ;
#15166=DIRECTION ( 'NONE',  ( -0.9970811988817435134, 0.07634843047859724008, 0.000000000000000000 ) ) ;
#15171=CARTESIAN_POINT ( 'NONE',  ( 112.0799890045248475, -9.868328341294098749, -11.32035403202665869 ) ) ;
#15177=B_SPLINE_CURVE_WITH_KNOTS ( 'NONE', 3,
 ( #27498, #41418, #23397, #10172, #37972, #34534, #40502, #3312, #31126, #34094 ),
 .UNSPECIFIED., .F., .F.,
 ( 4, 3, 3, 4 ),
 ( 0.000000000000000000, 0.0002476486447138720221, 0.0004952972925464089841, 0.0009604418836934709670 ),
 .UNSPECIFIED. ) ;
#15184=CARTESIAN_POINT ( 'NONE',  ( 112.2883483795247770, -8.402594152722688392, -16.93181055722141792 ) ) ;
#15188=CARTESIAN_POINT ( 'NONE',  ( 85.68405335838919257, -28.00027651839989318, -8.921533853845815543 ) ) ;
#15189=CARTESIAN_POINT ( 'NONE',  ( 109.2324108795247923, -8.938348069036489818, -9.318865927141430916 ) ) ;
#15192=DIRECTION ( 'NONE',  ( -0.7298031939408690105, -0.6836572958096084340, 0.000000000000000000 ) ) ;
#15195=CARTESIAN_POINT ( 'NONE',  ( 114.1635827545248389, -2.477300249445798297, -19.15521520033831138 ) ) ;
#15198=CARTESIAN_POINT ( 'NONE',  ( 82.47484345711939113, -31.70193537549793916, -22.53651891743845681 ) ) ;
#15201=CARTESIAN_POINT ( 'NONE',  ( 107.8433483795247838, -0.7896495226426338832, -9.318865927141430916 ) ) ;
#15204=EDGE_LOOP ( 'NONE', ( #41744, #6704, #33473, #35807 ) ) ;
#15211=CARTESIAN_POINT ( 'NONE',  ( 112.7745202545247878, -10.62599879583958717, -15.77991374673208469 ) ) ;
#15213=CARTESIAN_POINT ( 'NONE',  ( 116.8234308633710441, -1.692850972744459392, -17.55092091510499230 ) ) ;
#15215=VERTEX_POINT ( 'NONE', #231 ) ;
#15219=DIRECTION ( 'NONE',  ( -0.3445294493088594256, -0.9387755102040817867, 0.000000000000000000 ) ) ;
#15220=LINE ( 'NONE', #29127, #34022 ) ;
#15224=CARTESIAN_POINT ( 'NONE',  ( 64.01282776924010420, -34.86145050234441811, -5.893215200338315363 ) ) ;
#15237=CARTESIAN_POINT ( 'NONE',  ( 109.1629577545248395, -2.791137627527939813, -18.39754474579286025 ) ) ;
#15238=CARTESIAN_POINT ( 'NONE',  ( 114.8581140045248361, 0.1403307496149616695, -15.46607636864997204 ) ) ;
#15240=CARTESIAN_POINT ( 'NONE',  ( 83.48413635955418499, -32.78863198505981558, -23.89321520033831803 ) ) ;
#15243=CARTESIAN_POINT ( 'NONE',  ( 116.3860827545247787, -6.936859964151250502, -8.388885654883777576 ) ) ;
#15250=EDGE_CURVE ( 'NONE', #25472, #18453, #19080, .T. ) ;
#15251=CARTESIAN_POINT ( 'NONE',  ( 106.7320983795247855, -8.402594152722688392, -16.93181055722141792 ) ) ;
#15252=ORIENTED_EDGE ( 'NONE', *, *, #15526, .T. ) ;
#15260=ORIENTED_EDGE ( 'NONE', *, *, #17247, .T. ) ;
#15267=EDGE_CURVE ( 'NONE', #8254, #27006, #32151, .T. ) ;
#15269=CARTESIAN_POINT ( 'NONE',  ( 110.9687390045248208, -9.868328341294150263, -11.32035403202671553 ) ) ;
#15274=FACE_OUTER_BOUND ( 'NONE', #2982, .T. ) ;
#15289=ORIENTED_EDGE ( 'NONE', *, *, #31486, .F. ) ;
#15291=CARTESIAN_POINT ( 'NONE',  ( 116.0388171295248014, -10.62599879583958540, -13.39321520033831447 ) ) ;
#15293=CARTESIAN_POINT ( 'NONE',  ( 110.4825671295247815, 0.1403307496149613920, -13.39321520033831447 ) ) ;
#15294=CARTESIAN_POINT ( 'NONE',  ( 108.8851452545248151, -9.868328341294098749, -15.46607636864997204 ) ) ;
#15299=CARTESIAN_POINT ( 'NONE',  ( 108.5378796295247810, -4.863998795839590272, -19.15521520033831493 ) ) ;
#15306=CARTESIAN_POINT ( 'NONE',  ( 109.3713171295247832, -10.62599879583958540, -13.39321520033831447 ) ) ;
#15307=CARTESIAN_POINT ( 'NONE',  ( 113.7468640045248236, 0.1403307496149616695, -15.46607636864997204 ) ) ;
#15308=ORIENTED_EDGE ( 'NONE', *, *, #28952, .F. ) ;
#15309=LINE ( 'NONE', #39708, #33230 ) ;
#15319=CIRCLE ( 'NONE', #19680, 15.90000000000000036 ) ;
#15327=CARTESIAN_POINT ( 'NONE',  ( 106.5237390045248418, -9.868328341294098749, -11.32035403202665869 ) ) ;
#15333=ADVANCED_FACE ( 'NONE', ( #14592 ), #35465, .T. ) ;
#15336=EDGE_LOOP ( 'NONE', ( #24663, #12156 ) ) ;
#15339=CARTESIAN_POINT ( 'NONE',  ( 111.3160046295247838, -4.863998795839590272, -7.631215200338315796 ) ) ;
#15340=CIRCLE ( 'NONE', #16798, 5.000000000000000888 ) ;
#15346=ORIENTED_EDGE ( 'NONE', *, *, #22024, .T. ) ;
#15348=B_SPLINE_CURVE_WITH_KNOTS ( 'NONE', 3,
 ( #30214, #26113, #6031, #27025, #33379, #16770, #43902, #29756, #37259, #40940, #12670, #2610, #44358, #43668, #2384, #9018, #22916, #37496 ),
 .UNSPECIFIED., .F., .F.,
 ( 4, 2, 2, 1, 1, 1, 1, 2, 2, 2, 4 ),
 ( 0.000000000000000000, 0.2500000000003136380, 0.3750000000004710121, 0.4375000000005498935, 0.4687500000005943024, 0.4843750000006165068, 0.4921875000006225020, 0.4960937500006203926, 0.5000000000006181722, 0.7500000000003090861, 1.000000000000000000 ),
 .UNSPECIFIED. ) ;
#15350=CARTESIAN_POINT ( 'NONE',  ( 112.7745202545247878, -10.62599879583958717, -15.77991374673208469 ) ) ;
#15352=CARTESIAN_POINT ( 'NONE',  ( 116.8722546295247895, -4.863998795839590272, -18.39754474579285315 ) ) ;
#15353=CARTESIAN_POINT ( 'NONE',  ( 115.4831921295247952, 0.8980012041604618078, -13.39321520033831447 ) ) ;
#15354=B_SPLINE_CURVE_WITH_KNOTS ( 'NONE', 3,
 ( #31173, #23042, #33502, #2281, #41236, #16211, #30113, #44029, #34359, #17062, #21808, #38671, #14074, #609, #7670, #7011, #828, #17941, #42346, #31840, #1054, #7901, #10660, #14970, #42565, #35472, #42794, #10882, #18164, #17490, #28882, #7221, #35702, #42122, #24780, #14520, #27992, #39134, #14296, #4477, #4247, #25006, #38900, #21585, #34795, #11104, #32061, #28433, #14748, #28660, #24564, #11327, #7438, #25237, #21359, #24345, #18397, #32290, #38230, #20920, #21134, #3578, #31388, #158, #35009, #41897 ),
 .UNSPECIFIED., .F., .F.,
 ( 4, 2, 2, 1, 1, 2, 2, 2, 2, 2, 2, 2, 1, 1, 2, 2, 2, 2, 1, 1, 2, 2, 2, 2, 2, 2, 1, 1, 1, 2, 2, 2, 2, 1, 1, 1, 2, 2, 4 ),
 ( 0.000000000000000000, 0.06249999999999879263, 0.09374999999999800160, 0.1093749999999975991, 0.1171874999999972244, 0.1210937499999972106, 0.1249999999999972106, 0.1874999999999967248, 0.2187499999999965861, 0.2499999999999963918, 0.3124999999999960587, 0.3437499999999958922, 0.3593749999999957256, 0.3671874999999955036, 0.3710937499999953926, 0.3749999999999952260, 0.4374999999999928391, 0.4687499999999916733, 0.4843749999999909517, 0.4921874999999907296, 0.4960937499999905631, 0.4999999999999904521, 0.5624999999999886757, 0.6249999999999868994, 0.6874999999999851230, 0.7187499999999844569, 0.7343749999999841238, 0.7421874999999840128, 0.7460937499999840128, 0.7480468749999841238, 0.7499999999999842348, 0.8124999999999881206, 0.8437499999999902300, 0.8593749999999914513, 0.8671874999999922284, 0.8710937499999925615, 0.8730468749999927836, 0.8749999999999930056, 1.000000000000000000 ),
 .UNSPECIFIED. ) ;
#15357=AXIS2_PLACEMENT_3D ( 'NONE', #27765, #15756, #27545 ) ;
#15360=CARTESIAN_POINT ( 'NONE',  ( 108.8851452545248151, 0.8980012041604421569, -11.00651665394454071 ) ) ;
#15365=CARTESIAN_POINT ( 'NONE',  ( 117.0279894963340865, -11.45915905890350928, -5.771967884200551069 ) ) ;
#15368=CARTESIAN_POINT ( 'NONE',  ( 109.2294433043877575, -8.944666232049794274, -16.92356842977666886 ) ) ;
#15370=CARTESIAN_POINT ( 'NONE',  ( 111.7327233795247849, -1.325403438956436419, -9.854619843455211026 ) ) ;
#15371=CARTESIAN_POINT ( 'NONE',  ( 105.8292077545248446, -7.250697342233347165, -7.631215200338321125 ) ) ;
#15376=EDGE_CURVE ( 'NONE', #2865, #35384, #21271, .T. ) ;
#15377=VERTEX_POINT ( 'NONE', #4158 ) ;
#15385=( BOUNDED_CURVE ( )  B_SPLINE_CURVE ( 3, ( #11193, #14380, #4101, #25770 ),
 .UNSPECIFIED., .F., .F. ) 
 B_SPLINE_CURVE_WITH_KNOTS ( ( 4, 4 ),
 ( 1.159686988438800137, 1.570796326794895004 ),
 .UNSPECIFIED. ) 
 CURVE ( )  GEOMETRIC_REPRESENTATION_ITEM ( )  RATIONAL_B_SPLINE_CURVE ( ( 1.000000000000000000, 0.9859652809920760319, 0.9859652809920760319, 1.000000000000000000 ) ) 
 REPRESENTATION_ITEM ( '' )  );
#15390=CIRCLE ( 'NONE', #40889, 4.500000000000003553 ) ;
#15391=CARTESIAN_POINT ( 'NONE',  ( 64.69189222814998175, -41.76310523276723785, -20.39321520033831447 ) ) ;
#15393=CARTESIAN_POINT ( 'NONE',  ( 112.7050671295247923, 0.1403307496149613920, -13.39321520033831447 ) ) ;
#15399=CARTESIAN_POINT ( 'NONE',  ( 116.9417077545247992, -2.791137627527939813, -18.39754474579286025 ) ) ;
#15400=CARTESIAN_POINT ( 'NONE',  ( 109.6491296295247793, -4.863998795839590272, -8.388885654883775800 ) ) ;
#15411=CARTESIAN_POINT ( 'NONE',  ( 110.5520202545248054, 0.1403307496149616695, -11.32035403202665336 ) ) ;
#15416=CARTESIAN_POINT ( 'NONE',  ( 108.9545983795247821, -0.7896495226426338832, -9.318865927141430916 ) ) ;
#15419=DIRECTION ( 'NONE',  ( -1.387778780781445478E-15, -1.000000000000000000, 0.000000000000000000 ) ) ;
#15422=CARTESIAN_POINT ( 'NONE',  ( 106.2459265045248173, -2.791137627527939813, -8.388885654883777576 ) ) ;
#15423=CARTESIAN_POINT ( 'NONE',  ( 70.19189222814998175, -57.62004466406306591, -36.25082616574646721 ) ) ;
#15424=CARTESIAN_POINT ( 'NONE',  ( 83.02743615869442806, -30.94908174223593633, -21.89321520033831447 ) ) ;
#15427=CARTESIAN_POINT ( 'NONE',  ( 107.3571765045248299, -7.250697342233347165, -19.15521520033831138 ) ) ;
#15431=CARTESIAN_POINT ( 'NONE',  ( 79.79010115959992788, 5.106172230548759572, -4.893215200338314474 ) ) ;
#15437=CARTESIAN_POINT ( 'NONE',  ( 110.5520202545248054, -10.62599879583958717, -15.77991374673208469 ) ) ;
#15441=CARTESIAN_POINT ( 'NONE',  ( 110.2742077545248236, -7.250697342233347165, -7.631215200338321125 ) ) ;
#15447=CARTESIAN_POINT ( 'NONE',  ( 82.92338557575642710, -31.41857578345838675, -21.89321520033831447 ) ) ;
#15450=FACE_OUTER_BOUND ( 'NONE', #43134, .T. ) ;
#15452=FACE_OUTER_BOUND ( 'NONE', #32299, .T. ) ;
#15458=SHAPE_REPRESENTATION ( 'Main Bracket', ( #12375 ), #21301 ) ;
#15463=CARTESIAN_POINT ( 'NONE',  ( 113.8163171295247764, 0.1403307496149613920, -13.39321520033831447 ) ) ;
#15467=CARTESIAN_POINT ( 'NONE',  ( 115.2053796295247849, -4.863998795839590272, -19.15521520033831493 ) ) ;
#15468=CARTESIAN_POINT ( 'NONE',  ( 109.1629577545248395, -2.791137627527939813, -18.39754474579286025 ) ) ;
#15469=CARTESIAN_POINT ( 'NONE',  ( 83.49267580666517574, -32.76310523276723785, -23.89321520033831803 ) ) ;
#15471=AXIS2_PLACEMENT_3D ( 'NONE', #37563, #34791, #24341 ) ;
#15480=CARTESIAN_POINT ( 'NONE',  ( 108.6767858795247861, -8.402594152722688392, -9.854619843455216355 ) ) ;
#15481=ORIENTED_EDGE ( 'NONE', *, *, #18083, .F. ) ;
#15490=CARTESIAN_POINT ( 'NONE',  ( 114.7886608795247696, -1.325403438956436419, -16.93181055722141792 ) ) ;
#15500=DIRECTION ( 'NONE',  ( 0.000000000000000000, 0.3713878862591642460, -0.9284778069183722282 ) ) ;
#15501=CARTESIAN_POINT ( 'NONE',  ( 109.9269421295247753, -9.868328341294093420, -13.39321520033838553 ) ) ;
#15502=DIRECTION ( 'NONE',  ( 0.000000000000000000, 0.000000000000000000, 1.000000000000000000 ) ) ;
#15510=CARTESIAN_POINT ( 'NONE',  ( 116.6078919537301033, -9.852945098058393469, -13.98784572441250162 ) ) ;
#15518=CARTESIAN_POINT ( 'NONE',  ( 110.2047546295247855, -4.863998795839590272, -18.39754474579285315 ) ) ;
#15519=CARTESIAN_POINT ( 'NONE',  ( 107.8433483795247838, -8.402594152722688392, -16.93181055722141792 ) ) ;
#15523=CARTESIAN_POINT ( 'NONE',  ( 106.9404577545248145, -7.250697342233347165, -7.631215200338321125 ) ) ;
#15525=DIRECTION ( 'NONE',  ( -1.000000000000000000, 0.000000000000000000, 0.000000000000000000 ) ) ;
#15526=EDGE_CURVE ( 'NONE', #10099, #41818, #27810, .T. ) ;
#15529=AXIS2_PLACEMENT_3D ( 'NONE', #10013, #30519, #30970 ) ;
#15530=CARTESIAN_POINT ( 'NONE',  ( 111.5938171295247940, -10.62599879583958540, -13.39321520033831447 ) ) ;
#15535=VECTOR ( 'NONE', #30961, 1000.000000000000000 ) ;
#15544=CARTESIAN_POINT ( 'NONE',  ( 113.3109957829843779, 0.6362173239733635022, -14.64321520033831447 ) ) ;
#15547=CARTESIAN_POINT ( 'NONE',  ( 110.5266510812576826, -0.01829820670803256055, -12.14321520033831625 ) ) ;
#15549=CARTESIAN_POINT ( 'NONE',  ( 115.5526452545247622, 0.8980012041604421569, -11.00651665394454071 ) ) ;
#15557=ORIENTED_EDGE ( 'NONE', *, *, #16397, .F. ) ;
#15560=CARTESIAN_POINT ( 'NONE',  ( 61.69189222814998175, -66.36873802749349238, -42.40236911872441539 ) ) ;
#15562=CARTESIAN_POINT ( 'NONE',  ( 107.3571765045248299, -7.250697342233347165, -19.15521520033831138 ) ) ;
#15573=CARTESIAN_POINT ( 'NONE',  ( 112.9134265045247645, -7.250697342233347165, -19.15521520033831138 ) ) ;
#15576=CARTESIAN_POINT ( 'NONE',  ( 111.8716296295247901, -4.863998795839590272, -19.15521520033831493 ) ) ;
#15578=ORIENTED_EDGE ( 'NONE', *, *, #21874, .T. ) ;
#15582=CARTESIAN_POINT ( 'NONE',  ( 106.1764733795248219, -8.938348069036489818, -17.46756447353520159 ) ) ;
#15584=ADVANCED_FACE ( 'NONE', ( #41883 ), #24764, .T. ) ;
#15588=CARTESIAN_POINT ( 'NONE',  ( 116.6905827088848753, -11.81713141088397379, -6.316351274785676040 ) ) ;
#15591=CARTESIAN_POINT ( 'NONE',  ( 109.2295563141408650, -10.31498796290959774, -11.96776437853030828 ) ) ;
#15593=CARTESIAN_POINT ( 'NONE',  ( 113.8163171295247764, 0.1403307496149613920, -13.39321520033831447 ) ) ;
#15594=CARTESIAN_POINT ( 'NONE',  ( 115.7610046295247912, -4.863998795839590272, -18.39754474579285315 ) ) ;
#15597=CARTESIAN_POINT ( 'NONE',  ( 71.38975968946110129, -26.28004934490193989, -5.218938316979315317 ) ) ;
#15610=CARTESIAN_POINT ( 'NONE',  ( 107.9822546295247889, -4.863998795839590272, -7.631215200338315796 ) ) ;
#15611=CARTESIAN_POINT ( 'NONE',  ( 67.69189222814998175, -59.27884951796254853, -42.87418841894956500 ) ) ;
#15612=CYLINDRICAL_SURFACE ( 'NONE', #16454, 5.000000000000004441 ) ;
#15614=CARTESIAN_POINT ( 'NONE',  ( 115.4831921295247952, -9.868328341294093420, -13.39321520033831447 ) ) ;
#15624=CARTESIAN_POINT ( 'NONE',  ( 112.0105358795247810, -8.402594152722688392, -9.854619843455216355 ) ) ;
#15637=CARTESIAN_POINT ( 'NONE',  ( 110.3436608795247764, -1.325403438956436419, -16.93181055722141792 ) ) ;
#15642=CARTESIAN_POINT ( 'NONE',  ( 110.3436608795247764, -8.938348069036489818, -9.318865927141430916 ) ) ;
#15646=CARTESIAN_POINT ( 'NONE',  ( 109.8574890045247940, 0.8980012041604421569, -15.77991374673208469 ) ) ;
#15648=CARTESIAN_POINT ( 'NONE',  ( 83.90357420486833462, -31.65026256602387633, -22.30771876464736891 ) ) ;
#15651=CARTESIAN_POINT ( 'NONE',  ( 108.6767858795247861, -0.7896495226426338832, -17.46756447353520159 ) ) ;
#15666=CARTESIAN_POINT ( 'NONE',  ( 111.1770983795247787, -0.7896495226426338832, -9.318865927141430916 ) ) ;
#15668=CARTESIAN_POINT ( 'NONE',  ( 116.7770425732746986, -3.808795826660715367, -18.46995572362991567 ) ) ;
#15673=CARTESIAN_POINT ( 'NONE',  ( 70.19189222814998175, -66.20485342690169261, -45.06987807991856698 ) ) ;
#15677=DIRECTION ( 'NONE',  ( 0.000000000000000000, 1.000000000000000000, 0.000000000000000000 ) ) ;
#15678=CARTESIAN_POINT ( 'NONE',  ( 64.24559192882155401, -35.37386509779257437, -5.871741255084225841 ) ) ;
#15691=CARTESIAN_POINT ( 'NONE',  ( 112.9828796295247884, -4.863998795839590272, -8.388885654883775800 ) ) ;
#15695=CARTESIAN_POINT ( 'NONE',  ( 115.5526452545247622, 0.8980012041604421569, -11.00651665394454071 ) ) ;
#15696=CARTESIAN_POINT ( 'NONE',  ( 107.9822546295247889, -4.863998795839590272, -18.39754474579285315 ) ) ;
#15707=CARTESIAN_POINT ( 'NONE',  ( 107.9822546295247889, -4.863998795839590272, -18.39754474579285315 ) ) ;
#15718=CARTESIAN_POINT ( 'NONE',  ( 110.3436608795247764, -1.325403438956436419, -16.93181055722141792 ) ) ;
#15731=CARTESIAN_POINT ( 'NONE',  ( 109.8574890045248367, -9.868328341294150263, -11.32035403202669777 ) ) ;
#15735=CARTESIAN_POINT ( 'NONE',  ( 69.69189222814998175, -41.76310523276723785, -24.39321520033831447 ) ) ;
#15740=CARTESIAN_POINT ( 'NONE',  ( 116.6027202256327655, -9.865431707603255163, -13.72396611541779166 ) ) ;
#15747=CARTESIAN_POINT ( 'NONE',  ( 114.0941296295247867, -4.863998795839590272, -19.15521520033831493 ) ) ;
#15749=CARTESIAN_POINT ( 'NONE',  ( 110.0658483795247804, -8.402594152722688392, -16.93181055722141792 ) ) ;
#15750=CARTESIAN_POINT ( 'NONE',  ( 107.4960827545248350, -6.936859964151250502, -8.388885654883777576 ) ) ;
#15754=EDGE_LOOP ( 'NONE', ( #10535, #12632 ) ) ;
#15756=DIRECTION ( 'NONE',  ( 1.000000000000000000, 0.000000000000000000, 0.000000000000000000 ) ) ;
#15757=CYLINDRICAL_SURFACE ( 'NONE', #1569, 0.5000000000000004441 ) ;
#15761=CARTESIAN_POINT ( 'NONE',  ( 108.6767858795247861, -0.7896495226426338832, -17.46756447353520159 ) ) ;
#15763=VERTEX_POINT ( 'NONE', #43847 ) ;
#15764=CARTESIAN_POINT ( 'NONE',  ( 110.9034820646196806, 0.6269505268395592079, -14.64321520033834645 ) ) ;
#15777=CARTESIAN_POINT ( 'NONE',  ( 72.87572422742091760, -11.86958442233774313, -21.39321520033831447 ) ) ;
#15779=CARTESIAN_POINT ( 'NONE',  ( 106.8710046295248759, -4.863998795839590272, -18.39754474579285315 ) ) ;
#15781=AXIS2_PLACEMENT_3D ( 'NONE', #12003, #39812, #22479 ) ;
#15787=CIRCLE ( 'NONE', #44937, 20.00000000000000000 ) ;
#15790=CARTESIAN_POINT ( 'NONE',  ( 71.90980237029992850, -25.93883227901748967, -4.893215200338314474 ) ) ;
#15791=CARTESIAN_POINT ( 'NONE',  ( 107.4960827545248350, -2.477300249445798297, -19.15521520033831138 ) ) ;
#15800=CARTESIAN_POINT ( 'NONE',  ( 110.6214733795247867, -8.938348069036489818, -17.46756447353520159 ) ) ;
#15802=CARTESIAN_POINT ( 'NONE',  ( 113.0523327545247838, -2.477300249445798297, -19.15521520033831138 ) ) ;
#15803=AXIS2_PLACEMENT_3D ( 'NONE', #9051, #22953, #19082 ) ;
#15808=CARTESIAN_POINT ( 'NONE',  ( 108.8156921295247912, 0.8980012041604618078, -13.39321520033831447 ) ) ;
#15812=DIRECTION ( 'NONE',  ( 1.000000000000000000, 0.000000000000000000, 0.000000000000000000 ) ) ;
#15817=CARTESIAN_POINT ( 'NONE',  ( 109.2295007571409542, -9.177044000692852421, -16.67882263470107418 ) ) ;
#15819=CARTESIAN_POINT ( 'NONE',  ( 113.1217858795247935, -8.402594152722688392, -9.854619843455216355 ) ) ;
#15820=CARTESIAN_POINT ( 'NONE',  ( 112.6356140045247827, 0.1403307496149616695, -15.46607636864997204 ) ) ;
#15823=CARTESIAN_POINT ( 'NONE',  ( 69.25500790402072937, -25.95870368663648975, -5.871751884747664185 ) ) ;
#15826=ORIENTED_EDGE ( 'NONE', *, *, #341, .T. ) ;
#15833=VERTEX_POINT ( 'NONE', #19221 ) ;
#15843=EDGE_CURVE ( 'NONE', #35580, #27652, #28199, .T. ) ;
#15846=CARTESIAN_POINT ( 'NONE',  ( 111.5243640045248412, 0.1403307496149616695, -15.46607636864997204 ) ) ;
#15852=ORIENTED_EDGE ( 'NONE', *, *, #35034, .T. ) ;
#15853=CARTESIAN_POINT ( 'NONE',  ( 117.0806140045248185, 0.1403307496149616695, -15.46607636864997204 ) ) ;
#15854=CARTESIAN_POINT ( 'NONE',  ( 108.3295202545248657, 0.1403307496149616695, -11.32035403202665336 ) ) ;
#15855=AXIS2_PLACEMENT_3D ( 'NONE', #34294, #13345, #33603 ) ;
#15864=LINE ( 'NONE', #22920, #15874 ) ;
#15866=CARTESIAN_POINT ( 'NONE',  ( 110.6214733795247867, -1.325403438956436419, -9.854619843455211026 ) ) ;
#15870=CARTESIAN_POINT ( 'NONE',  ( 110.4825671295247815, -10.62599879583958540, -13.39321520033831447 ) ) ;
#15873=DIRECTION ( 'NONE',  ( 0.000000000000000000, 1.000000000000000000, 2.168404344971010101E-16 ) ) ;
#15874=VECTOR ( 'NONE', #23381, 1000.000000000000000 ) ;
#15875=CARTESIAN_POINT ( 'NONE',  ( 110.0658483795247804, -0.7896495226426338832, -9.318865927141430916 ) ) ;
#15877=CARTESIAN_POINT ( 'NONE',  ( 83.52255208528447383, -32.68847348073289538, -24.11834731266797505 ) ) ;
#15880=CARTESIAN_POINT ( 'NONE',  ( 107.9822546295247889, -4.863998795839590272, -7.631215200338315796 ) ) ;
#15894=CARTESIAN_POINT ( 'NONE',  ( 109.1629577545248395, -7.250697342233347165, -7.631215200338321125 ) ) ;
#15896=CARTESIAN_POINT ( 'NONE',  ( 84.10271796608054728, -31.10763468207608895, -20.89321520033831447 ) ) ;
#15904=CARTESIAN_POINT ( 'NONE',  ( 69.69189222814998175, -41.76310523276723785, -24.89321520033831447 ) ) ;
#15911=DIRECTION ( 'NONE',  ( 0.000000000000000000, 0.3713878862591642460, -0.9284778069183722282 ) ) ;
#15920=CARTESIAN_POINT ( 'NONE',  ( 114.7192077545248594, -2.791137627527939813, -18.39754474579286025 ) ) ;
#15922=( BOUNDED_CURVE ( )  B_SPLINE_CURVE ( 3, ( #29329, #33174, #21812, #12235 ),
 .UNSPECIFIED., .F., .T. ) 
 B_SPLINE_CURVE_WITH_KNOTS ( ( 4, 4 ),
 ( 1.570796326794895004, 1.981905665150994977 ),
 .UNSPECIFIED. ) 
 CURVE ( )  GEOMETRIC_REPRESENTATION_ITEM ( )  RATIONAL_B_SPLINE_CURVE ( ( 1.000000000000000000, 0.9859652809920760319, 0.9859652809920760319, 1.000000000000000000 ) ) 
 REPRESENTATION_ITEM ( '' )  );
#15925=CARTESIAN_POINT ( 'NONE',  ( 114.9275671295247889, -10.62599879583958540, -13.39321520033831447 ) ) ;
#15926=CARTESIAN_POINT ( 'NONE',  ( 110.0658483795247804, -8.402594152722688392, -16.93181055722141792 ) ) ;
#15930=CARTESIAN_POINT ( 'NONE',  ( 112.4272546295247821, -4.863998795839590272, -18.39754474579285315 ) ) ;
#15936=CARTESIAN_POINT ( 'NONE',  ( 78.69189222814998175, -49.76310523276723785, -24.89321520033831447 ) ) ;
#15937=CARTESIAN_POINT ( 'NONE',  ( 109.0240515045248202, -6.936859964151250502, -18.39754474579286025 ) ) ;
#15946=CARTESIAN_POINT ( 'NONE',  ( 111.5243640045248412, 0.1403307496149616695, -15.46607636864997204 ) ) ;
#15948=DIRECTION ( 'NONE',  ( -1.000000000000000000, 0.000000000000000000, 0.000000000000000000 ) ) ;
#15949=EDGE_LOOP ( 'NONE', ( #20482, #39412, #24479, #42553 ) ) ;
#15952=DIRECTION ( 'NONE',  ( 0.000000000000000000, 0.3713878862591650232, -0.9284778069183718952 ) ) ;
#15956=EDGE_CURVE ( 'NONE', #34537, #10427, #878, .T. ) ;
#15958=CARTESIAN_POINT ( 'NONE',  ( 107.2294421295247844, -9.051693226400931991, -21.39321520033831447 ) ) ;
#15959=DIRECTION ( 'NONE',  ( 0.000000000000000000, 0.000000000000000000, 1.000000000000000000 ) ) ;
#15962=CARTESIAN_POINT ( 'NONE',  ( 63.69189222814998175, -69.76310523276724496, 3.106784799661685526 ) ) ;
#15967=VECTOR ( 'NONE', #31776, 1000.000000000000000 ) ;
#15974=CARTESIAN_POINT ( 'NONE',  ( 113.3301452545248083, 0.8980012041604421569, -11.00651665394454071 ) ) ;
#15975=CARTESIAN_POINT ( 'NONE',  ( 110.2742077545248094, -2.791137627527939813, -18.39754474579286025 ) ) ;
#15976=CARTESIAN_POINT ( 'NONE',  ( 107.0099108795247815, -1.325403438956436419, -16.93181055722141792 ) ) ;
#15977=CARTESIAN_POINT ( 'NONE',  ( 64.14770544480609260, -35.52995977698498109, -5.855554904209406608 ) ) ;
#15980=CARTESIAN_POINT ( 'NONE',  ( 70.19189222814998175, -40.46710316615127567, -32.62080435916936239 ) ) ;
#15986=CARTESIAN_POINT ( 'NONE',  ( 111.3160046295247838, -4.863998795839590272, -7.631215200338315796 ) ) ;
#15998=CARTESIAN_POINT ( 'NONE',  ( 83.16394245587648015, -30.76310523276723785, -21.89321520033831447 ) ) ;
#16005=CARTESIAN_POINT ( 'NONE',  ( 112.6356140045247827, -10.62599879583958717, -11.00651665394454604 ) ) ;
#16013=DIRECTION ( 'NONE',  ( 0.000000000000000000, 1.069961080215129965E-32, -1.000000000000000000 ) ) ;
#16016=CARTESIAN_POINT ( 'NONE',  ( 105.7597546295248350, -4.863998795839590272, -7.631215200338315796 ) ) ;
#16026=CARTESIAN_POINT ( 'NONE',  ( 114.8581140045248361, -10.62599879583958717, -11.00651665394454604 ) ) ;
#16027=CARTESIAN_POINT ( 'NONE',  ( 114.3024890045248156, -9.868328341294098749, -11.32035403202665869 ) ) ;
#16028=CARTESIAN_POINT ( 'NONE',  ( 111.4549108795247747, -8.938348069036489818, -9.318865927141430916 ) ) ;
#16034=CARTESIAN_POINT ( 'NONE',  ( 106.8710046295248759, -4.863998795839590272, -7.631215200338315796 ) ) ;
#16038=CARTESIAN_POINT ( 'NONE',  ( 116.8344096179147442, -11.69876286440622692, -6.100568865546136088 ) ) ;
#16041=AXIS2_PLACEMENT_3D ( 'NONE', #832, #14751, #35932 ) ;
#16042=CARTESIAN_POINT ( 'NONE',  ( 109.2296186286734638, -9.487811336982241883, -16.25376729502801254 ) ) ;
#16045=CARTESIAN_POINT ( 'NONE',  ( 112.4272546295247821, -4.863998795839590272, -18.39754474579285315 ) ) ;
#16046=CARTESIAN_POINT ( 'NONE',  ( 110.8298327545248299, -6.936859964151250502, -8.388885654883777576 ) ) ;
#16049=CARTESIAN_POINT ( 'NONE',  ( 69.77874801882427391, -26.16868962091858464, -5.786137840895065665 ) ) ;
#16059=CARTESIAN_POINT ( 'NONE',  ( 143.3676850761856940, -69.76310523276724496, -0.9932152003383157846 ) ) ;
#16064=CARTESIAN_POINT ( 'NONE',  ( 106.8710046295248759, -4.863998795839590272, -7.631215200338315796 ) ) ;
#16067=CARTESIAN_POINT ( 'NONE',  ( 111.3160046295247838, -4.863998795839590272, -18.39754474579285315 ) ) ;
#16070=AXIS2_PLACEMENT_3D ( 'NONE', #19394, #2058, #27320 ) ;
#16074=ORIENTED_EDGE ( 'NONE', *, *, #8044, .T. ) ;
#16075=CARTESIAN_POINT ( 'NONE',  ( 117.1500671295247713, 0.1403307496149613920, -13.39321520033831447 ) ) ;
#16080=CARTESIAN_POINT ( 'NONE',  ( 79.00611218289952831, -44.99489077589586827, -23.89321520033831803 ) ) ;
#16086=CARTESIAN_POINT ( 'NONE',  ( 112.1494421295248003, -9.868328341294093420, -13.39321520033831447 ) ) ;
#16090=CARTESIAN_POINT ( 'NONE',  ( 113.4690515045247992, -6.936859964151250502, -18.39754474579286025 ) ) ;
#16092=CYLINDRICAL_SURFACE ( 'NONE', #1931, 4.999999999999997335 ) ;
#16095=CARTESIAN_POINT ( 'NONE',  ( 110.6909265045248247, -7.250697342233347165, -19.15521520033831138 ) ) ;
#16099=CARTESIAN_POINT ( 'NONE',  ( 114.3719421295247827, 0.8980012041604618078, -13.39321520033831447 ) ) ;
#16102=CARTESIAN_POINT ( 'NONE',  ( 105.8986608795248401, -8.938348069036489818, -9.318865927141430916 ) ) ;
#16104=EDGE_CURVE ( 'NONE', #25316, #16340, #42667, .T. ) ;
#16107=CARTESIAN_POINT ( 'NONE',  ( 109.3534539124563736, 0.06785227275816346770, -12.14321520033833046 ) ) ;
#16114=VECTOR ( 'NONE', #32372, 1000.000000000000114 ) ;
#16117=CARTESIAN_POINT ( 'NONE',  ( 110.9687390045248350, 0.8980012041604421569, -15.77991374673208469 ) ) ;
#16119=CARTESIAN_POINT ( 'NONE',  ( 116.8155157646764479, -2.029803478747229661, -17.78032935472251097 ) ) ;
#16128=DIRECTION ( 'NONE',  ( -1.000000000000000000, 6.760077337439384200E-16, 0.000000000000000000 ) ) ;
#16130=CARTESIAN_POINT ( 'NONE',  ( 108.1211608795247798, -1.325403438956436419, -16.93181055722141792 ) ) ;
#16134=AXIS2_PLACEMENT_3D ( 'NONE', #3686, #50, #14630 ) ;
#16143=CARTESIAN_POINT ( 'NONE',  ( 113.4690515045247992, -6.936859964151250502, -18.39754474579286025 ) ) ;
#16147=CARTESIAN_POINT ( 'NONE',  ( 114.8581140045248361, -10.62599879583958717, -11.00651665394454604 ) ) ;
#16148=CARTESIAN_POINT ( 'NONE',  ( 107.1488171295248861, 0.1403307496149613920, -13.39321520033831447 ) ) ;
#16149=CARTESIAN_POINT ( 'NONE',  ( 83.24289279524387553, -31.94143910891574123, -23.46319239529895384 ) ) ;
#16152=LINE ( 'NONE', #9533, #6592 ) ;
#16153=CARTESIAN_POINT ( 'NONE',  ( 114.0246765045248196, -2.791137627527939813, -8.388885654883777576 ) ) ;
#16155=ADVANCED_FACE ( 'NONE', ( #11653 ), #2589, .T. ) ;
#16160=ADVANCED_FACE ( 'NONE', ( #41008 ), #20916, .F. ) ;
#16167=VECTOR ( 'NONE', #38812, 1000.000000000000000 ) ;
#16171=CARTESIAN_POINT ( 'NONE',  ( 71.91396631829535124, -25.73035770285813939, -4.893215200338314474 ) ) ;
#16173=CARTESIAN_POINT ( 'NONE',  ( 114.0246765045248196, -2.791137627527939813, -8.388885654883777576 ) ) ;
#16177=ORIENTED_EDGE ( 'NONE', *, *, #21711, .T. ) ;
#16185=CARTESIAN_POINT ( 'NONE',  ( 109.7880358795247986, -8.402594152722736354, -9.854619843455244776 ) ) ;
#16198=B_SPLINE_CURVE_WITH_KNOTS ( 'NONE', 3,
 ( #25928, #29119, #33194, #8820, #15668, #22500, #36621, #29569, #12704, #40289, #1301, #33412, #32528, #2192, #30021, #16119, #9280, #23188, #43031, #15213, #37066, #30248, #6070, #17251, #6763, #10408, #23876, #34332, #13602, #20672, #45062, #27291, #41650, #41430, #44621, #33877, #3106, #40744, #13387, #44393, #12935, #41204, #2646, #16578, #31139, #10187, #24093, #23645, #37987, #34548, #17033, #9502 ),
 .UNSPECIFIED., .F., .F.,
 ( 4, 2, 2, 2, 1, 1, 2, 2, 2, 2, 2, 1, 1, 1, 2, 2, 2, 2, 1, 1, 1, 2, 2, 2, 2, 2, 1, 1, 2, 2, 4 ),
 ( 0.000000000000000000, 0.1250000000000105471, 0.1875000000000157652, 0.2187500000000184019, 0.2343750000000194844, 0.2421875000000199563, 0.2460937500000202061, 0.2500000000000204281, 0.3750000000000289213, 0.4375000000000331402, 0.4687500000000358047, 0.4843750000000378031, 0.4921875000000388023, 0.4960937500000392464, 0.4980468750000394684, 0.5000000000000396350, 0.5625000000000532907, 0.5937500000000599520, 0.6093750000000628386, 0.6171875000000638378, 0.6210937500000648370, 0.6230468750000655032, 0.6250000000000660583, 0.6875000000000504041, 0.7187500000000430767, 0.7343750000000398570, 0.7421875000000383027, 0.7460937500000374145, 0.7480468750000370814, 0.7500000000000366374, 1.000000000000000000 ),
 .UNSPECIFIED. ) ;
#16203=CARTESIAN_POINT ( 'NONE',  ( 110.5520202545248054, -10.62599879583958717, -15.77991374673208469 ) ) ;
#16204=CARTESIAN_POINT ( 'NONE',  ( 107.9128015045248219, -6.936859964151250502, -18.39754474579286025 ) ) ;
#16206=CARTESIAN_POINT ( 'NONE',  ( 109.5796765045248122, -2.791137627527939813, -8.388885654883777576 ) ) ;
#16210=CARTESIAN_POINT ( 'NONE',  ( 114.3339130180080758, 0.7607806665038616689, -14.64321520033833579 ) ) ;
#16211=CARTESIAN_POINT ( 'NONE',  ( 109.2294508954661154, -7.975540152821279705, -8.597489492498922914 ) ) ;
#16214=CARTESIAN_POINT ( 'NONE',  ( 105.6208483795248299, -8.402594152722688392, -16.93181055722141792 ) ) ;
#16216=CARTESIAN_POINT ( 'NONE',  ( 105.4819421295248247, 0.8980012041604618078, -13.39321520033831447 ) ) ;
#16217=DIRECTION ( 'NONE',  ( 0.000000000000000000, 0.3713878862591642460, -0.9284778069183722282 ) ) ;
#16225=EDGE_CURVE ( 'NONE', #1124, #16653, #20249, .T. ) ;
#16229=AXIS2_PLACEMENT_3D ( 'NONE', #24407, #17564, #31238 ) ;
#16234=ORIENTED_EDGE ( 'NONE', *, *, #6940, .F. ) ;
#16237=CARTESIAN_POINT ( 'NONE',  ( 113.8857702545248003, -10.62599879583958717, -15.77991374673208469 ) ) ;
#16239=ORIENTED_EDGE ( 'NONE', *, *, #9432, .T. ) ;
#16240=VECTOR ( 'NONE', #37535, 1000.000000000000000 ) ;
#16245=PLANE ( 'NONE',  #43990 ) ;
#16247=CARTESIAN_POINT ( 'NONE',  ( 107.5655358795247736, -0.7896495226426338832, -17.46756447353520159 ) ) ;
#16258=CARTESIAN_POINT ( 'NONE',  ( 113.8163171295247764, -10.62599879583958540, -13.39321520033831447 ) ) ;
#16260=CARTESIAN_POINT ( 'NONE',  ( 113.3301452545248083, -9.868328341294098749, -15.46607636864997204 ) ) ;
#16261=CARTESIAN_POINT ( 'NONE',  ( 109.9269421295247753, 0.8980012041604618078, -13.39321520033831447 ) ) ;
#16268=CARTESIAN_POINT ( 'NONE',  ( 61.69084222814998242, -4.863998795839590272, -13.39321520033831447 ) ) ;
#16272=VERTEX_POINT ( 'NONE', #34135 ) ;
#16273=CIRCLE ( 'NONE', #29376, 1.300000000000000044 ) ;
#16277=EDGE_CURVE ( 'NONE', #42739, #12720, #38662, .T. ) ;
#16278=CARTESIAN_POINT ( 'NONE',  ( 109.4407702545248355, 0.1403307496149616695, -11.32035403202665336 ) ) ;
#16279=CARTESIAN_POINT ( 'NONE',  ( 110.6909265045248247, -2.791137627527939813, -8.388885654883777576 ) ) ;
#16282=CARTESIAN_POINT ( 'NONE',  ( 68.68839935636917460, -25.95913848132418522, -5.893215200338315363 ) ) ;
#16292=CIRCLE ( 'NONE', #22110, 2.000000000000001776 ) ;
#16297=CARTESIAN_POINT ( 'NONE',  ( 108.2600671295247992, -10.62599879583958540, -13.39321520033831447 ) ) ;
#16301=CARTESIAN_POINT ( 'NONE',  ( 109.9963952545248134, -9.868328341294098749, -15.46607636864997204 ) ) ;
#16302=CARTESIAN_POINT ( 'NONE',  ( 109.2294421295247844, -49.76310523276723785, -19.39321520033831447 ) ) ;
#16307=CARTESIAN_POINT ( 'NONE',  ( 116.5281640045247684, -9.863998795839588496, -11.32214738847284075 ) ) ;
#16315=ORIENTED_EDGE ( 'NONE', *, *, #7152, .T. ) ;
#16318=CARTESIAN_POINT ( 'NONE',  ( 112.0799890045248475, -9.868328341294098749, -11.32035403202665869 ) ) ;
#16321=CIRCLE ( 'NONE', #27974, 2.000000000000000888 ) ;
#16323=CARTESIAN_POINT ( 'NONE',  ( 113.5385046295247804, -4.863998795839590272, -18.39754474579285315 ) ) ;
#16327=CARTESIAN_POINT ( 'NONE',  ( 110.8992858795247827, -0.7896495226426338832, -17.46756447353520159 ) ) ;
#16328=CARTESIAN_POINT ( 'NONE',  ( 114.2330358795247776, -0.7896495226426338832, -17.46756447353520159 ) ) ;
#16334=ORIENTED_EDGE ( 'NONE', *, *, #27250, .F. ) ;
#16340=VERTEX_POINT ( 'NONE', #6788 ) ;
#16343=CARTESIAN_POINT ( 'NONE',  ( 109.0240515045248202, -2.477300249445798297, -7.631215200338321125 ) ) ;
#16355=CARTESIAN_POINT ( 'NONE',  ( 108.0517077545248696, -2.791137627527939813, -18.39754474579286025 ) ) ;
#16366=CARTESIAN_POINT ( 'NONE',  ( 114.9275671295247889, 0.1403307496149613920, -13.39321520033831447 ) ) ;
#16370=CARTESIAN_POINT ( 'NONE',  ( 114.1635827545248389, -2.477300249445798297, -19.15521520033831138 ) ) ;
#16371=CARTESIAN_POINT ( 'NONE',  ( 110.3436608795247764, -1.325403438956436419, -16.93181055722141792 ) ) ;
#16372=CARTESIAN_POINT ( 'NONE',  ( 116.4555358795247884, -0.7896495226426338832, -17.46756447353520159 ) ) ;
#16377=CARTESIAN_POINT ( 'NONE',  ( 113.5385046295247804, -4.863998795839590272, -18.39754474579285315 ) ) ;
#16378=EDGE_LOOP ( 'NONE', ( #31883, #37777, #38203, #289, #13334 ) ) ;
#16379=CARTESIAN_POINT ( 'NONE',  ( 109.2296175750677918, -0.1364591305989521774, -15.31803853156103479 ) ) ;
#16386=CARTESIAN_POINT ( 'NONE',  ( 117.1051842552189868, -11.31802912314491394, -21.73478718693168688 ) ) ;
#16388=ORIENTED_EDGE ( 'NONE', *, *, #9786, .T. ) ;
#16392=FILL_AREA_STYLE_COLOUR ( '', #27134 ) ;
#16397=EDGE_CURVE ( 'NONE', #21643, #31933, #33011, .T. ) ;
#16398=CARTESIAN_POINT ( 'NONE',  ( 112.0799890045248475, -9.868328341294098749, -11.32035403202665869 ) ) ;
#16404=DIRECTION ( 'NONE',  ( 0.000000000000000000, -0.3713878862591650232, 0.9284778069183718952 ) ) ;
#16406=CIRCLE ( 'NONE', #1092, 4.500000000000003553 ) ;
#16409=CARTESIAN_POINT ( 'NONE',  ( 61.69189222814998175, -49.76310523276723785, -19.39321520033831447 ) ) ;
#16410=CARTESIAN_POINT ( 'NONE',  ( 110.4384831777918805, -0.01829820670803256055, -14.64321520033831447 ) ) ;
#16417=AXIS2_PLACEMENT_3D ( 'NONE', #13767, #3047, #17190 ) ;
#16420=FACE_OUTER_BOUND ( 'NONE', #26863, .T. ) ;
#16428=ORIENTED_EDGE ( 'NONE', *, *, #20834, .F. ) ;
#16430=CARTESIAN_POINT ( 'NONE',  ( 112.1494421295248003, 0.8980012041604618078, -13.39321520033831447 ) ) ;
#16431=CARTESIAN_POINT ( 'NONE',  ( 107.6349890045248401, -9.868328341294098749, -11.32035403202665869 ) ) ;
#16433=CARTESIAN_POINT ( 'NONE',  ( 109.7185827545248600, -2.477300249445798297, -19.15521520033832203 ) ) ;
#16436=DIRECTION ( 'NONE',  ( -0.1736481776669309696, -0.9848077530122079093, 0.000000000000000000 ) ) ;
#16441=CARTESIAN_POINT ( 'NONE',  ( 106.8710046295248759, -4.863998795839590272, -7.631215200338315796 ) ) ;
#16442=DIRECTION ( 'NONE',  ( 1.000000000000000000, 0.000000000000000000, 0.000000000000000000 ) ) ;
#16453=ORIENTED_EDGE ( 'NONE', *, *, #27284, .T. ) ;
#16454=AXIS2_PLACEMENT_3D ( 'NONE', #26328, #12886, #5788 ) ;
#16461=CARTESIAN_POINT ( 'NONE',  ( 110.8992858795247827, -0.7896495226426338832, -17.46756447353520159 ) ) ;
#16472=CARTESIAN_POINT ( 'NONE',  ( 105.6903015045248253, -2.477300249445798297, -7.631215200338321125 ) ) ;
#16480=VERTEX_POINT ( 'NONE', #36818 ) ;
#16485=CARTESIAN_POINT ( 'NONE',  ( 109.7880358795247986, -0.7896495226426338832, -17.46756447353520159 ) ) ;
#16486=CARTESIAN_POINT ( 'NONE',  ( 113.8163171295247764, 0.1403307496149613920, -13.39321520033831447 ) ) ;
#16487=CARTESIAN_POINT ( 'NONE',  ( 109.2324108795247923, -8.938348069036489818, -9.318865927141430916 ) ) ;
#16494=CARTESIAN_POINT ( 'NONE',  ( 109.2294421295247844, -8.865838614420134434, -9.247624522711900497 ) ) ;
#16506=CARTESIAN_POINT ( 'NONE',  ( 107.6349890045248401, -9.868328341294098749, -11.32035403202665869 ) ) ;
#16507=CARTESIAN_POINT ( 'NONE',  ( 110.1353015045248469, -6.936859964151250502, -18.39754474579286025 ) ) ;
#16509=CARTESIAN_POINT ( 'NONE',  ( 70.84837298282427298, -25.38184484516613892, -5.473262044462615883 ) ) ;
#16525=CARTESIAN_POINT ( 'NONE',  ( 108.3295202545248657, -10.62599879583958717, -15.77991374673208469 ) ) ;
#16527=ORIENTED_EDGE ( 'NONE', *, *, #44843, .T. ) ;
#16529=CARTESIAN_POINT ( 'NONE',  ( 107.8433483795247838, -8.402594152722688392, -16.93181055722141792 ) ) ;
#16540=VECTOR ( 'NONE', #16436, 1000.000000000000114 ) ;
#16543=CARTESIAN_POINT ( 'NONE',  ( 114.1453860982116737, 0.3867979994853637526, -12.14321520033831625 ) ) ;
#16546=EDGE_LOOP ( 'NONE', ( #20503, #19886, #23350, #36231 ) ) ;
#16548=CARTESIAN_POINT ( 'NONE',  ( 55.39394582045726168, -26.25884925591183716, -19.39321520033831447 ) ) ;
#16549=CARTESIAN_POINT ( 'NONE',  ( 116.1777233795247781, -8.938348069036489818, -17.46756447353520159 ) ) ;
#16551=AXIS2_PLACEMENT_3D ( 'NONE', #15904, #26386, #29354 ) ;
#16553=CYLINDRICAL_SURFACE ( 'NONE', #24972, 5.000000000000004441 ) ;
#16554=CARTESIAN_POINT ( 'NONE',  ( 114.6497546295247929, -4.863998795839590272, -18.39754474579285315 ) ) ;
#16558=CARTESIAN_POINT ( 'NONE',  ( 109.7185827545247889, -2.477300249445798297, -19.15521520033831138 ) ) ;
#16560=CARTESIAN_POINT ( 'NONE',  ( 115.8304577545247582, -7.250697342233347165, -7.631215200338321125 ) ) ;
#16576=CARTESIAN_POINT ( 'NONE',  ( 112.0105358795247810, -8.402594152722688392, -9.854619843455216355 ) ) ;
#16578=CARTESIAN_POINT ( 'NONE',  ( 116.8560548885474901, -0.4970007677390160805, -16.32824759579170149 ) ) ;
#16579=CARTESIAN_POINT ( 'NONE',  ( 112.1494421295248003, 0.8980012041604618078, -13.39321520033831447 ) ) ;
#16580=ORIENTED_EDGE ( 'NONE', *, *, #28718, .F. ) ;
#16583=LINE ( 'NONE', #26383, #20417 ) ;
#16584=CARTESIAN_POINT ( 'NONE',  ( 109.2294421295247844, -11.83367149576868727, -7.393215200338315363 ) ) ;
#16586=CARTESIAN_POINT ( 'NONE',  ( 117.0895350763799456, 1.621925030527854528, -5.439520474528995564 ) ) ;
#16587=CARTESIAN_POINT ( 'NONE',  ( 113.9533551332721828, 0.2334052082820642360, -14.64321520033831447 ) ) ;
#16589=CARTESIAN_POINT ( 'NONE',  ( 107.5655358795247736, -8.402594152722688392, -9.854619843455216355 ) ) ;
#16604=CARTESIAN_POINT ( 'NONE',  ( 110.2047546295247855, -4.863998795839590272, -7.631215200338315796 ) ) ;
#16605=CARTESIAN_POINT ( 'NONE',  ( 104.9263171295248327, 0.1403307496149613920, -13.39321520033831447 ) ) ;
#16606=CARTESIAN_POINT ( 'NONE',  ( 115.8304577545247582, -7.250697342233347165, -7.631215200338321125 ) ) ;
#16609=FACE_OUTER_BOUND ( 'NONE', #31325, .T. ) ;
#16610=CARTESIAN_POINT ( 'NONE',  ( 113.8163171295247764, 0.1403307496149613920, -13.39321520033831447 ) ) ;
#16611=ORIENTED_EDGE ( 'NONE', *, *, #20682, .F. ) ;
#16619=CARTESIAN_POINT ( 'NONE',  ( 104.9263171295248327, 0.1403307496149613920, -13.39321520033831447 ) ) ;
#16627=CARTESIAN_POINT ( 'NONE',  ( 109.8574890045247940, -9.868328341294098749, -11.32035403202665869 ) ) ;
#16634=CARTESIAN_POINT ( 'NONE',  ( 78.69189222814998175, -63.77884951796256274, -31.62409037935697143 ) ) ;
#16638=LINE ( 'NONE', #30308, #21609 ) ;
#16653=VERTEX_POINT ( 'NONE', #37737 ) ;
#16656=CARTESIAN_POINT ( 'NONE',  ( 113.8163171295247764, -10.62599879583958540, -13.39321520033831447 ) ) ;
#16657=FACE_OUTER_BOUND ( 'NONE', #29018, .T. ) ;
#16658=CARTESIAN_POINT ( 'NONE',  ( 62.02687168119881278, -37.86334235074598098, -5.893215200338315363 ) ) ;
#16667=CARTESIAN_POINT ( 'NONE',  ( 105.7597546295248350, -4.863998795839590272, -7.631215200338315796 ) ) ;
#16676=ADVANCED_FACE ( 'NONE', ( #41626 ), #16553, .F. ) ;
#16691=CARTESIAN_POINT ( 'NONE',  ( 110.5520202545248054, -10.62599879583958717, -15.77991374673208469 ) ) ;
#16693=ORIENTED_EDGE ( 'NONE', *, *, #14485, .F. ) ;
#16698=DIRECTION ( 'NONE',  ( -0.07634843047859724008, -0.9970811988817435134, 0.000000000000000000 ) ) ;
#16699=LINE ( 'NONE', #9860, #41816 ) ;
#16703=CARTESIAN_POINT ( 'NONE',  ( 143.3676850761856940, -82.08636712479707853, -32.64558696907351987 ) ) ;
#16715=CARTESIAN_POINT ( 'NONE',  ( 108.6073327545248048, -2.477300249445798297, -19.15521520033831138 ) ) ;
#16716=CARTESIAN_POINT ( 'NONE',  ( 113.2606921295247702, -9.868328341294093420, -13.39321520033831447 ) ) ;
#16717=CARTESIAN_POINT ( 'NONE',  ( 107.3571765045248299, -7.250697342233347165, -19.15521520033831138 ) ) ;
#16728=CARTESIAN_POINT ( 'NONE',  ( 116.5944421295247793, -4.863998795839590272, -13.39321520033831447 ) ) ;
#16729=ORIENTED_EDGE ( 'NONE', *, *, #13075, .T. ) ;
#16734=CARTESIAN_POINT ( 'NONE',  ( 108.9545983795247821, -8.402594152722688392, -16.93181055722141792 ) ) ;
#16735=CARTESIAN_POINT ( 'NONE',  ( 109.7185827545247889, -6.936859964151250502, -8.388885654883777576 ) ) ;
#16748=CARTESIAN_POINT ( 'NONE',  ( 76.69189222814998175, -49.76310523276720232, -19.39321520033831447 ) ) ;
#16754=ORIENTED_EDGE ( 'NONE', *, *, #22270, .F. ) ;
#16757=CARTESIAN_POINT ( 'NONE',  ( 107.9128015045248219, -6.936859964151250502, -18.39754474579286025 ) ) ;
#16764=CARTESIAN_POINT ( 'NONE',  ( 92.26512299712632625, -23.76310523276723785, -4.893215200338314474 ) ) ;
#16767=AXIS2_PLACEMENT_3D ( 'NONE', #38234, #23909, #16842 ) ;
#16768=LINE ( 'NONE', #24058, #24271 ) ;
#16770=CARTESIAN_POINT ( 'NONE',  ( 70.60074220370958642, -26.44921982560606466, -5.510037297638909592 ) ) ;
#16773=ORIENTED_EDGE ( 'NONE', *, *, #35878, .T. ) ;
#16776=DIRECTION ( 'NONE',  ( 0.2588190451025180749, -0.9659258262890690894, 0.000000000000000000 ) ) ;
#16777=CARTESIAN_POINT ( 'NONE',  ( 106.4542858795248179, -8.402594152722688392, -9.854619843455216355 ) ) ;
#16778=B_SPLINE_CURVE_WITH_KNOTS ( 'NONE', 3,
 ( #2290, #36271, #15764, #43578, #12348, #39931, #26701, #9370, #37161, #26025 ),
 .UNSPECIFIED., .F., .F.,
 ( 4, 3, 3, 4 ),
 ( 0.000000000000000000, 0.0002476486447138875262, 0.0004952972925464190672, 0.0009604418836934809417 ),
 .UNSPECIFIED. ) ;
#16783=CARTESIAN_POINT ( 'NONE',  ( 114.7192077545248594, -2.791137627527939813, -18.39754474579286025 ) ) ;
#16786=DIRECTION ( 'NONE',  ( 0.000000000000000000, 0.000000000000000000, -1.000000000000000000 ) ) ;
#16788=CARTESIAN_POINT ( 'NONE',  ( 114.9970202545248412, -10.62599879583958717, -15.77991374673208469 ) ) ;
#16793=FACE_OUTER_BOUND ( 'NONE', #16546, .T. ) ;
#16798=AXIS2_PLACEMENT_3D ( 'NONE', #16728, #6461, #13080 ) ;
#16806=CARTESIAN_POINT ( 'NONE',  ( 110.7603796295247918, -4.863998795839590272, -8.388885654883775800 ) ) ;
#16809=CARTESIAN_POINT ( 'NONE',  ( 111.8716296295247901, -4.863998795839590272, -19.15521520033831493 ) ) ;
#16817=CARTESIAN_POINT ( 'NONE',  ( 61.69189222814998175, -55.76310523276723785, -34.89321520033831092 ) ) ;
#16818=CARTESIAN_POINT ( 'NONE',  ( 107.0099108795247815, -1.325403438956436419, -16.93181055722141792 ) ) ;
#16829=CARTESIAN_POINT ( 'NONE',  ( 113.2226630180080775, 0.7607806665038616689, -14.64321520033831447 ) ) ;
#16832=CARTESIAN_POINT ( 'NONE',  ( 112.7745202545247878, -10.62599879583958717, -15.77991374673208469 ) ) ;
#16833=CARTESIAN_POINT ( 'NONE',  ( 104.9957702545248566, 0.1403307496149616695, -11.32035403202665336 ) ) ;
#16834=CARTESIAN_POINT ( 'NONE',  ( 116.1777233795247781, -8.938348069036489818, -17.46756447353520159 ) ) ;
#16838=CARTESIAN_POINT ( 'NONE',  ( 113.0341360982116754, 0.3867979994853637526, -12.14321520033829493 ) ) ;
#16839=CARTESIAN_POINT ( 'NONE',  ( 115.0664733795247798, -1.325403438956436419, -9.854619843455211026 ) ) ;
#16842=DIRECTION ( 'NONE',  ( 0.000000000000000000, -1.000000000000000000, 0.000000000000000000 ) ) ;
#16847=ORIENTED_EDGE ( 'NONE', *, *, #28384, .F. ) ;
#16849=CARTESIAN_POINT ( 'NONE',  ( 116.7323956815296668, -11.78763665103780944, -21.33811264340862124 ) ) ;
#16855=CARTESIAN_POINT ( 'NONE',  ( 71.67504600870660170, -26.72445618319088823, -4.893215200338314474 ) ) ;
#16858=CARTESIAN_POINT ( 'NONE',  ( 106.0375671295248310, 0.1403307496149613920, -13.39321520033831447 ) ) ;
#16861=DIRECTION ( 'NONE',  ( 0.000000000000000000, 0.000000000000000000, -1.000000000000000000 ) ) ;
#16870=DIRECTION ( 'NONE',  ( -1.000000000000000000, 0.000000000000000000, 0.000000000000000000 ) ) ;
#16886=CARTESIAN_POINT ( 'NONE',  ( 108.6767858795247861, -0.7896495226426338832, -17.46756447353520159 ) ) ;
#16887=CARTESIAN_POINT ( 'NONE',  ( 106.2459265045248173, -2.791137627527939813, -8.388885654883777576 ) ) ;
#16889=AXIS2_PLACEMENT_3D ( 'NONE', #41388, #24050, #37247 ) ;
#16890=CARTESIAN_POINT ( 'NONE',  ( 64.33603543187328455, -36.45978439725600850, -5.630764011073099873 ) ) ;
#16892=ORIENTED_EDGE ( 'NONE', *, *, #6433, .T. ) ;
#16898=CARTESIAN_POINT ( 'NONE',  ( 116.0388171295248014, 0.1403307496149613920, -13.39321520033831447 ) ) ;
#16910=ORIENTED_EDGE ( 'NONE', *, *, #7152, .F. ) ;
#16918=CARTESIAN_POINT ( 'NONE',  ( 106.5931921295248372, 0.8980012041604618078, -13.39321520033831447 ) ) ;
#16925=LINE ( 'NONE', #6876, #25069 ) ;
#16937=CARTESIAN_POINT ( 'NONE',  ( 116.0840026197984827, -0.01983013475163192263, -12.14321520033831625 ) ) ;
#16938=CARTESIAN_POINT ( 'NONE',  ( 106.7320983795247855, -0.7896495226426338832, -9.318865927141430916 ) ) ;
#16939=CARTESIAN_POINT ( 'NONE',  ( 114.0246765045248196, -2.791137627527939813, -8.388885654883777576 ) ) ;
#16940=CARTESIAN_POINT ( 'NONE',  ( 108.0517077545248696, -7.250697342233347165, -7.631215200338321125 ) ) ;
#16944=ORIENTED_EDGE ( 'NONE', *, *, #351, .T. ) ;
#16946=CARTESIAN_POINT ( 'NONE',  ( 113.5385046295247804, -4.863998795839590272, -7.631215200338315796 ) ) ;
#16954=CARTESIAN_POINT ( 'NONE',  ( 115.4831921295247952, -9.868328341294093420, -13.39321520033831447 ) ) ;
#16956=FACE_OUTER_BOUND ( 'NONE', #6871, .T. ) ;
#16960=CARTESIAN_POINT ( 'NONE',  ( 108.5378796295247810, -4.863998795839590272, -8.388885654883775800 ) ) ;
#16961=CARTESIAN_POINT ( 'NONE',  ( 107.5655358795247736, -8.402594152722688392, -9.854619843455216355 ) ) ;
#16973=PLANE ( 'NONE',  #22343 ) ;
#16974=EDGE_CURVE ( 'NONE', #21756, #32023, #35736, .T. ) ;
#16986=CARTESIAN_POINT ( 'NONE',  ( 115.5526452545247622, 0.8980012041604421569, -11.00651665394454071 ) ) ;
#16999=CARTESIAN_POINT ( 'NONE',  ( 64.53261755725110049, -37.43192534259661386, -5.214988841577086198 ) ) ;
#17000=LINE ( 'NONE', #41835, #29799 ) ;
#17005=CARTESIAN_POINT ( 'NONE',  ( 116.5249890045247980, 0.8980012041604421569, -15.77991374673208469 ) ) ;
#17009=CARTESIAN_POINT ( 'NONE',  ( 115.3442858795247759, -8.402594152722688392, -9.854619843455216355 ) ) ;
#17012=CARTESIAN_POINT ( 'NONE',  ( 108.0517077545248696, -7.250697342233347165, -7.631215200338321125 ) ) ;
#17013=CARTESIAN_POINT ( 'NONE',  ( 117.2294421295248270, -10.43749303616872837, -4.992153861205963494 ) ) ;
#17014=CARTESIAN_POINT ( 'NONE',  ( 113.8163171295247764, -10.62599879583958540, -13.39321520033831447 ) ) ;
#17033=CARTESIAN_POINT ( 'NONE',  ( 116.8819505665422724, 0.1389869644409600646, -15.19553865127072889 ) ) ;
#17034=CARTESIAN_POINT ( 'NONE',  ( 111.4549108795247747, -8.938348069036489818, -9.318865927141430916 ) ) ;
#17042=CARTESIAN_POINT ( 'NONE',  ( 109.0935046295247872, -4.863998795839590272, -18.39754474579285315 ) ) ;
#17057=CARTESIAN_POINT ( 'NONE',  ( 111.1770983795247787, -0.7896495226426338832, -9.318865927141430916 ) ) ;
#17058=CARTESIAN_POINT ( 'NONE',  ( 105.1346765045248475, -2.791137627527939813, -8.388885654883777576 ) ) ;
#17059=CARTESIAN_POINT ( 'NONE',  ( 115.2748327545248657, -2.477300249445798297, -19.15521520033831138 ) ) ;
#17062=CARTESIAN_POINT ( 'NONE',  ( 109.2294422377198515, -7.708454464063350109, -8.449852329660794581 ) ) ;
#17064=CARTESIAN_POINT ( 'NONE',  ( 107.9128015045248219, -6.936859964151250502, -18.39754474579286025 ) ) ;
#17066=CARTESIAN_POINT ( 'NONE',  ( 109.2294421296414129, -0.4681310589162339664, -15.92169685210972574 ) ) ;
#17072=CARTESIAN_POINT ( 'NONE',  ( 113.6079577545248185, -7.250697342233347165, -7.631215200338321125 ) ) ;
#17082=CARTESIAN_POINT ( 'NONE',  ( 107.6349890045248401, -9.868328341294098749, -11.32035403202665869 ) ) ;
#17091=CARTESIAN_POINT ( 'NONE',  ( 115.5526452545247622, 0.8980012041604421569, -11.00651665394454071 ) ) ;
#17094=CARTESIAN_POINT ( 'NONE',  ( 69.01908044833261613, -25.32952000468398879, -0.8932152003383146965 ) ) ;
#17095=CARTESIAN_POINT ( 'NONE',  ( 78.39334728892299609, -58.37107721070194799, -0.4530934645980765896 ) ) ;
#17099=ADVANCED_FACE ( 'NONE', ( #32002 ), #38392, .T. ) ;
#17110=CARTESIAN_POINT ( 'NONE',  ( 107.3571765045248299, -7.250697342233347165, -19.15521520033831138 ) ) ;
#17111=CARTESIAN_POINT ( 'NONE',  ( 70.19189222814998175, -84.91840466455968794, -47.17007500872661296 ) ) ;
#17112=CARTESIAN_POINT ( 'NONE',  ( 104.9263171295248327, 0.1403307496149613920, -13.39321520033831447 ) ) ;
#17115=ORIENTED_EDGE ( 'NONE', *, *, #23651, .T. ) ;
#17118=CARTESIAN_POINT ( 'NONE',  ( 76.69189222814998175, -50.16718729050181480, 3.106784799661685526 ) ) ;
#17120=CARTESIAN_POINT ( 'NONE',  ( 106.9404577545248145, -7.250697342233347165, -7.631215200338321125 ) ) ;
#17128=CARTESIAN_POINT ( 'NONE',  ( 82.53488078675573547, -31.62014037238083830, -22.36964567811433469 ) ) ;
#17135=DIRECTION ( 'NONE',  ( -1.000000000000000000, 0.000000000000000000, 0.000000000000000000 ) ) ;
#17142=VECTOR ( 'NONE', #28471, 1000.000000000000000 ) ;
#17143=CARTESIAN_POINT ( 'NONE',  ( 108.2600671295247992, -10.62599879583958540, -13.39321520033831447 ) ) ;
#17152=CARTESIAN_POINT ( 'NONE',  ( 66.06194382436763135, -14.97931106434683635, -19.39321520033831447 ) ) ;
#17153=ADVANCED_FACE ( 'NONE', ( #26529 ), #43403, .T. ) ;
#17160=ORIENTED_EDGE ( 'NONE', *, *, #40060, .T. ) ;
#17163=CARTESIAN_POINT ( 'NONE',  ( 107.3571765045248299, -7.250697342233347165, -19.15521520033831138 ) ) ;
#17164=CARTESIAN_POINT ( 'NONE',  ( 110.8298327545248299, -6.936859964151250502, -8.388885654883777576 ) ) ;
#17165=CARTESIAN_POINT ( 'NONE',  ( 108.9545983795247821, -0.7896495226426338832, -9.318865927141430916 ) ) ;
#17170=CARTESIAN_POINT ( 'NONE',  ( 112.1494421295248003, 0.8980012041604618078, -13.39321520033831447 ) ) ;
#17173=DIRECTION ( 'NONE',  ( 0.000000000000000000, 0.000000000000000000, 1.000000000000000000 ) ) ;
#17177=CARTESIAN_POINT ( 'NONE',  ( 113.9552233795247815, -1.325403438956436419, -9.854619843455211026 ) ) ;
#17179=CARTESIAN_POINT ( 'NONE',  ( 69.69189222814998175, -41.76310523276723785, -24.39321520033831447 ) ) ;
#17182=CARTESIAN_POINT ( 'NONE',  ( 107.0099108795247815, -1.325403438956436419, -16.93181055722141792 ) ) ;
#17183=CARTESIAN_POINT ( 'NONE',  ( 107.6349890045248401, -9.868328341294098749, -11.32035403202665869 ) ) ;
#17190=DIRECTION ( 'NONE',  ( -1.000000000000000000, 0.000000000000000000, 0.000000000000000000 ) ) ;
#17192=ORIENTED_EDGE ( 'NONE', *, *, #29791, .F. ) ;
#17198=VECTOR ( 'NONE', #37018, 1000.000000000000000 ) ;
#17203=CARTESIAN_POINT ( 'NONE',  ( 113.7468640045248236, -10.62599879583958717, -11.00651665394454604 ) ) ;
#17204=CARTESIAN_POINT ( 'NONE',  ( 115.1359265045248321, -2.791137627527939813, -8.388885654883754484 ) ) ;
#17209=DIRECTION ( 'NONE',  ( 0.000000000000000000, 1.000000000000000000, 0.000000000000000000 ) ) ;
#17211=EDGE_CURVE ( 'NONE', #30513, #42470, #11766, .T. ) ;
#17212=CARTESIAN_POINT ( 'NONE',  ( 111.7327388068194836, 0.1168444861213632779, -12.14321520033831625 ) ) ;
#17214=CARTESIAN_POINT ( 'NONE',  ( 65.36445175461375356, -36.61467555475167757, -5.472084168854603803 ) ) ;
#17220=DIRECTION ( 'NONE',  ( 0.000000000000000000, 0.000000000000000000, -1.000000000000000000 ) ) ;
#17221=CARTESIAN_POINT ( 'NONE',  ( 114.6497546295247929, -4.863998795839590272, -7.631215200338315796 ) ) ;
#17227=CARTESIAN_POINT ( 'NONE',  ( 108.2600671295247992, 0.1403307496149613920, -13.39321520033831447 ) ) ;
#17231=CARTESIAN_POINT ( 'NONE',  ( 107.5655358795247736, -0.7896495226426338832, -17.46756447353520159 ) ) ;
#17232=CARTESIAN_POINT ( 'NONE',  ( 109.5102233795247884, -8.938348069036489818, -17.46756447353520159 ) ) ;
#17235=CARTESIAN_POINT ( 'NONE',  ( 114.5108483795247878, -0.7896495226426338832, -9.318865927141425587 ) ) ;
#17247=EDGE_CURVE ( 'NONE', #36801, #26421, #22872, .T. ) ;
#17248=EDGE_CURVE ( 'NONE', #26462, #28048, #22200, .T. ) ;
#17251=CARTESIAN_POINT ( 'NONE',  ( 116.8251712076233417, -1.620372813598558004, -17.49680154955593991 ) ) ;
#17252=CARTESIAN_POINT ( 'NONE',  ( 112.7050671295247923, -10.62599879583958540, -13.39321520033831447 ) ) ;
#17261=CARTESIAN_POINT ( 'NONE',  ( 111.1245697905468859, 0.6938714319018670640, -12.14321520033833579 ) ) ;
#17263=CARTESIAN_POINT ( 'NONE',  ( 117.0806140045248185, 0.1403307496149616695, -15.46607636864997204 ) ) ;
#17268=CARTESIAN_POINT ( 'NONE',  ( 116.0829010812576882, -0.01829820670803256055, -12.14321520033834290 ) ) ;
#17270=VERTEX_POINT ( 'NONE', #213 ) ;
#17276=CARTESIAN_POINT ( 'NONE',  ( 109.9269421295247753, 0.8980012041604618078, -13.39321520033831447 ) ) ;
#17277=ADVANCED_FACE ( 'NONE', ( #35069 ), #3419, .F. ) ;
#17279=CARTESIAN_POINT ( 'NONE',  ( 114.2330358795247776, -0.7896495226426338832, -17.46756447353520159 ) ) ;
#17282=CARTESIAN_POINT ( 'NONE',  ( 67.69189222814998175, -59.27884951796255564, -42.87418841894956500 ) ) ;
#17285=CARTESIAN_POINT ( 'NONE',  ( 110.4825671295247815, 0.1403307496149613920, -13.39321520033831447 ) ) ;
#17286=CARTESIAN_POINT ( 'NONE',  ( 109.2294421295247844, -1.388378309844742642, -16.99368411936019641 ) ) ;
#17291=CARTESIAN_POINT ( 'NONE',  ( 113.3507721536727928, 0.3967854368540359999, -10.50530088663809636 ) ) ;
#17292=VECTOR ( 'NONE', #36928, 1000.000000000000000 ) ;
#17293=ORIENTED_EDGE ( 'NONE', *, *, #37471, .T. ) ;
#17301=EDGE_CURVE ( 'NONE', #42470, #10099, #37216, .T. ) ;
#17302=CARTESIAN_POINT ( 'NONE',  ( 108.7462390045248242, -9.868328341294098749, -11.32035403202665869 ) ) ;
#17308=DIRECTION ( 'NONE',  ( -0.3445294493088599252, -0.9387755102040817867, 0.000000000000000000 ) ) ;
#17311=CARTESIAN_POINT ( 'NONE',  ( 115.4831921295247952, 0.8980012041604618078, -13.39321520033831447 ) ) ;
#17315=FACE_OUTER_BOUND ( 'NONE', #43577, .T. ) ;
#17320=DIRECTION ( 'NONE',  ( 0.000000000000000000, -1.000000000000000000, 0.000000000000000000 ) ) ;
#17327=CARTESIAN_POINT ( 'NONE',  ( 107.2182702545248105, -10.62599879583958717, -15.77991374673208469 ) ) ;
#17329=CARTESIAN_POINT ( 'NONE',  ( 106.2459265045248173, -2.791137627527939813, -8.388885654883777576 ) ) ;
#17339=CARTESIAN_POINT ( 'NONE',  ( 110.0658483795247804, -8.402594152722688392, -16.93181055722141792 ) ) ;
#17341=EDGE_LOOP ( 'NONE', ( #10597, #33281, #10027, #28982 ) ) ;
#17353=ADVANCED_FACE ( 'NONE', ( #28043 ), #3850, .T. ) ;
#17361=CARTESIAN_POINT ( 'NONE',  ( 106.5237390045248418, 0.8980012041604421569, -15.77991374673208469 ) ) ;
#17367=DIRECTION ( 'NONE',  ( 0.000000000000000000, 0.000000000000000000, 1.000000000000000000 ) ) ;
#17379=CARTESIAN_POINT ( 'NONE',  ( 116.0845533854058829, -0.02059610140724144056, -12.14321520033831625 ) ) ;
#17380=CARTESIAN_POINT ( 'NONE',  ( 106.9404577545248145, -7.250697342233347165, -7.631215200338321125 ) ) ;
#17381=CARTESIAN_POINT ( 'NONE',  ( 109.0240515045248202, -6.936859964151250502, -18.39754474579286025 ) ) ;
#17382=CARTESIAN_POINT ( 'NONE',  ( 106.0375671295248310, -10.62599879583958540, -13.39321520033831447 ) ) ;
#17387=CARTESIAN_POINT ( 'NONE',  ( 111.3160046295247838, -4.863998795839590272, -7.631215200338315796 ) ) ;
#17392=LINE ( 'NONE', #37451, #37299 ) ;
#17394=CARTESIAN_POINT ( 'NONE',  ( 116.5944421295247793, 0.8980012041604618078, -13.39321520033831447 ) ) ;
#17395=CARTESIAN_POINT ( 'NONE',  ( 106.9404577545248145, -7.250697342233347165, -7.631215200338321125 ) ) ;
#17400=CARTESIAN_POINT ( 'NONE',  ( 115.2053796295247849, -4.863998795839590272, -19.15521520033831493 ) ) ;
#17401=CARTESIAN_POINT ( 'NONE',  ( 108.8851452545248151, -9.868328341294098749, -15.46607636864997204 ) ) ;
#17420=CARTESIAN_POINT ( 'NONE',  ( 114.4413952545248350, 0.8980012041604421569, -11.00651665394454071 ) ) ;
#17421=CARTESIAN_POINT ( 'NONE',  ( 115.2053796295247849, -4.863998795839638234, -8.388885654883775800 ) ) ;
#17426=CARTESIAN_POINT ( 'NONE',  ( 116.0388171295248014, 0.1403307496149613920, -13.39321520033831447 ) ) ;
#17429=CARTESIAN_POINT ( 'NONE',  ( 86.04230958663548279, -25.82262605124143917, -7.893215200338315363 ) ) ;
#17435=DIRECTION ( 'NONE',  ( 0.9970811988817434024, -0.07634843047859724008, 0.000000000000000000 ) ) ;
#17436=CARTESIAN_POINT ( 'NONE',  ( 111.2465515045248168, -2.477300249445798297, -7.631215200338321125 ) ) ;
#17441=CARTESIAN_POINT ( 'NONE',  ( 108.6767858795247861, -8.402594152722688392, -9.854619843455216355 ) ) ;
#17443=CARTESIAN_POINT ( 'NONE',  ( 109.2294419155992671, -4.095350944532103021, -18.49013907498823528 ) ) ;
#17445=CARTESIAN_POINT ( 'NONE',  ( 107.2182702545248105, -10.62599879583958717, -15.77991374673208469 ) ) ;
#17446=CARTESIAN_POINT ( 'NONE',  ( 108.4684265045247997, -7.250697342233347165, -19.15521520033831138 ) ) ;
#17461=CARTESIAN_POINT ( 'NONE',  ( 113.7468640045248236, -10.62599879583958717, -11.00651665394454604 ) ) ;
#17468=CIRCLE ( 'NONE', #14572, 1.999999999999999112 ) ;
#17469=DIRECTION ( 'NONE',  ( 0.9387755102040806765, -0.3445294493088623122, 0.000000000000000000 ) ) ;
#17472=FACE_OUTER_BOUND ( 'NONE', #6533, .T. ) ;
#17473=CARTESIAN_POINT ( 'NONE',  ( 115.6220983795247861, -8.402594152722688392, -16.93181055722141792 ) ) ;
#17475=( NAMED_UNIT ( * ) PLANE_ANGLE_UNIT ( ) SI_UNIT ( $, .RADIAN. ) );
#17477=CARTESIAN_POINT ( 'NONE',  ( 67.69189222814998175, -49.76310523276723785, -40.89321520033831092 ) ) ;
#17487=CARTESIAN_POINT ( 'NONE',  ( 112.8439733795247832, -8.938348069036489818, -17.46756447353520159 ) ) ;
#17490=CARTESIAN_POINT ( 'NONE',  ( 109.2294741910440052, -4.090390389109569647, -7.902357633321886787 ) ) ;
#17492=CARTESIAN_POINT ( 'NONE',  ( 109.0935046295247872, -4.863998795839590272, -18.39754474579285315 ) ) ;
#17496=CARTESIAN_POINT ( 'NONE',  ( 109.0240515045248202, -2.477300249445798297, -7.631215200338321125 ) ) ;
#17497=LINE ( 'NONE', #27327, #28657 ) ;
#17499=ORIENTED_EDGE ( 'NONE', *, *, #41809, .T. ) ;
#17509=CARTESIAN_POINT ( 'NONE',  ( 108.5378796295247810, -4.863998795839590272, -8.388885654883775800 ) ) ;
#17519=CARTESIAN_POINT ( 'NONE',  ( 114.0941296295247867, -4.863998795839590272, -19.15521520033831493 ) ) ;
#17542=CARTESIAN_POINT ( 'NONE',  ( 107.7738952545248310, 0.8980012041604421569, -11.00651665394454071 ) ) ;
#17544=CARTESIAN_POINT ( 'NONE',  ( 114.6497546295247929, -4.863998795839541422, -18.39754474579285315 ) ) ;
#17553=CARTESIAN_POINT ( 'NONE',  ( 113.2606921295247702, -9.868328341294093420, -13.39321520033831447 ) ) ;
#17561=CARTESIAN_POINT ( 'NONE',  ( 82.45341866970989031, -31.73112455768813689, -22.62568415223593377 ) ) ;
#17564=DIRECTION ( 'NONE',  ( 1.000000000000000000, 0.000000000000000000, 0.000000000000000000 ) ) ;
#17565=FACE_OUTER_BOUND ( 'NONE', #32590, .T. ) ;
#17569=AXIS2_PLACEMENT_3D ( 'NONE', #19462, #25417, #39318 ) ;
#17572=EDGE_LOOP ( 'NONE', ( #41000, #5465, #9855 ) ) ;
#17574=B_SPLINE_SURFACE_WITH_KNOTS ( 'NONE', 3, 3, ( 
 ( #3070, #41397, #6726, #37952, #20637, #9927 ),
 ( #23841, #6498, #20413, #34297, #34514, #16999 ),
 ( #3292, #30888, #17214, #13567, #44810, #31105 ),
 ( #25941, #1088, #8612, #36187, #4509, #39848 ),
 ( #21617, #25718, #18196, #7703, #25040, #32091 ),
 ( #39399, #38933, #18650, #15678, #12038, #862 ),
 ( #42598, #11811, #22511, #28915, #15002, #21841 ),
 ( #1531, #18432, #42825, #29131, #15224, #29582 ) ),
 .UNSPECIFIED., .F., .F., .F.,
 ( 4, 2, 2, 4 ),
 ( 4, 2, 4 ),
 ( 0.000000000000000000, 0.5000000000000000000, 0.7500000000000000000, 1.000000000000000000 ),
 ( 0.000000000000000000, 0.5000000000000000000, 1.000000000000000000 ),
 .UNSPECIFIED. ) ;
#17577=CARTESIAN_POINT ( 'NONE',  ( 109.0935046295247872, -4.863998795839590272, -7.631215200338315796 ) ) ;
#17584=EDGE_CURVE ( 'NONE', #40407, #3603, #37365, .T. ) ;
#17597=CARTESIAN_POINT ( 'NONE',  ( 116.0855952810452862, -0.02204510709163942650, -12.14321520033831625 ) ) ;
#17598=CARTESIAN_POINT ( 'NONE',  ( 113.7468640045248236, 0.1403307496149616695, -15.46607636864997204 ) ) ;
#17600=CARTESIAN_POINT ( 'NONE',  ( 108.9545983795247821, -8.402594152722688392, -16.93181055722141792 ) ) ;
#17601=CARTESIAN_POINT ( 'NONE',  ( 111.9410827545248708, -6.936859964151250502, -8.388885654883777576 ) ) ;
#17606=CARTESIAN_POINT ( 'NONE',  ( 110.6909265045248247, -7.250697342233347165, -19.15521520033831138 ) ) ;
#17613=CARTESIAN_POINT ( 'NONE',  ( 113.1217858795247935, -0.7896495226426338832, -17.46756447353520159 ) ) ;
#17614=CARTESIAN_POINT ( 'NONE',  ( 114.9970202545248412, 0.1403307496149616695, -11.32035403202665336 ) ) ;
#17619=CARTESIAN_POINT ( 'NONE',  ( 113.5385046295247804, -4.863998795839590272, -7.631215200338315796 ) ) ;
#17620=CARTESIAN_POINT ( 'NONE',  ( 105.0652233795248378, -1.325403438956436419, -9.854619843455211026 ) ) ;
#17624=ORIENTED_EDGE ( 'NONE', *, *, #35047, .F. ) ;
#17630=CARTESIAN_POINT ( 'NONE',  ( 109.7185827545247889, -6.936859964151250502, -8.388885654883777576 ) ) ;
#17632=ORIENTED_EDGE ( 'NONE', *, *, #30026, .T. ) ;
#17640=CARTESIAN_POINT ( 'NONE',  ( 115.0664733795247798, -8.938348069036489818, -17.46756447353520159 ) ) ;
#17655=ORIENTED_EDGE ( 'NONE', *, *, #23779, .T. ) ;
#17657=CARTESIAN_POINT ( 'NONE',  ( 109.5102388068194870, 0.1168444861213632779, -12.14321520033833757 ) ) ;
#17658=CARTESIAN_POINT ( 'NONE',  ( 112.9134265045247645, -7.250697342233347165, -19.15521520033831138 ) ) ;
#17662=CARTESIAN_POINT ( 'NONE',  ( 112.0105358795248804, -8.402594152722736354, -9.854619843455244776 ) ) ;
#17663=CARTESIAN_POINT ( 'NONE',  ( 111.0381921295247878, -9.868328341294093420, -13.39321520033831447 ) ) ;
#17666=CARTESIAN_POINT ( 'NONE',  ( 109.2294714807263887, -6.964600658336093097, -18.24697958790709151 ) ) ;
#17668=CARTESIAN_POINT ( 'NONE',  ( 108.1906140045248463, -10.62599879583958717, -11.00651665394454604 ) ) ;
#17669=CARTESIAN_POINT ( 'NONE',  ( 117.2294421295247844, -10.72535413672978599, -21.89321520033831447 ) ) ;
#17670=CARTESIAN_POINT ( 'NONE',  ( 110.5520202545248054, -10.62599879583958717, -15.77991374673208469 ) ) ;
#17676=ORIENTED_EDGE ( 'NONE', *, *, #43166, .T. ) ;
#17680=EDGE_CURVE ( 'NONE', #39064, #11127, #17497, .T. ) ;
#17682=ORIENTED_EDGE ( 'NONE', *, *, #43722, .T. ) ;
#17686=DIRECTION ( 'NONE',  ( -1.000000000000000000, 0.000000000000000000, 0.000000000000000000 ) ) ;
#17687=CARTESIAN_POINT ( 'NONE',  ( 109.5796765045248122, -7.250697342233347165, -19.15521520033831138 ) ) ;
#17688=CARTESIAN_POINT ( 'NONE',  ( 143.3676850761856940, -69.76310523276724496, -16.89321520033831447 ) ) ;
#17691=CIRCLE ( 'NONE', #43186, 0.5000000000000004441 ) ;
#17697=CARTESIAN_POINT ( 'NONE',  ( 116.3166296295247832, -4.863998795839590272, -8.388885654883775800 ) ) ;
#17699=DIRECTION ( 'NONE',  ( 0.000000000000000000, 0.000000000000000000, -1.000000000000000000 ) ) ;
#17707=CARTESIAN_POINT ( 'NONE',  ( 115.9693640045247776, 0.1403307496149616695, -15.46607636864997204 ) ) ;
#17712=CARTESIAN_POINT ( 'NONE',  ( 110.6214733795247867, -8.938348069036489818, -17.46756447353520159 ) ) ;
#17716=CARTESIAN_POINT ( 'NONE',  ( 115.4451630180080883, 0.7607806665037644134, -14.64321520033834467 ) ) ;
#17719=CARTESIAN_POINT ( 'NONE',  ( 111.1076452545248259, -9.868328341294098749, -15.46607636864997204 ) ) ;
#17720=CARTESIAN_POINT ( 'NONE',  ( 116.5060880209376535, 2.200519030075564597, -20.49989231505612963 ) ) ;
#17723=CARTESIAN_POINT ( 'NONE',  ( 112.1494421295248003, 0.8980012041604618078, -13.39321520033831447 ) ) ;
#17725=ORIENTED_EDGE ( 'NONE', *, *, #9761, .T. ) ;
#17726=UNCERTAINTY_MEASURE_WITH_UNIT (LENGTH_MEASURE( 1.000000000000000082E-05 ), #21341, 'distance_accuracy_value', 'NONE');
#17734=CARTESIAN_POINT ( 'NONE',  ( 107.0099108795247815, -1.325403438956436419, -16.93181055722141792 ) ) ;
#17744=CARTESIAN_POINT ( 'NONE',  ( 114.9970202545248412, -10.62599879583958717, -15.77991374673208469 ) ) ;
#17752=VECTOR ( 'NONE', #39568, 1000.000000000000000 ) ;
#17759=ORIENTED_EDGE ( 'NONE', *, *, #30102, .F. ) ;
#17761=CARTESIAN_POINT ( 'NONE',  ( 115.7610046295247912, -4.863998795839590272, -18.39754474579285315 ) ) ;
#17767=VERTEX_POINT ( 'NONE', #24350 ) ;
#17776=CARTESIAN_POINT ( 'NONE',  ( 111.8021765045248372, -2.791137627527939813, -8.388885654883777576 ) ) ;
#17778=ORIENTED_EDGE ( 'NONE', *, *, #28630, .F. ) ;
#17787=CARTESIAN_POINT ( 'NONE',  ( 110.2065776191212763, 0.4261359969231631739, -12.14321520033831625 ) ) ;
#17789=ORIENTED_EDGE ( 'NONE', *, *, #17796, .F. ) ;
#17796=EDGE_CURVE ( 'NONE', #24941, #34537, #20928, .T. ) ;
#17799=CARTESIAN_POINT ( 'NONE',  ( 105.7597546295248350, -4.863998795839590272, -7.631215200338315796 ) ) ;
#17804=LINE ( 'NONE', #38759, #41609 ) ;
#17818=CARTESIAN_POINT ( 'NONE',  ( 114.7886608795247696, -1.325403438956436419, -16.93181055722141792 ) ) ;
#17819=CARTESIAN_POINT ( 'NONE',  ( 108.4684265045247997, -2.791137627527939813, -8.388885654883777576 ) ) ;
#17820=CARTESIAN_POINT ( 'NONE',  ( 111.8021765045248372, -2.791137627527939813, -8.388885654883777576 ) ) ;
#17825=CARTESIAN_POINT ( 'NONE',  ( 110.8298327545248299, -2.477300249445798297, -19.15521520033831138 ) ) ;
#17831=EDGE_CURVE ( 'NONE', #40625, #29947, #45100, .T. ) ;
#17832=CARTESIAN_POINT ( 'NONE',  ( 116.3166296295247832, -4.863998795839590272, -19.15521520033831493 ) ) ;
#17833=CARTESIAN_POINT ( 'NONE',  ( 105.8986608795248401, -8.938348069036489818, -9.318865927141430916 ) ) ;
#17835=ORIENTED_EDGE ( 'NONE', *, *, #25861, .F. ) ;
#17836=DIRECTION ( 'NONE',  ( -1.000000000000000000, 0.000000000000000000, 0.000000000000000000 ) ) ;
#17839=CARTESIAN_POINT ( 'NONE',  ( 116.0388171295248014, -10.62599879583958540, -13.39321520033831447 ) ) ;
#17840=CARTESIAN_POINT ( 'NONE',  ( 109.0240515045248202, -6.936859964151250502, -18.39754474579286025 ) ) ;
#17853=CARTESIAN_POINT ( 'NONE',  ( 112.1494421295248003, -9.868328341294093420, -13.39321520033831447 ) ) ;
#17863=CYLINDRICAL_SURFACE ( 'NONE', #42688, 2.000000000000000444 ) ;
#17865=CARTESIAN_POINT ( 'NONE',  ( 110.2047546295247855, -4.863998795839590272, -7.631215200338315796 ) ) ;
#17866=CARTESIAN_POINT ( 'NONE',  ( 117.1162029564635674, -11.29425726270896035, -21.74748621749282051 ) ) ;
#17870=ORIENTED_EDGE ( 'NONE', *, *, #23468, .T. ) ;
#17871=AXIS2_PLACEMENT_3D ( 'NONE', #29449, #31963, #18294 ) ;
#17875=CARTESIAN_POINT ( 'NONE',  ( 115.2053796295247849, -4.863998795839590272, -19.15521520033831493 ) ) ;
#17879=LINE ( 'NONE', #34734, #45109 ) ;
#17880=CARTESIAN_POINT ( 'NONE',  ( 110.6909265045248247, -7.250697342233347165, -19.15521520033831138 ) ) ;
#17885=CARTESIAN_POINT ( 'NONE',  ( 111.1770983795247787, -8.402594152722688392, -16.93181055722141792 ) ) ;
#17886=VERTEX_POINT ( 'NONE', #13031 ) ;
#17888=CARTESIAN_POINT ( 'NONE',  ( 109.2294337548798779, -7.896060072502915084, -17.78522704774125174 ) ) ;
#17892=CARTESIAN_POINT ( 'NONE',  ( 115.1359265045248605, -2.791137627527939813, -8.388885654883777576 ) ) ;
#17893=CARTESIAN_POINT ( 'NONE',  ( 107.8433483795247838, -0.7896495226426338832, -9.318865927141430916 ) ) ;
#17900=VERTEX_POINT ( 'NONE', #27161 ) ;
#17902=CARTESIAN_POINT ( 'NONE',  ( 84.86020291624612355, -30.49489077589588604, -18.39321520033831803 ) ) ;
#17905=ORIENTED_EDGE ( 'NONE', *, *, #39993, .F. ) ;
#17908=EDGE_CURVE ( 'NONE', #34165, #30525, #981, .T. ) ;
#17910=CARTESIAN_POINT ( 'NONE',  ( 109.9269421295247753, 0.8980012041604618078, -13.39321520033831447 ) ) ;
#17920=CARTESIAN_POINT ( 'NONE',  ( 115.3442858795247759, -8.402594152722688392, -9.854619843455216355 ) ) ;
#17932=CARTESIAN_POINT ( 'NONE',  ( 113.3995983795247895, -8.402594152722688392, -16.93181055722141792 ) ) ;
#17936=CARTESIAN_POINT ( 'NONE',  ( 84.89885432604606308, -29.90127023760751612, -11.39376025726712349 ) ) ;
#17937=CARTESIAN_POINT ( 'NONE',  ( 112.7050671295247923, -10.62599879583958540, -13.39321520033831447 ) ) ;
#17940=CARTESIAN_POINT ( 'NONE',  ( 116.5987716749792895, -9.866677412677834269, -13.52174868289714027 ) ) ;
#17941=CARTESIAN_POINT ( 'NONE',  ( 109.2295693424392908, -6.082835033032921501, -7.893315249734571104 ) ) ;
#17943=CARTESIAN_POINT ( 'NONE',  ( 110.9687390045248350, -9.868328341294098749, -11.32035403202665869 ) ) ;
#17944=CARTESIAN_POINT ( 'NONE',  ( 116.5324863327809339, 2.186940848879305399, -20.53455829175617353 ) ) ;
#17947=CARTESIAN_POINT ( 'NONE',  ( 109.9269421295247753, 0.8980012041604618078, -13.39321520033831447 ) ) ;
#17957=CARTESIAN_POINT ( 'NONE',  ( 113.4690515045247992, -2.477300249445798297, -7.631215200338321125 ) ) ;
#17967=CARTESIAN_POINT ( 'NONE',  ( 106.1764733795248219, -1.325403438956436419, -9.854619843455211026 ) ) ;
#17971=CARTESIAN_POINT ( 'NONE',  ( 77.38585178070579218, -56.64430055435828848, -1.796958453011376022 ) ) ;
#17981=CARTESIAN_POINT ( 'NONE',  ( 84.86020291624612355, -29.99489077589588959, -12.39321520033834645 ) ) ;
#17983=ORIENTED_EDGE ( 'NONE', *, *, #26672, .T. ) ;
#17985=CARTESIAN_POINT ( 'NONE',  ( 112.0799890045248475, -9.868328341294098749, -11.32035403202665869 ) ) ;
#17998=CARTESIAN_POINT ( 'NONE',  ( 113.9552233795247815, -1.325403438956436419, -9.854619843455211026 ) ) ;
#18011=CARTESIAN_POINT ( 'NONE',  ( 115.4137390045248566, -9.868328341294098749, -11.32035403202665869 ) ) ;
#18022=LINE ( 'NONE', #1362, #16114 ) ;
#18028=DIRECTION ( 'NONE',  ( 1.000000000000000000, 0.000000000000000000, 0.000000000000000000 ) ) ;
#18038=ORIENTED_EDGE ( 'NONE', *, *, #32620, .T. ) ;
#18040=CARTESIAN_POINT ( 'NONE',  ( 116.3166296295247832, -4.863998795839590272, -19.15521520033831493 ) ) ;
#18041=CARTESIAN_POINT ( 'NONE',  ( 112.3578015045248861, -6.936859964151250502, -18.39754474579286025 ) ) ;
#18042=CARTESIAN_POINT ( 'NONE',  ( 111.1076452545248259, -9.868328341294098749, -15.46607636864997204 ) ) ;
#18043=CARTESIAN_POINT ( 'NONE',  ( 112.4272546295247821, -4.863998795839590272, -18.39754474579285315 ) ) ;
#18050=CARTESIAN_POINT ( 'NONE',  ( 107.6349890045248401, 0.8980012041604421569, -15.77991374673208469 ) ) ;
#18056=CARTESIAN_POINT ( 'NONE',  ( 79.05243529145373316, 4.793396140045460108, -5.736853407927685389 ) ) ;
#18058=CARTESIAN_POINT ( 'NONE',  ( 115.6220983795247861, -0.7896495226426338832, -9.318865927141430916 ) ) ;
#18059=CARTESIAN_POINT ( 'NONE',  ( 111.3160046295247838, -4.863998795839590272, -18.39754474579285315 ) ) ;
#18068=ORIENTED_EDGE ( 'NONE', *, *, #33209, .T. ) ;
#18074=CARTESIAN_POINT ( 'NONE',  ( 106.7320983795247855, -0.7896495226426338832, -9.318865927141430916 ) ) ;
#18075=CARTESIAN_POINT ( 'NONE',  ( 111.1076452545248259, -9.868328341294098749, -15.46607636864997204 ) ) ;
#18077=EDGE_CURVE ( 'NONE', #32023, #12824, #18867, .T. ) ;
#18083=EDGE_CURVE ( 'NONE', #30411, #12824, #27641, .T. ) ;
#18088=EDGE_CURVE ( 'NONE', #26016, #35384, #16768, .T. ) ;
#18089=CARTESIAN_POINT ( 'NONE',  ( 110.4825671295247815, -10.62599879583958540, -13.39321520033831447 ) ) ;
#18095=CARTESIAN_POINT ( 'NONE',  ( 115.1359265045248605, -7.250697342233347165, -19.15521520033831138 ) ) ;
#18103=CARTESIAN_POINT ( 'NONE',  ( 110.9687390045248350, 0.8980012041604421569, -15.77991374673208469 ) ) ;
#18110=CARTESIAN_POINT ( 'NONE',  ( 109.9269421295247753, -9.868328341294093420, -13.39321520033831447 ) ) ;
#18113=CARTESIAN_POINT ( 'NONE',  ( 109.2294421295618321, -7.227482384100928137, -18.13879607630843793 ) ) ;
#18116=CARTESIAN_POINT ( 'NONE',  ( 116.3166296295247832, -4.863998795839590272, -8.388885654883775800 ) ) ;
#18117=CARTESIAN_POINT ( 'NONE',  ( 106.1070202545248407, -10.62599879583958717, -15.77991374673208469 ) ) ;
#18125=LINE ( 'NONE', #14706, #40005 ) ;
#18127=( BOUNDED_CURVE ( )  B_SPLINE_CURVE ( 2, ( #41408, #14243, #24724, #41179, #3304, #10164, #3741, #31118, #20865, #30900, #6281, #3524, #27937, #45042, #24294, #41628, #34085 ),
 .UNSPECIFIED., .F., .F. ) 
 B_SPLINE_CURVE_WITH_KNOTS ( ( 3, 2, 2, 2, 2, 2, 2, 2, 3 ),
 ( 0.4035091206787220219, 0.4124999999999999778, 0.4249999999999999889, 0.4375000000000000000, 0.4500000000000000111, 0.4625000000000000222, 0.4749999999999999778, 0.4874999999999999889, 0.4964908793212780003 ),
 .UNSPECIFIED. ) 
 CURVE ( )  GEOMETRIC_REPRESENTATION_ITEM ( )  RATIONAL_B_SPLINE_CURVE ( ( 0.9692594319298230010, 0.9452488050343769155, 1.000000000000000000, 0.9238795325112869605, 1.000000000000000000, 0.9238795325112869605, 1.000000000000000000, 0.9238795325112869605, 1.000000000000000000, 0.9238795325112869605, 1.000000000000000000, 0.9238795325112869605, 1.000000000000000000, 0.9238795325112869605, 1.000000000000000000, 0.9452488050343769155, 0.9692594319298220018 ) ) 
 REPRESENTATION_ITEM ( '' )  );
#18129=ORIENTED_EDGE ( 'NONE', *, *, #20701, .F. ) ;
#18133=CARTESIAN_POINT ( 'NONE',  ( 108.6073327545248048, -2.477300249445798297, -19.15521520033831138 ) ) ;
#18134=CYLINDRICAL_SURFACE ( 'NONE', #26422, 20.00000000000000000 ) ;
#18136=CARTESIAN_POINT ( 'NONE',  ( 115.3442858795247759, -8.402594152722688392, -9.854619843455216355 ) ) ;
#18145=CARTESIAN_POINT ( 'NONE',  ( 113.2606921295247702, -9.868328341294093420, -13.39321520033831447 ) ) ;
#18153=ORIENTED_EDGE ( 'NONE', *, *, #3058, .T. ) ;
#18154=LINE ( 'NONE', #31829, #39163 ) ;
#18156=CARTESIAN_POINT ( 'NONE',  ( 116.1082702545247827, 0.1403307496149616695, -11.32035403202665336 ) ) ;
#18159=CARTESIAN_POINT ( 'NONE',  ( 86.21301144467663846, -26.71832258603155807, -8.459175720980109503 ) ) ;
#18160=CARTESIAN_POINT ( 'NONE',  ( 112.7745202545247878, -10.62599879583958717, -15.77991374673208469 ) ) ;
#18164=CARTESIAN_POINT ( 'NONE',  ( 109.2294819584304548, -4.447028745678551331, -7.844385157708282819 ) ) ;
#18166=CARTESIAN_POINT ( 'NONE',  ( 115.4831921295247952, 0.8980012041604618078, -13.39321520033831447 ) ) ;
#18167=DIRECTION ( 'NONE',  ( 0.000000000000000000, 0.000000000000000000, -1.000000000000000000 ) ) ;
#18170=CARTESIAN_POINT ( 'NONE',  ( 113.0523327545247838, -2.477300249445798297, -19.15521520033831138 ) ) ;
#18171=EDGE_CURVE ( 'NONE', #17900, #40637, #29171, .T. ) ;
#18182=CARTESIAN_POINT ( 'NONE',  ( 112.0799890045248475, 0.8980012041604421569, -15.77991374673208469 ) ) ;
#18185=CARTESIAN_POINT ( 'NONE',  ( 63.69189222814998175, -50.16718729050181480, -4.893215200338314474 ) ) ;
#18196=CARTESIAN_POINT ( 'NONE',  ( 64.70066334234053329, -35.74738352678537012, -5.786960771376285173 ) ) ;
#18198=CARTESIAN_POINT ( 'NONE',  ( 115.9294421295247872, -10.76310523276723785, -4.893215200338314474 ) ) ;
#18210=CARTESIAN_POINT ( 'NONE',  ( 111.7327233795247849, -1.325403438956436419, -9.854619843455211026 ) ) ;
#18212=CARTESIAN_POINT ( 'NONE',  ( 114.7192077545248452, -2.791137627527887410, -18.39754474579284249 ) ) ;
#18215=DIRECTION ( 'NONE',  ( 0.000000000000000000, 0.000000000000000000, -1.000000000000000000 ) ) ;
#18218=AXIS2_PLACEMENT_3D ( 'NONE', #21452, #35335, #18028 ) ;
#18225=CARTESIAN_POINT ( 'NONE',  ( 109.9269421295247753, -9.868328341294093420, -13.39321520033831447 ) ) ;
#18234=LINE ( 'NONE', #14365, #20129 ) ;
#18237=ORIENTED_EDGE ( 'NONE', *, *, #15015, .T. ) ;
#18242=CARTESIAN_POINT ( 'NONE',  ( 70.19189222814998175, -66.90480655070588512, -34.57954022122791571 ) ) ;
#18256=CARTESIAN_POINT ( 'NONE',  ( 77.77634386988368931, 3.254514819260763581, -7.393215200338315363 ) ) ;
#18268=CARTESIAN_POINT ( 'NONE',  ( 115.2053796295247849, -4.863998795839590272, -19.15521520033831493 ) ) ;
#18269=CARTESIAN_POINT ( 'NONE',  ( 113.6774108795247997, -1.325403438956436419, -16.93181055722141792 ) ) ;
#18270=CARTESIAN_POINT ( 'NONE',  ( 111.6632702545248605, 0.1403307496149616695, -11.32035403202665336 ) ) ;
#18275=CARTESIAN_POINT ( 'NONE',  ( 105.7597546295248350, -4.863998795839590272, -7.631215200338315796 ) ) ;
#18278=CARTESIAN_POINT ( 'NONE',  ( 109.2294520814496650, -0.4000957807073393102, -15.81271325186753351 ) ) ;
#18279=CARTESIAN_POINT ( 'NONE',  ( 79.38366267499158369, 5.039764807350117337, -6.277090637128386774 ) ) ;
#18281=CARTESIAN_POINT ( 'NONE',  ( 112.7050671295247923, -10.62599879583958540, -13.39321520033831447 ) ) ;
#18282=CARTESIAN_POINT ( 'NONE',  ( 109.5796765045248122, -2.791137627527939813, -8.388885654883777576 ) ) ;
#18294=DIRECTION ( 'NONE',  ( 0.000000000000000000, 0.000000000000000000, -1.000000000000000000 ) ) ;
#18296=ORIENTED_EDGE ( 'NONE', *, *, #43714, .T. ) ;
#18299=CARTESIAN_POINT ( 'NONE',  ( 106.7320983795247855, -8.402594152722688392, -16.93181055722141792 ) ) ;
#18307=FACE_OUTER_BOUND ( 'NONE', #40274, .T. ) ;
#18313=CARTESIAN_POINT ( 'NONE',  ( 109.9269421295247753, 0.8980012041604618078, -13.39321520033831447 ) ) ;
#18318=B_SPLINE_CURVE_WITH_KNOTS ( 'NONE', 3,
 ( #8224, #15740, #15510, #8669, #4341, #43104, #25335, #29417, #12100, #5014, #5241, #22353, #1148, #21901, #22130, #1813, #26004, #22572, #28979, #39460, #7993, #36023, #41831, #14844, #32381, #15065, #18932, #39908, #36474, #39228, #4567, #4791, #925, #35795, #10591, #32819, #19157, #18491, #33038, #24493, #18712, #42884, #39003 ),
 .UNSPECIFIED., .F., .F.,
 ( 4, 2, 2, 2, 1, 1, 1, 2, 2, 2, 2, 2, 2, 2, 2, 2, 2, 2, 2, 2, 2, 2, 4 ),
 ( 0.000000000000000000, 0.1250000000000104361, 0.1875000000000154321, 0.2187500000000180134, 0.2343750000000193456, 0.2421875000000199563, 0.2460937500000199285, 0.2480468750000195954, 0.2500000000000192624, 0.3750000000000177636, 0.4375000000000173195, 0.4687500000000175970, 0.4843750000000168754, 0.4921875000000162093, 0.4960937500000164313, 0.5000000000000166533, 0.6250000000000119904, 0.6875000000000097700, 0.7187500000000087708, 0.7343750000000083267, 0.7500000000000078826, 0.8750000000000039968, 1.000000000000000000 ),
 .UNSPECIFIED. ) ;
#18323=CARTESIAN_POINT ( 'NONE',  ( 116.0286950891469786, 2.331313199634366118, -12.14321520033831625 ) ) ;
#18330=CARTESIAN_POINT ( 'NONE',  ( 110.6214733795247867, -8.938348069036489818, -17.46756447353520159 ) ) ;
#18339=CARTESIAN_POINT ( 'NONE',  ( 109.2295187470875817, -2.680572428980009914, -17.98422477323183344 ) ) ;
#18344=CARTESIAN_POINT ( 'NONE',  ( 114.0941296295247867, -4.863998795839590272, -8.388885654883775800 ) ) ;
#18358=ORIENTED_EDGE ( 'NONE', *, *, #43166, .F. ) ;
#18360=ADVANCED_FACE ( 'NONE', ( #39535 ), #14463, .T. ) ;
#18363=CARTESIAN_POINT ( 'NONE',  ( 108.6767858795247861, -0.7896495226426338832, -17.46756447353520159 ) ) ;
#18367=DIRECTION ( 'NONE',  ( -0.9659258262890688673, -0.2588190451025190186, 0.000000000000000000 ) ) ;
#18369=CARTESIAN_POINT ( 'NONE',  ( 113.6774108795247997, -1.325403438956436419, -16.93181055722141792 ) ) ;
#18377=CARTESIAN_POINT ( 'NONE',  ( 109.2324108795247923, -1.325403438956436419, -16.93181055722141792 ) ) ;
#18386=ORIENTED_EDGE ( 'NONE', *, *, #22951, .T. ) ;
#18389=CARTESIAN_POINT ( 'NONE',  ( 113.2606921295247702, -9.868328341294093420, -13.39321520033831447 ) ) ;
#18392=CARTESIAN_POINT ( 'NONE',  ( 84.86020291624612355, -29.99489077589590025, -11.89662724278569073 ) ) ;
#18393=CARTESIAN_POINT ( 'NONE',  ( 108.1906140045248463, -10.62599879583958717, -11.00651665394454604 ) ) ;
#18397=CARTESIAN_POINT ( 'NONE',  ( 109.2294535371698174, -0.3920599432768472337, -10.47762860381350336 ) ) ;
#18399=CARTESIAN_POINT ( 'NONE',  ( 115.8999108795247821, -8.938348069036489818, -9.318865927141430916 ) ) ;
#18401=CARTESIAN_POINT ( 'NONE',  ( 86.04230958663552542, -25.82262605124138943, -7.893215200338315363 ) ) ;
#18402=CARTESIAN_POINT ( 'NONE',  ( 82.50011035870637954, -31.66751168766318614, -23.35869902906633655 ) ) ;
#18405=CARTESIAN_POINT ( 'NONE',  ( 110.8298327545248299, -2.477300249445798297, -19.15521520033831138 ) ) ;
#18415=CARTESIAN_POINT ( 'NONE',  ( 111.5938171295247940, -10.62599879583958540, -13.39321520033831447 ) ) ;
#18416=VECTOR ( 'NONE', #32030, 1000.000000000000227 ) ;
#18417=B_SPLINE_CURVE_WITH_KNOTS ( 'NONE', 3,
 ( #35584, #10546, #35125, #38337 ),
 .UNSPECIFIED., .F., .F.,
 ( 4, 4 ),
 ( 0.000000000000000000, 1.000000000000000000 ),
 .UNSPECIFIED. ) ;
#18425=ORIENTED_EDGE ( 'NONE', *, *, #41490, .T. ) ;
#18432=CARTESIAN_POINT ( 'NONE',  ( 64.01282776924008999, -34.86145050234441811, -5.893215200338315363 ) ) ;
#18447=CARTESIAN_POINT ( 'NONE',  ( 114.4413952545248350, -9.868328341294098749, -15.46607636864997204 ) ) ;
#18453=VERTEX_POINT ( 'NONE', #9198 ) ;
#18458=CARTESIAN_POINT ( 'NONE',  ( 109.7880358795247986, -8.402594152722688392, -9.854619843455216355 ) ) ;
#18459=ORIENTED_EDGE ( 'NONE', *, *, #6734, .F. ) ;
#18471=CARTESIAN_POINT ( 'NONE',  ( 115.6220983795247861, -8.402594152722688392, -16.93181055722141792 ) ) ;
#18472=AXIS2_PLACEMENT_3D ( 'NONE', #24235, #34688, #3476 ) ;
#18483=ADVANCED_FACE ( 'NONE', ( #39976 ), #2339, .F. ) ;
#18484=CARTESIAN_POINT ( 'NONE',  ( 79.43841117369071014, 5.060937148469339064, -20.42529936998274209 ) ) ;
#18491=CARTESIAN_POINT ( 'NONE',  ( 116.7165501589519749, -6.821145072361184170, -18.12697020542095672 ) ) ;
#18498=CARTESIAN_POINT ( 'NONE',  ( 115.7610046295247912, -4.863998795839590272, -18.39754474579285315 ) ) ;
#18499=CARTESIAN_POINT ( 'NONE',  ( 114.7886608795247696, -1.325403438956436419, -16.93181055722141792 ) ) ;
#18504=CARTESIAN_POINT ( 'NONE',  ( 108.1211608795247798, -8.938348069036489818, -9.318865927141430916 ) ) ;
#18508=DIRECTION ( 'NONE',  ( 0.000000000000000000, 0.000000000000000000, 1.000000000000000000 ) ) ;
#18510=CARTESIAN_POINT ( 'NONE',  ( 110.4825671295247815, -10.62599879583958540, -13.39321520033831447 ) ) ;
#18511=CARTESIAN_POINT ( 'NONE',  ( 111.0381921295247878, -9.868328341294093420, -13.39321520033831447 ) ) ;
#18520=ORIENTED_EDGE ( 'NONE', *, *, #27569, .T. ) ;
#18528=CARTESIAN_POINT ( 'NONE',  ( 114.7886608795247696, -8.938348069036489818, -9.318865927141430916 ) ) ;
#18530=ORIENTED_EDGE ( 'NONE', *, *, #31267, .F. ) ;
#18537=ORIENTED_EDGE ( 'NONE', *, *, #28384, .T. ) ;
#18539=CARTESIAN_POINT ( 'NONE',  ( 61.80837279822206654, -65.83902806826597498, -43.67070380127381668 ) ) ;
#18540=CARTESIAN_POINT ( 'NONE',  ( 111.0381921295247878, 0.8980012041604618078, -13.39321520033831447 ) ) ;
#18544=DIRECTION ( 'NONE',  ( 0.000000000000000000, -0.6161630946014903243, -0.7876185884367603585 ) ) ;
#18549=CARTESIAN_POINT ( 'NONE',  ( 117.0111608795247946, -1.325403438956436419, -16.93181055722141792 ) ) ;
#18550=CARTESIAN_POINT ( 'NONE',  ( 114.6497546295247929, -4.863998795839590272, -7.631215200338315796 ) ) ;
#18552=ORIENTED_EDGE ( 'NONE', *, *, #6433, .F. ) ;
#18555=CARTESIAN_POINT ( 'NONE',  ( 107.3571765045248299, -7.250697342233347165, -19.15521520033831138 ) ) ;
#18560=CARTESIAN_POINT ( 'NONE',  ( 79.05243529145373316, 4.793396140045460108, -4.893215200338314474 ) ) ;
#18561=CARTESIAN_POINT ( 'NONE',  ( 107.2182702545248105, 0.1403307496149616695, -11.32035403202665336 ) ) ;
#18563=CARTESIAN_POINT ( 'NONE',  ( 115.9693640045247776, -10.62599879583958540, -11.00651665394454604 ) ) ;
#18564=CARTESIAN_POINT ( 'NONE',  ( 109.2294435684327141, -10.04426263482621273, -15.20456221528482388 ) ) ;
#18566=CARTESIAN_POINT ( 'NONE',  ( 113.1912390045248031, -9.868328341294098749, -11.32035403202665869 ) ) ;
#18567=CARTESIAN_POINT ( 'NONE',  ( 107.2877233795247776, -8.938348069036489818, -17.46756447353520159 ) ) ;
#18570=DIRECTION ( 'NONE',  ( 0.000000000000000000, -1.000000000000000000, 0.000000000000000000 ) ) ;
#18573=ORIENTED_EDGE ( 'NONE', *, *, #3448, .T. ) ;
#18580=( BOUNDED_CURVE ( )  B_SPLINE_CURVE ( 3, ( #9463, #9016, #2382, #40249 ),
 .UNSPECIFIED., .F., .F. ) 
 B_SPLINE_CURVE_WITH_KNOTS ( ( 4, 4 ),
 ( 3.141592653589795336, 4.712388980384689674 ),
 .UNSPECIFIED. ) 
 CURVE ( )  GEOMETRIC_REPRESENTATION_ITEM ( )  RATIONAL_B_SPLINE_CURVE ( ( 1.000000000000000000, 0.8047378541243649375, 0.8047378541243649375, 1.000000000000000000 ) ) 
 REPRESENTATION_ITEM ( '' )  );
#18583=CARTESIAN_POINT ( 'NONE',  ( 110.5520202545248054, -10.62599879583958717, -15.77991374673208469 ) ) ;
#18588=CARTESIAN_POINT ( 'NONE',  ( 112.2188952545247531, -9.868328341294098749, -15.46607636864997204 ) ) ;
#18594=CARTESIAN_POINT ( 'NONE',  ( 110.0658483795247804, -8.402594152722688392, -16.93181055722141792 ) ) ;
#18606=CARTESIAN_POINT ( 'NONE',  ( 112.3578015045248861, -6.936859964151250502, -18.39754474579286025 ) ) ;
#18610=CARTESIAN_POINT ( 'NONE',  ( 86.21326076097346913, -26.71771895156159715, -8.459066486029300336 ) ) ;
#18611=CARTESIAN_POINT ( 'NONE',  ( 108.7462390045248242, 0.8980012041604421569, -15.77991374673208469 ) ) ;
#18618=CARTESIAN_POINT ( 'NONE',  ( 114.6497546295247929, -4.863998795839590272, -7.631215200338315796 ) ) ;
#18620=DIRECTION ( 'NONE',  ( 0.000000000000000000, 0.000000000000000000, 1.000000000000000000 ) ) ;
#18624=CARTESIAN_POINT ( 'NONE',  ( 108.0517077545248696, -7.250697342233347165, -7.631215200338321125 ) ) ;
#18628=DIRECTION ( 'NONE',  ( 0.3445294493088594256, 0.9387755102040817867, 0.000000000000000000 ) ) ;
#18630=CARTESIAN_POINT ( 'NONE',  ( 116.3198046295247963, -4.863998795839590272, -8.393215200338314474 ) ) ;
#18636=CARTESIAN_POINT ( 'NONE',  ( 115.6915515045247531, -2.477300249445798297, -7.631215200338321125 ) ) ;
#18645=CARTESIAN_POINT ( 'NONE',  ( 60.19189222814998175, -66.20485342690169261, -45.06987807991851724 ) ) ;
#18650=CARTESIAN_POINT ( 'NONE',  ( 64.35867204304231848, -35.30545456751979572, -5.871741255084275579 ) ) ;
#18655=EDGE_CURVE ( 'NONE', #27212, #32081, #17392, .T. ) ;
#18666=CARTESIAN_POINT ( 'NONE',  ( 112.8439733795247832, -1.325403438956436419, -9.854619843455211026 ) ) ;
#18667=CARTESIAN_POINT ( 'NONE',  ( 82.59722093989569203, -31.76965857943681826, -23.00835853622210436 ) ) ;
#18670=AXIS2_PLACEMENT_3D ( 'NONE', #44543, #13755, #27884 ) ;
#18678=CARTESIAN_POINT ( 'NONE',  ( 106.2459265045248173, -2.791137627527939813, -8.388885654883777576 ) ) ;
#18690=VERTEX_POINT ( 'NONE', #7117 ) ;
#18691=VECTOR ( 'NONE', #16870, 1000.000000000000000 ) ;
#18692=CARTESIAN_POINT ( 'NONE',  ( 117.1500671295247713, 0.1403307496149613920, -13.39321520033831447 ) ) ;
#18695=EDGE_LOOP ( 'NONE', ( #26979, #19101, #44226, #22335, #9535 ) ) ;
#18704=DIRECTION ( 'NONE',  ( 0.000000000000000000, -1.000000000000000000, -6.938893903907222067E-15 ) ) ;
#18712=CARTESIAN_POINT ( 'NONE',  ( 116.7470998475920254, -5.364568849815520402, -18.53181687022155799 ) ) ;
#18717=STYLED_ITEM('',(#45162),#6587);
#18719=CARTESIAN_POINT ( 'NONE',  ( 115.8999108795247821, -8.938348069036489818, -9.318865927141430916 ) ) ;
#18720=CARTESIAN_POINT ( 'NONE',  ( 109.8574890045248509, -9.868328341294098749, -11.32035403202665869 ) ) ;
#18721=CARTESIAN_POINT ( 'NONE',  ( 110.8992858795247827, -8.402594152722688392, -9.854619843455216355 ) ) ;
#18724=ORIENTED_EDGE ( 'NONE', *, *, #30687, .F. ) ;
#18726=CARTESIAN_POINT ( 'NONE',  ( 108.9545983795247821, -0.7896495226426338832, -9.318865927141430916 ) ) ;
#18729=CYLINDRICAL_SURFACE ( 'NONE', #11682, 2.000000000000003109 ) ;
#18732=CARTESIAN_POINT ( 'NONE',  ( 109.8574890045247940, 0.8980012041604421569, -15.77991374673208469 ) ) ;
#18733=CARTESIAN_POINT ( 'NONE',  ( 109.7880358795247986, -8.402594152722688392, -9.854619843455216355 ) ) ;
#18744=ORIENTED_EDGE ( 'NONE', *, *, #7475, .F. ) ;
#18752=CARTESIAN_POINT ( 'NONE',  ( 107.2182702545248105, 0.1403307496149616695, -11.32035403202665336 ) ) ;
#18762=CARTESIAN_POINT ( 'NONE',  ( 61.78267613169789740, -65.90120773829286804, -43.52498728833642616 ) ) ;
#18763=CARTESIAN_POINT ( 'NONE',  ( 112.9828796295247884, -4.863998795839590272, -19.15521520033831493 ) ) ;
#18764=AXIS2_PLACEMENT_3D ( 'NONE', #24264, #3273, #44566 ) ;
#18770=ORIENTED_EDGE ( 'NONE', *, *, #12948, .F. ) ;
#18773=CARTESIAN_POINT ( 'NONE',  ( 111.6632702545248605, -10.62599879583958717, -15.77991374673208469 ) ) ;
#18774=CARTESIAN_POINT ( 'NONE',  ( 116.5944421295247793, -9.868328341294093420, -13.39321520033831447 ) ) ;
#18775=CARTESIAN_POINT ( 'NONE',  ( 116.2471765045247594, -7.250697342233347165, -19.15521520033831138 ) ) ;
#18780=CARTESIAN_POINT ( 'NONE',  ( 107.9128015045248219, -2.477300249445798297, -7.631215200338321125 ) ) ;
#18788=CARTESIAN_POINT ( 'NONE',  ( 109.2294421295247844, -8.865838614420134434, -9.247624522711900497 ) ) ;
#18790=EDGE_CURVE ( 'NONE', #24351, #21469, #32287, .T. ) ;
#18791=CARTESIAN_POINT ( 'NONE',  ( 112.3578015045248861, -6.936859964151250502, -18.39754474579286025 ) ) ;
#18792=CARTESIAN_POINT ( 'NONE',  ( 106.8710046295248759, -4.863998795839590272, -7.631215200338315796 ) ) ;
#18797=EDGE_LOOP ( 'NONE', ( #7336, #34147, #8471, #10744 ) ) ;
#18802=EDGE_LOOP ( 'NONE', ( #39861, #1746, #14260, #36054 ) ) ;
#18803=LINE ( 'NONE', #16748, #38348 ) ;
#18808=CARTESIAN_POINT ( 'NONE',  ( 114.7192077545248594, -2.791137627527939813, -18.39754474579286025 ) ) ;
#18815=CARTESIAN_POINT ( 'NONE',  ( 111.9410827545248708, -6.936859964151250502, -8.388885654883777576 ) ) ;
#18822=EDGE_LOOP ( 'NONE', ( #18296, #11494 ) ) ;
#18825=CARTESIAN_POINT ( 'NONE',  ( 108.1906140045248037, 0.1403307496149616695, -15.46607636864997204 ) ) ;
#18830=CARTESIAN_POINT ( 'NONE',  ( 109.5102233795247884, -8.938348069036489818, -17.46756447353520159 ) ) ;
#18836=CARTESIAN_POINT ( 'NONE',  ( 106.5931921295248372, -9.868328341294093420, -13.39321520033831447 ) ) ;
#18838=CARTESIAN_POINT ( 'NONE',  ( 82.71771818927497577, -31.37104225293308701, -22.09381113811972597 ) ) ;
#18846=CARTESIAN_POINT ( 'NONE',  ( 112.6609831777918913, -0.01829820670813664396, -14.64321520033831447 ) ) ;
#18852=CARTESIAN_POINT ( 'NONE',  ( 115.2053796295247849, -4.863998795839590272, -19.15521520033831493 ) ) ;
#18855=CARTESIAN_POINT ( 'NONE',  ( 110.4825671295247815, -10.62599879583958540, -13.39321520033834290 ) ) ;
#18857=ORIENTED_EDGE ( 'NONE', *, *, #40402, .T. ) ;
#18860=VERTEX_POINT ( 'NONE', #39247 ) ;
#18867=B_SPLINE_CURVE_WITH_KNOTS ( 'NONE', 3,
 ( #44583, #23608, #17212, #32162, #931, #31934, #30886, #700, #14620, #27251 ),
 .UNSPECIFIED., .F., .F.,
 ( 4, 3, 3, 4 ),
 ( 0.000000000000000000, 0.0002476487219222849707, 0.0004952974148303769834, 0.0009534114850261750764 ),
 .UNSPECIFIED. ) ;
#18869=ADVANCED_FACE ( 'NONE', ( #4809, #21475 ), #32398, .F. ) ;
#18877=CARTESIAN_POINT ( 'NONE',  ( 115.0664733795247798, -1.325403438956436419, -9.854619843455211026 ) ) ;
#18881=CARTESIAN_POINT ( 'NONE',  ( 116.4555358795247884, -0.7896495226426338832, -17.46756447353520159 ) ) ;
#18882=CARTESIAN_POINT ( 'NONE',  ( 107.0099108795247815, -1.325403438956436419, -16.93181055722141792 ) ) ;
#18883=CARTESIAN_POINT ( 'NONE',  ( 63.69189222814998175, -40.21211973637273474, -4.893215200338314474 ) ) ;
#18894=CARTESIAN_POINT ( 'NONE',  ( 105.6903015045248253, -6.936859964151250502, -18.39754474579286025 ) ) ;
#18901=DIRECTION ( 'NONE',  ( 0.9970811988817434024, -0.07634843047859753151, 0.000000000000000000 ) ) ;
#18909=ORIENTED_EDGE ( 'NONE', *, *, #20009, .F. ) ;
#18913=CARTESIAN_POINT ( 'NONE',  ( 110.8298327545248299, -6.936859964151250502, -8.388885654883788234 ) ) ;
#18915=VERTEX_POINT ( 'NONE', #32623 ) ;
#18917=AXIS2_PLACEMENT_3D ( 'NONE', #7101, #13732, #34673 ) ;
#18919=CARTESIAN_POINT ( 'NONE',  ( 110.2047546295247855, -4.863998795839541422, -18.39754474579285315 ) ) ;
#18932=CARTESIAN_POINT ( 'NONE',  ( 116.6779416893911616, -8.401490633876564473, -17.04399421721747743 ) ) ;
#18937=CARTESIAN_POINT ( 'NONE',  ( 114.6998541094426969, 0.3591747506842615789, -12.14321520033831625 ) ) ;
#18938=CARTESIAN_POINT ( 'NONE',  ( 114.3719421295247827, 0.8980012041604618078, -13.39321520033831447 ) ) ;
#18939=CARTESIAN_POINT ( 'NONE',  ( 110.8992858795247827, -8.402594152722688392, -9.854619843455216355 ) ) ;
#18940=CARTESIAN_POINT ( 'NONE',  ( 110.3436608795247764, -1.325403438956436419, -16.93181055722141792 ) ) ;
#18944=CARTESIAN_POINT ( 'NONE',  ( 106.6626452545248611, 0.8980012041604421569, -11.00651665394454071 ) ) ;
#18947=CARTESIAN_POINT ( 'NONE',  ( 109.2295909607760933, -0.1191545588266860467, -15.28045812891908284 ) ) ;
#18950=CARTESIAN_POINT ( 'NONE',  ( 110.7603796295247918, -4.863998795839590272, -19.15521520033831493 ) ) ;
#18958=CYLINDRICAL_SURFACE ( 'NONE', #29294, 2.000000000000000000 ) ;
#18970=CARTESIAN_POINT ( 'NONE',  ( 108.2600671295247992, 0.1403307496149613920, -13.39321520033831447 ) ) ;
#18972=EDGE_CURVE ( 'NONE', #11934, #16272, #40025, .T. ) ;
#18979=CARTESIAN_POINT ( 'NONE',  ( 62.68840920241336789, -64.78138427943380862, -45.84136708138180438 ) ) ;
#18980=CARTESIAN_POINT ( 'NONE',  ( 107.7738952545248310, 0.8980012041604421569, -11.00651665394454071 ) ) ;
#18981=AXIS2_PLACEMENT_3D ( 'NONE', #36084, #28143, #21742 ) ;
#18988=ORIENTED_EDGE ( 'NONE', *, *, #22220, .T. ) ;
#18991=CARTESIAN_POINT ( 'NONE',  ( 111.2465515045248168, -2.477300249445798297, -7.631215200338321125 ) ) ;
#18992=CARTESIAN_POINT ( 'NONE',  ( 115.8304577545247582, -2.791137627527939813, -18.39754474579286025 ) ) ;
#18993=CARTESIAN_POINT ( 'NONE',  ( 110.4131140045248287, -10.62599879583958717, -11.00651665394454604 ) ) ;
#18999=CARTESIAN_POINT ( 'NONE',  ( 106.5237390045248418, 0.8980012041604421569, -15.77991374673208469 ) ) ;
#19003=CARTESIAN_POINT ( 'NONE',  ( 116.6195842771102917, -11.86478987849519662, -6.418176294668409554 ) ) ;
#19005=DIRECTION ( 'NONE',  ( 0.000000000000000000, 0.000000000000000000, -1.000000000000000000 ) ) ;
#19006=CARTESIAN_POINT ( 'NONE',  ( 109.2296195588419749, -9.603284990525381204, -16.08186249415100733 ) ) ;
#19008=CARTESIAN_POINT ( 'NONE',  ( 112.2188952545247531, -9.868328341294098749, -15.46607636864997204 ) ) ;
#19009=CARTESIAN_POINT ( 'NONE',  ( 115.5526452545247622, -9.868328341294098749, -15.46607636864997204 ) ) ;
#19012=CARTESIAN_POINT ( 'NONE',  ( 71.36090047007586179, -25.24828423334623650, -5.221195830130035631 ) ) ;
#19028=CARTESIAN_POINT ( 'NONE',  ( 105.7597546295248350, -4.863998795839590272, -7.631215200338315796 ) ) ;
#19031=CARTESIAN_POINT ( 'NONE',  ( 114.0941296295247867, -4.863998795839590272, -8.388885654883775800 ) ) ;
#19033=FACE_OUTER_BOUND ( 'NONE', #20795, .T. ) ;
#19034=DIRECTION ( 'NONE',  ( 0.6383198453882299450, 0.7697712484781087383, -9.200178928217186715E-17 ) ) ;
#19040=CARTESIAN_POINT ( 'NONE',  ( 109.5102233795247884, -1.325403438956436419, -9.854619843455211026 ) ) ;
#19043=DIRECTION ( 'NONE',  ( -1.000000000000000000, 0.000000000000000000, 0.000000000000000000 ) ) ;
#19049=EDGE_LOOP ( 'NONE', ( #24151, #40916, #27833, #3461, #12789 ) ) ;
#19050=CARTESIAN_POINT ( 'NONE',  ( 114.8834831777918879, -0.01829820670803256055, -14.64321520033831447 ) ) ;
#19052=CARTESIAN_POINT ( 'NONE',  ( 107.8433483795247838, -8.402594152722688392, -16.93181055722141792 ) ) ;
#19057=CARTESIAN_POINT ( 'NONE',  ( 106.7320983795247855, -0.7896495226426338832, -9.318865927141430916 ) ) ;
#19063=CARTESIAN_POINT ( 'NONE',  ( 112.7050671295247923, -10.62599879583958540, -13.39321520033831447 ) ) ;
#19065=CARTESIAN_POINT ( 'NONE',  ( 82.45341866970989031, -31.73112455768813689, -22.62568415223593377 ) ) ;
#19068=CARTESIAN_POINT ( 'NONE',  ( 106.5237390045248418, 0.8980012041604421569, -15.77991374673208469 ) ) ;
#19071=ORIENTED_EDGE ( 'NONE', *, *, #28346, .T. ) ;
#19072=CARTESIAN_POINT ( 'NONE',  ( 112.6135934012278881, 0.04929351793716424401, -14.64321520033828961 ) ) ;
#19079=CARTESIAN_POINT ( 'NONE',  ( 110.3436608795247764, -8.938348069036489818, -9.318865927141430916 ) ) ;
#19080=CIRCLE ( 'NONE', #8864, 20.00000000000000000 ) ;
#19082=DIRECTION ( 'NONE',  ( 1.000000000000000000, 0.000000000000000000, 0.000000000000000000 ) ) ;
#19083=CARTESIAN_POINT ( 'NONE',  ( 116.0388171295248014, -10.62599879583958540, -13.39321520033831447 ) ) ;
#19089=CARTESIAN_POINT ( 'NONE',  ( 115.0664888068194927, 0.1168444861213632779, -12.14321520033831625 ) ) ;
#19095=DIRECTION ( 'NONE',  ( 0.000000000000000000, 0.9284778069183720062, 0.3713878862591650232 ) ) ;
#19101=ORIENTED_EDGE ( 'NONE', *, *, #13618, .F. ) ;
#19104=FACE_OUTER_BOUND ( 'NONE', #2501, .T. ) ;
#19109=VECTOR ( 'NONE', #25753, 1000.000000000000000 ) ;
#19111=CARTESIAN_POINT ( 'NONE',  ( 114.9970202545248412, -10.62599879583958717, -15.77991374673208469 ) ) ;
#19112=CARTESIAN_POINT ( 'NONE',  ( 109.3713171295247832, 0.1403307496149613920, -13.39321520033831447 ) ) ;
#19116=CARTESIAN_POINT ( 'NONE',  ( 64.69189222814998175, -41.76310523276723785, -4.893215200338314474 ) ) ;
#19117=CARTESIAN_POINT ( 'NONE',  ( 116.1082702545247827, 0.1403307496149616695, -11.32035403202665336 ) ) ;
#19124=CARTESIAN_POINT ( 'NONE',  ( 109.5102233795247884, -1.325403438956436419, -9.854619843455211026 ) ) ;
#19125=ORIENTED_EDGE ( 'NONE', *, *, #19698, .T. ) ;
#19131=CARTESIAN_POINT ( 'NONE',  ( 79.63740429864273551, 3.112009832785464614, -19.89321520033831447 ) ) ;
#19132=CYLINDRICAL_SURFACE ( 'NONE', #12846, 20.00000000000000355 ) ;
#19135=CARTESIAN_POINT ( 'NONE',  ( 113.3995983795247895, -8.402594152722688392, -16.93181055722141792 ) ) ;
#19145=DIRECTION ( 'NONE',  ( -1.000000000000000000, 0.000000000000000000, 0.000000000000000000 ) ) ;
#19148=LINE ( 'NONE', #33031, #14937 ) ;
#19157=CARTESIAN_POINT ( 'NONE',  ( 116.7153894074022418, -6.872978516340015886, -18.10395076569972517 ) ) ;
#19166=CARTESIAN_POINT ( 'NONE',  ( 112.4967077545247633, -7.250697342233347165, -7.631215200338321125 ) ) ;
#19167=CARTESIAN_POINT ( 'NONE',  ( 111.1770983795247787, -8.402594152722688392, -16.93181055722141792 ) ) ;
#19168=CARTESIAN_POINT ( 'NONE',  ( 109.1629577545248395, -2.791137627527939813, -18.39754474579286025 ) ) ;
#19171=ORIENTED_EDGE ( 'NONE', *, *, #25857, .F. ) ;
#19173=FACE_OUTER_BOUND ( 'NONE', #36530, .T. ) ;
#19179=CARTESIAN_POINT ( 'NONE',  ( 110.0658483795247804, -0.7896495226426338832, -9.318865927141430916 ) ) ;
#19193=EDGE_CURVE ( 'NONE', #22775, #22330, #33754, .T. ) ;
#19201=CARTESIAN_POINT ( 'NONE',  ( 108.3295202545248657, 0.1403307496149616695, -11.32035403202665336 ) ) ;
#19207=CARTESIAN_POINT ( 'NONE',  ( 78.69189222814998175, -69.76310523276724496, -0.9932152003383157846 ) ) ;
#19211=CARTESIAN_POINT ( 'NONE',  ( 61.70909112414298647, -66.14783507974324550, -42.93797631241571366 ) ) ;
#19212=CARTESIAN_POINT ( 'NONE',  ( 107.0793640045248196, -10.62599879583958717, -11.00651665394454604 ) ) ;
#19218=ORIENTED_EDGE ( 'NONE', *, *, #35001, .F. ) ;
#19221=CARTESIAN_POINT ( 'NONE',  ( 77.12856116249137983, -44.30583187727815186, -4.893215200338314474 ) ) ;
#19222=CARTESIAN_POINT ( 'NONE',  ( 111.0381921295247878, 0.8980012041604618078, -13.39321520033831447 ) ) ;
#19225=CARTESIAN_POINT ( 'NONE',  ( 110.0658483795247804, -0.7896495226426338832, -9.318865927141430916 ) ) ;
#19229=CARTESIAN_POINT ( 'NONE',  ( 62.74672096151675760, -37.51679531015581404, -5.130621874892657530 ) ) ;
#19230=CARTESIAN_POINT ( 'NONE',  ( 106.4542858795248179, -0.7896495226426338832, -17.46756447353520159 ) ) ;
#19236=DIRECTION ( 'NONE',  ( 0.7697712484781088493, -0.6383198453882299450, 0.000000000000000000 ) ) ;
#19237=CARTESIAN_POINT ( 'NONE',  ( 109.2292917470664833, -9.019994622780936666, -16.84346519180415669 ) ) ;
#19239=CARTESIAN_POINT ( 'NONE',  ( 111.6632702545248605, 0.1403307496149616695, -11.32035403202665336 ) ) ;
#19240=CARTESIAN_POINT ( 'NONE',  ( 109.7880358795247986, -8.402594152722688392, -9.854619843455216355 ) ) ;
#19243=CARTESIAN_POINT ( 'NONE',  ( 70.55229225240181279, -24.89194276641628889, -5.467054258871676176 ) ) ;
#19247=ADVANCED_FACE ( 'NONE', ( #43815 ), #18958, .F. ) ;
#19255=EDGE_LOOP ( 'NONE', ( #6819, #35614, #14591, #30381 ) ) ;
#19261=CARTESIAN_POINT ( 'NONE',  ( 107.8433483795247838, -0.7896495226426338832, -9.318865927141430916 ) ) ;
#19265=CARTESIAN_POINT ( 'NONE',  ( 111.5938171295247940, 0.1403307496149613920, -13.39321520033831447 ) ) ;
#19266=CARTESIAN_POINT ( 'NONE',  ( 79.72353890764954087, 4.236894767232761261, -4.893215200338314474 ) ) ;
#19272=CARTESIAN_POINT ( 'NONE',  ( 116.5976171295247923, -9.863998795839538758, -13.39321520033831447 ) ) ;
#19273=CARTESIAN_POINT ( 'NONE',  ( 107.9128015045248219, -6.936859964151250502, -18.39754474579286025 ) ) ;
#19282=ORIENTED_EDGE ( 'NONE', *, *, #30927, .T. ) ;
#19283=CARTESIAN_POINT ( 'NONE',  ( 110.2010952706806819, 0.3193521225029610777, -14.64321520033831447 ) ) ;
#19285=CARTESIAN_POINT ( 'NONE',  ( 112.0105358795247810, -8.402594152722688392, -9.854619843455216355 ) ) ;
#19290=CARTESIAN_POINT ( 'NONE',  ( 109.6491296295247793, -4.863998795839590272, -19.15521520033831493 ) ) ;
#19294=CARTESIAN_POINT ( 'NONE',  ( 110.9687390045248350, 0.8980012041604421569, -15.77991374673208469 ) ) ;
#19296=CARTESIAN_POINT ( 'NONE',  ( 116.4555358795247884, -0.7896495226426338832, -17.46756447353520159 ) ) ;
#19299=CARTESIAN_POINT ( 'NONE',  ( 107.1488171295247867, -10.62599879583958540, -13.39321520033831447 ) ) ;
#19312=CARTESIAN_POINT ( 'NONE',  ( 109.6491296295247793, -4.863998795839590272, -19.15521520033831493 ) ) ;
#19319=CARTESIAN_POINT ( 'NONE',  ( 115.0190408578216932, 0.04929351793716424401, -12.14321520033833934 ) ) ;
#19324=CARTESIAN_POINT ( 'NONE',  ( 109.7439176093651980, 0.5600166689815611054, -14.64321520033831447 ) ) ;
#19334=CARTESIAN_POINT ( 'NONE',  ( 115.7610046295247912, -4.863998795839590272, -18.39754474579285315 ) ) ;
#19336=VECTOR ( 'NONE', #24277, 1000.000000000000000 ) ;
#19339=CARTESIAN_POINT ( 'NONE',  ( 113.6079577545248043, -7.250697342233347165, -7.631215200338321125 ) ) ;
#19340=CARTESIAN_POINT ( 'NONE',  ( 108.5378796295247810, -4.863998795839590272, -8.388885654883775800 ) ) ;
#19343=DIRECTION ( 'NONE',  ( 0.000000000000000000, 0.000000000000000000, -1.000000000000000000 ) ) ;
#19344=CARTESIAN_POINT ( 'NONE',  ( 114.9275671295247889, 0.1403307496149613920, -13.39321520033831447 ) ) ;
#19351=CARTESIAN_POINT ( 'NONE',  ( 107.9128015045248219, -6.936859964151250502, -18.39754474579286025 ) ) ;
#19361=CARTESIAN_POINT ( 'NONE',  ( 111.6632702545248605, 0.1403307496149616695, -11.32035403202665336 ) ) ;
#19366=CARTESIAN_POINT ( 'NONE',  ( 143.3676850761856940, -68.13214146720427777, -20.74076566292611545 ) ) ;
#19370=DIRECTION ( 'NONE',  ( 0.000000000000000000, 2.168404344971010101E-16, -1.000000000000000000 ) ) ;
#19387=CARTESIAN_POINT ( 'NONE',  ( 111.5938171295247940, -10.62599879583958540, -13.39321520033831447 ) ) ;
#19388=CARTESIAN_POINT ( 'NONE',  ( 110.9687390045248350, -9.868328341294098749, -11.32035403202665869 ) ) ;
#19389=CARTESIAN_POINT ( 'NONE',  ( 108.1906140045248463, 0.1403307496149616695, -15.46607636864997204 ) ) ;
#19394=CARTESIAN_POINT ( 'NONE',  ( 61.69189222814998175, -50.16718729050181480, 3.106784799661685526 ) ) ;
#19400=CARTESIAN_POINT ( 'NONE',  ( 108.3295202545248657, -10.62599879583958717, -15.77991374673208469 ) ) ;
#19401=CARTESIAN_POINT ( 'NONE',  ( 69.69189222814998175, -41.76310523276723785, -24.39321520033831447 ) ) ;
#19419=CARTESIAN_POINT ( 'NONE',  ( 113.3301452545248083, 0.8980012041604421569, -11.00651665394454071 ) ) ;
#19428=FACE_OUTER_BOUND ( 'NONE', #10083, .T. ) ;
#19439=ORIENTED_EDGE ( 'NONE', *, *, #10852, .F. ) ;
#19442=CARTESIAN_POINT ( 'NONE',  ( 112.0799890045248475, 0.8980012041604421569, -15.77991374673208469 ) ) ;
#19443=CARTESIAN_POINT ( 'NONE',  ( 114.8581140045248361, 0.1403307496149616695, -15.46607636864997204 ) ) ;
#19444=CARTESIAN_POINT ( 'NONE',  ( 113.1912390045248031, 0.8980012041604421569, -15.77991374673208469 ) ) ;
#19448=CARTESIAN_POINT ( 'NONE',  ( 63.69189222814998175, -37.86175736943883408, -4.893215200338314474 ) ) ;
#19449=CARTESIAN_POINT ( 'NONE',  ( 109.0935046295247872, -4.863998795839590272, -7.631215200338315796 ) ) ;
#19453=CARTESIAN_POINT ( 'NONE',  ( 116.6292570341474288, -11.85868526616381047, -6.404461157504905522 ) ) ;
#19455=EDGE_LOOP ( 'NONE', ( #31130, #39502, #37840, #5549 ) ) ;
#19457=CARTESIAN_POINT ( 'NONE',  ( 109.2294548792482516, -10.43681072401148135, -13.08540494253950470 ) ) ;
#19459=CARTESIAN_POINT ( 'NONE',  ( 114.0246765045248196, -2.791137627527939813, -8.388885654883777576 ) ) ;
#19460=CARTESIAN_POINT ( 'NONE',  ( 112.8439733795247832, -1.325403438956436419, -9.854619843455211026 ) ) ;
#19462=CARTESIAN_POINT ( 'NONE',  ( 117.2294421295247844, 1.035107641088057973, -4.893215200338314474 ) ) ;
#19463=CARTESIAN_POINT ( 'NONE',  ( 70.09983049117633414, -25.86019782604198980, -5.724353937072335086 ) ) ;
#19466=ORIENTED_EDGE ( 'NONE', *, *, #5958, .T. ) ;
#19468=EDGE_CURVE ( 'NONE', #4906, #22775, #16292, .T. ) ;
#19474=DIRECTION ( 'NONE',  ( -3.317300593186674996E-33, 1.195183497228115774E-16, -1.000000000000000000 ) ) ;
#19481=CARTESIAN_POINT ( 'NONE',  ( 108.1906140045248463, -10.62599879583958717, -11.00651665394454604 ) ) ;
#19482=LINE ( 'NONE', #15611, #13346 ) ;
#19484=CARTESIAN_POINT ( 'NONE',  ( 108.3989733795247759, -1.325403438956436419, -9.854619843455211026 ) ) ;
#19494=CARTESIAN_POINT ( 'NONE',  ( 116.8722546295247895, -4.863998795839590272, -18.39754474579285315 ) ) ;
#19497=CARTESIAN_POINT ( 'NONE',  ( 116.5944421295247793, -4.863998795839590272, -18.39321520033831803 ) ) ;
#19500=CARTESIAN_POINT ( 'NONE',  ( 114.3216384760652744, 0.6362173239733635022, -12.14321520033831625 ) ) ;
#19504=CARTESIAN_POINT ( 'NONE',  ( 109.8889130180080826, 0.7607806665037644134, -14.64321520033833579 ) ) ;
#19506=CARTESIAN_POINT ( 'NONE',  ( 112.2188952545247531, -9.868328341294098749, -15.46607636864997204 ) ) ;
#19511=CARTESIAN_POINT ( 'NONE',  ( 113.6774108795247997, -1.325403438956436419, -16.93181055722141792 ) ) ;
#19512=CARTESIAN_POINT ( 'NONE',  ( 78.69189222814998175, -48.76310523276723785, -24.89321520033831447 ) ) ;
#19516=CARTESIAN_POINT ( 'NONE',  ( 111.8021765045248372, -7.250697342233347165, -19.15521520033831138 ) ) ;
#19517=CARTESIAN_POINT ( 'NONE',  ( 116.2175407567830518, 2.316852922634951017, -20.12813529906391352 ) ) ;
#19518=CARTESIAN_POINT ( 'NONE',  ( 114.5803015045248117, -2.477300249445798297, -7.631215200338321125 ) ) ;
#19521=CARTESIAN_POINT ( 'NONE',  ( 106.8015515045248378, -2.477300249445798297, -7.631215200338321125 ) ) ;
#19525=CARTESIAN_POINT ( 'NONE',  ( 109.2914656780534841, 0.1539732345883643161, -12.14321520033831625 ) ) ;
#19534=CARTESIAN_POINT ( 'NONE',  ( 108.8851452545248151, 0.8980012041604421569, -11.00651665394454071 ) ) ;
#19536=CARTESIAN_POINT ( 'NONE',  ( 110.6909265045248247, -7.250697342233347165, -19.15521520033832203 ) ) ;
#19538=ORIENTED_EDGE ( 'NONE', *, *, #42605, .F. ) ;
#19545=CARTESIAN_POINT ( 'NONE',  ( 92.26512299712632625, -23.76310523276723785, -6.893215200338315363 ) ) ;
#19547=CARTESIAN_POINT ( 'NONE',  ( 61.76986277844709861, -39.32091226840162079, -4.893215200338314474 ) ) ;
#19557=CARTESIAN_POINT ( 'NONE',  ( 114.3024890045248156, -9.868328341294098749, -11.32035403202665869 ) ) ;
#19561=CARTESIAN_POINT ( 'NONE',  ( 113.7468640045248236, -10.62599879583958717, -11.00651665394454604 ) ) ;
#19562=CARTESIAN_POINT ( 'NONE',  ( 108.1906140045248463, 0.1403307496149616695, -15.46607636864997204 ) ) ;
#19563=CARTESIAN_POINT ( 'NONE',  ( 82.83387690911449397, -31.80118368680629715, -23.16660311822836960 ) ) ;
#19567=CARTESIAN_POINT ( 'NONE',  ( 113.2606921295247702, -9.868328341294093420, -13.39321520033831447 ) ) ;
#19574=CARTESIAN_POINT ( 'NONE',  ( 116.4165695033805292, -11.97005334918662101, -21.03157055382677854 ) ) ;
#19575=VERTEX_POINT ( 'NONE', #27831 ) ;
#19579=SURFACE_SIDE_STYLE ('',( #23921 ) ) ;
#19581=CARTESIAN_POINT ( 'NONE',  ( 71.90980237029992850, -25.93883227901748967, -4.893215200338314474 ) ) ;
#19583=CARTESIAN_POINT ( 'NONE',  ( 113.6079577545248043, -2.791137627527939813, -18.39754474579286025 ) ) ;
#19595=DIRECTION ( 'NONE',  ( -1.000000000000000000, 0.000000000000000000, 0.000000000000000000 ) ) ;
#19599=CARTESIAN_POINT ( 'NONE',  ( 70.36267391504958368, -5.685877709920885259, -4.893215200338314474 ) ) ;
#19609=EDGE_LOOP ( 'NONE', ( #235, #31951, #40012, #28671 ) ) ;
#19611=CARTESIAN_POINT ( 'NONE',  ( 111.0381921295247878, 0.8980012041604618078, -13.39321520033831447 ) ) ;
#19612=CARTESIAN_POINT ( 'NONE',  ( 109.6491296295247793, -4.863998795839590272, -8.388885654883775800 ) ) ;
#19613=CARTESIAN_POINT ( 'NONE',  ( 110.1353015045248469, -6.936859964151250502, -18.39754474579286025 ) ) ;
#19614=CARTESIAN_POINT ( 'NONE',  ( 64.29809874639587974, -36.27217697897505388, -5.693345502272438630 ) ) ;
#19619=CARTESIAN_POINT ( 'NONE',  ( 117.2294421295247417, -10.73794132348372266, -21.89321520033831092 ) ) ;
#19621=CARTESIAN_POINT ( 'NONE',  ( 106.6626452545248611, -9.868328341294098749, -15.46607636864997204 ) ) ;
#19623=CARTESIAN_POINT ( 'NONE',  ( 115.1359265045248605, -2.791137627527939813, -8.388885654883777576 ) ) ;
#19635=EDGE_LOOP ( 'NONE', ( #33747, #8966, #26140, #11191, #37633, #5385, #27514, #43292, #18386, #7372, #43262, #25615, #41759, #9769 ) ) ;
#19642=CARTESIAN_POINT ( 'NONE',  ( 113.6774108795247997, -8.938348069036489818, -9.318865927141430916 ) ) ;
#19649=AXIS2_PLACEMENT_3D ( 'NONE', #35849, #18544, #1645 ) ;
#19663=CARTESIAN_POINT ( 'NONE',  ( 113.8857702545248003, -10.62599879583958717, -15.77991374673208469 ) ) ;
#19664=CARTESIAN_POINT ( 'NONE',  ( 112.0105358795247810, -8.402594152722688392, -9.854619843455216355 ) ) ;
#19665=CARTESIAN_POINT ( 'NONE',  ( 111.8021765045248372, -7.250697342233347165, -19.15521520033831138 ) ) ;
#19680=AXIS2_PLACEMENT_3D ( 'NONE', #41682, #44657, #10443 ) ;
#19683=CARTESIAN_POINT ( 'NONE',  ( 116.1082702545247827, -10.62599879583958717, -15.77991374673208469 ) ) ;
#19684=CARTESIAN_POINT ( 'NONE',  ( 112.0105358795248804, -8.402594152722688392, -9.854619843455216355 ) ) ;
#19687=CARTESIAN_POINT ( 'NONE',  ( 80.19189222814998175, -75.31442247550837976, -37.94335727672635272 ) ) ;
#19688=CARTESIAN_POINT ( 'NONE',  ( 68.96255064148981262, -26.01231434226903616, -5.893215200338315363 ) ) ;
#19691=ORIENTED_EDGE ( 'NONE', *, *, #15010, .F. ) ;
#19698=EDGE_CURVE ( 'NONE', #20261, #8479, #39522, .T. ) ;
#19700=VECTOR ( 'NONE', #41013, 1000.000000000000114 ) ;
#19703=CARTESIAN_POINT ( 'NONE',  ( 106.1764733795248219, -8.938348069036489818, -17.46756447353520159 ) ) ;
#19707=CARTESIAN_POINT ( 'NONE',  ( 110.3436608795247764, -1.325403438956436419, -16.93181055722141792 ) ) ;
#19709=DIRECTION ( 'NONE',  ( -0.6383198453882299450, -0.7697712484781087383, 0.000000000000000000 ) ) ;
#19720=DIRECTION ( 'NONE',  ( 0.000000000000000000, 0.000000000000000000, -1.000000000000000000 ) ) ;
#19727=CARTESIAN_POINT ( 'NONE',  ( 109.7880358795247986, -8.402594152722688392, -9.854619843455216355 ) ) ;
#19733=CARTESIAN_POINT ( 'NONE',  ( 105.6903015045248253, -2.477300249445798297, -7.631215200338321125 ) ) ;
#19738=CARTESIAN_POINT ( 'NONE',  ( 109.4407702545248355, -10.62599879583958717, -15.77991374673208469 ) ) ;
#19739=CARTESIAN_POINT ( 'NONE',  ( 116.0286950891469786, 2.331313199634366118, -19.89321520033831447 ) ) ;
#19740=CARTESIAN_POINT ( 'NONE',  ( 113.6079577545248043, -7.250697342233347165, -7.631215200338321125 ) ) ;
#19743=CARTESIAN_POINT ( 'NONE',  ( 114.4620221536727485, 0.3967854368540359999, -10.50530088663808925 ) ) ;
#19761=CARTESIAN_POINT ( 'NONE',  ( 107.7738952545248310, 0.8980012041604421569, -11.00651665394454071 ) ) ;
#19773=CARTESIAN_POINT ( 'NONE',  ( 108.9545983795247821, -8.402594152722688392, -16.93181055722141792 ) ) ;
#19774=DIRECTION ( 'NONE',  ( -0.1736481776669309696, -0.9848077530122079093, 0.000000000000000000 ) ) ;
#19776=CIRCLE ( 'NONE', #33587, 4.500000000000003553 ) ;
#19784=CARTESIAN_POINT ( 'NONE',  ( 116.1082702545247827, 0.1403307496149616695, -11.32035403202665336 ) ) ;
#19788=CARTESIAN_POINT ( 'NONE',  ( 114.6497546295247929, -4.863998795839590272, -7.631215200338315796 ) ) ;
#19790=CARTESIAN_POINT ( 'NONE',  ( 108.7462390045248242, -9.868328341294098749, -11.32035403202665869 ) ) ;
#19795=CARTESIAN_POINT ( 'NONE',  ( 115.6220983795247861, -8.402594152722688392, -16.93181055722141792 ) ) ;
#19796=ORIENTED_EDGE ( 'NONE', *, *, #25029, .T. ) ;
#19813=CARTESIAN_POINT ( 'NONE',  ( 110.0658483795247804, -8.402594152722688392, -16.93181055722141792 ) ) ;
#19825=FACE_OUTER_BOUND ( 'NONE', #33298, .T. ) ;
#19844=CARTESIAN_POINT ( 'NONE',  ( 113.1217858795247935, -0.7896495226426338832, -17.46756447353520159 ) ) ;
#19846=VECTOR ( 'NONE', #16404, 1000.000000000000114 ) ;
#19852=CARTESIAN_POINT ( 'NONE',  ( 87.44708369096657918, -21.99489077589588604, -18.39321520033831803 ) ) ;
#19854=CARTESIAN_POINT ( 'NONE',  ( 104.9263171295248327, 0.1403307496149613920, -13.39321520033831447 ) ) ;
#19857=CARTESIAN_POINT ( 'NONE',  ( 114.6497546295247929, -4.863998795839590272, -18.39754474579285315 ) ) ;
#19860=DIRECTION ( 'NONE',  ( 0.000000000000000000, 0.000000000000000000, 1.000000000000000000 ) ) ;
#19871=ADVANCED_FACE ( 'NONE', ( #23232 ), #8646, .T. ) ;
#19877=STYLED_ITEM ( 'NONE', ( #2924 ), #41161 ) ;
#19878=CARTESIAN_POINT ( 'NONE',  ( 114.3024890045248156, 0.8980012041604421569, -15.77991374673208469 ) ) ;
#19881=VECTOR ( 'NONE', #2367, 1000.000000000000000 ) ;
#19886=ORIENTED_EDGE ( 'NONE', *, *, #30026, .F. ) ;
#19888=CARTESIAN_POINT ( 'NONE',  ( 108.6767858795247861, -0.7896495226426338832, -17.46756447353520159 ) ) ;
#19899=CARTESIAN_POINT ( 'NONE',  ( 108.1211608795247798, -8.938348069036489818, -9.318865927141430916 ) ) ;
#19901=CARTESIAN_POINT ( 'NONE',  ( 111.2465515045248168, -6.936859964151250502, -18.39754474579286025 ) ) ;
#19902=CARTESIAN_POINT ( 'NONE',  ( 112.7050671295247923, -10.62599879583958540, -13.39321520033831447 ) ) ;
#19919=CARTESIAN_POINT ( 'NONE',  ( 108.6767858795247861, -8.402594152722688392, -9.854619843455216355 ) ) ;
#19920=CARTESIAN_POINT ( 'NONE',  ( 110.6214733795247867, -1.325403438956436419, -9.854619843455211026 ) ) ;
#19922=CARTESIAN_POINT ( 'NONE',  ( 70.64808409340794526, -25.00190304748438663, -5.469311635450234910 ) ) ;
#19929=ADVANCED_FACE ( 'NONE', ( #2018 ), #33461, .F. ) ;
#19937=CARTESIAN_POINT ( 'NONE',  ( 108.4684265045247997, -7.250697342233347165, -19.15521520033831138 ) ) ;
#19941=CARTESIAN_POINT ( 'NONE',  ( 110.1353015045248469, -6.936859964151250502, -18.39754474579286025 ) ) ;
#19942=CIRCLE ( 'NONE', #25766, 4.500000000000003553 ) ;
#19943=CARTESIAN_POINT ( 'NONE',  ( 115.4137390045248566, -9.868328341294150263, -11.32035403202669777 ) ) ;
#19948=DIRECTION ( 'NONE',  ( 0.000000000000000000, 0.000000000000000000, -1.000000000000000000 ) ) ;
#19953=CARTESIAN_POINT ( 'NONE',  ( 114.0027383310706881, 0.1843591316377651834, -12.14321520033831625 ) ) ;
#19958=FACE_OUTER_BOUND ( 'NONE', #24521, .T. ) ;
#19959=CARTESIAN_POINT ( 'NONE',  ( 116.2471765045247594, -7.250697342233347165, -19.15521520033831138 ) ) ;
#19964=CARTESIAN_POINT ( 'NONE',  ( 115.4137390045248566, -9.868328341294098749, -11.32035403202665869 ) ) ;
#19968=CARTESIAN_POINT ( 'NONE',  ( 110.3436608795247764, -8.938348069036489818, -9.318865927141430916 ) ) ;
#19970=CARTESIAN_POINT ( 'NONE',  ( 112.2883483795247770, -0.7896495226426338832, -9.318865927141430916 ) ) ;
#19973=CARTESIAN_POINT ( 'NONE',  ( 116.2659068881580708, -12.01880880694303855, -4.893215200338314474 ) ) ;
#19986=CARTESIAN_POINT ( 'NONE',  ( 107.9822546295247889, -4.863998795839590272, -7.631215200338315796 ) ) ;
#19988=CARTESIAN_POINT ( 'NONE',  ( 112.2188952545247531, -9.868328341294098749, -15.46607636864997204 ) ) ;
#19990=CARTESIAN_POINT ( 'NONE',  ( 70.19189222814998175, -60.21979223295905825, -40.52181113153821457 ) ) ;
#20001=CARTESIAN_POINT ( 'NONE',  ( 114.1889176093651912, 0.5600166689815611054, -14.64321520033831447 ) ) ;
#20002=CARTESIAN_POINT ( 'NONE',  ( 106.1070202545248407, 0.1403307496149616695, -11.32035403202665336 ) ) ;
#20009=EDGE_CURVE ( 'NONE', #27061, #14735, #32792, .T. ) ;
#20019=CARTESIAN_POINT ( 'NONE',  ( 110.6214733795247867, -8.938348069036489818, -17.46756447353520159 ) ) ;
#20020=CARTESIAN_POINT ( 'NONE',  ( 106.8710046295248759, -4.863998795839590272, -18.39754474579285315 ) ) ;
#20021=CARTESIAN_POINT ( 'NONE',  ( 82.73277184789131411, -31.78424552905355327, -23.09918304670232558 ) ) ;
#20025=CARTESIAN_POINT ( 'NONE',  ( 112.7965408578216824, 0.04929351793716424401, -12.14321520033834467 ) ) ;
#20026=CARTESIAN_POINT ( 'NONE',  ( 114.3024890045248156, -9.868328341294098749, -11.32035403202665869 ) ) ;
#20028=CARTESIAN_POINT ( 'NONE',  ( 109.2293626546097158, -0.7401772152451036035, -16.31465090027937137 ) ) ;
#20036=CARTESIAN_POINT ( 'NONE',  ( 116.6056978591944642, -11.87337149029565175, -21.21309283736433571 ) ) ;
#20046=CARTESIAN_POINT ( 'NONE',  ( 113.8857702545248003, 0.1403307496149616695, -11.32035403202665336 ) ) ;
#20049=( BOUNDED_SURFACE ( )  B_SPLINE_SURFACE ( 1, 2, ( 
 ( #7194, #34981, #3112, #3767, #10856, #24751, #7412, #21332, #24099, #3991, #582, #6537, #20455, #44855, #37992, #6768, #11076, #8550, #7876, #24978, #36122, #32478, #1694, #4220, #15614, #38873, #18136, #7643, #39336, #39780, #42980, #1253, #1468, #25879, #25435, #18808, #11529, #22451, #28854, #14944, #21784, #29296, #29069, #8328, #19031, #11750, #15164, #29521, #4891, #11977, #18369, #21556, #1027, #36343, #35445, #801, #4666, #42767, #32032, #25658, #14719, #8104, #28631, #39563, #15393, #43209, #22004, #5114, #32699, #42539, #35900, #18588, #32918, #11300, #22227, #25209, #39107, #35674, #4449, #32258, #19265, #15846, #29741, #26329, #16067, #37246, #13106, #27009, #12201, #33595, #40929, #12428, #9681, #12659, #33367, #23598, #26556, #33144, #19707, #26786, #26099, #19941, #37019, #16301, #5789, #20178, #2829, #40236, #5564, #5348, #23140, #2370, #40695, #44347, #6257, #33830, #36571, #43652, #30202, #1916, #9003, #37484, #22902, #36795, #44121, #9449, #19484, #40470, #12887, #23363, #9230, #34062, #2137, #16757, #16529, #6018, #43437, #29973, #43889, #2599, #30428, #40004, #8769, #22675, #3281, #38159, #27241, #41825, #10585, #20840, #24483, #24047, #307, #24270, #85, #35165, #3720, #38372, #14220, #38588, #20402 ),
 ( #7145, #24700, #3942, #21056, #13337, #30654, #28136, #44572, #34933, #41387, #37717, #41156, #3503, #37940, #9917, #16986, #7366, #6715, #23830, #6487, #3059, #10363, #17640, #31537, #6934, #21280, #42043, #34719, #10141, #10804, #13997, #17420, #20626, #34286, #41604, #30878, #13779, #44798, #13556, #27466, #31095, #17203, #34502, #45021, #27690, #31311, #27914, #39284, #38824, #8050, #11482, #21954, #18763, #42491, #7593, #39512, #14667, #31762, #35845, #533, #745, #1420, #32653, #21508, #42715, #22402, #8500, #980, #39057, #4619, #29248, #4170, #28807, #31981, #43157, #1205, #15339, #25824, #28583, #11252, #18540, #15119, #25161, #14895, #32431, #29026, #25388, #11924, #18089, #36297, #36074, #42937, #17865, #4396, #35395, #11698, #18313, #22178, #39731, #35624, #32207, #25609, #14443, #8275, #4844, #28351, #42263, #7828, #11028, #24928, #21735, #9625, #23306, #12832, #19888, #13052, #39955, #23547, #5296, #23082, #26731, #36523, #44065, #44297, #5065, #40640, #32870, #18980, #2545, #1639, #16247, #15791, #12150, #15562, #36962, #12379, #29466, #19212, #26951, #43604, #43382, #26052, #22624, #29922, #30150, #9395, #12605, #40872, #37189, #43837, #29692, #5963, #33539, #5734, #26277, #33775, #16016, #16472, #33315, #30375, #8719 ) ),
 .UNSPECIFIED., .F., .F., .F. ) 
 B_SPLINE_SURFACE_WITH_KNOTS ( ( 2, 2 ),
 ( 3, 2, 2, 2, 2, 2, 2, 2, 2, 2, 2, 2, 2, 2, 2, 2, 2, 2, 2, 2, 2, 2, 2, 2, 2, 2, 2, 2, 2, 2, 2, 2, 2, 2, 2, 2, 2, 2, 2, 2, 2, 2, 2, 2, 2, 2, 2, 2, 2, 2, 2, 2, 2, 2, 2, 2, 2, 2, 2, 2, 2, 2, 2, 2, 2, 2, 2, 2, 2, 2, 2, 2, 2, 2, 2, 2, 2, 2, 2, 2, 3 ),
 ( 0.000000000000000000, 1.000000000000000000 ),
 ( 0.000000000000000000, 0.01250000000000000069, 0.02500000000000000139, 0.03749999999999999861, 0.05000000000000000278, 0.06250000000000000000, 0.07499999999999999722, 0.08749999999999999445, 0.1000000000000000056, 0.1125000000000000028, 0.1250000000000000000, 0.1375000000000000111, 0.1499999999999999944, 0.1625000000000000056, 0.1749999999999999889, 0.1875000000000000000, 0.2000000000000000111, 0.2124999999999999944, 0.2250000000000000056, 0.2374999999999999889, 0.2500000000000000000, 0.2625000000000000111, 0.2750000000000000222, 0.2874999999999999778, 0.2999999999999999889, 0.3125000000000000000, 0.3250000000000000111, 0.3375000000000000222, 0.3499999999999999778, 0.3624999999999999889, 0.3750000000000000000, 0.3875000000000000111, 0.4000000000000000222, 0.4124999999999999778, 0.4249999999999999889, 0.4375000000000000000, 0.4500000000000000111, 0.4625000000000000222, 0.4749999999999999778, 0.4874999999999999889, 0.5000000000000000000, 0.5124999999999999556, 0.5250000000000000222, 0.5374999999999999778, 0.5500000000000000444, 0.5625000000000000000, 0.5749999999999999556, 0.5875000000000000222, 0.5999999999999999778, 0.6125000000000000444, 0.6250000000000000000, 0.6374999999999999556, 0.6500000000000000222, 0.6624999999999999778, 0.6750000000000000444, 0.6875000000000000000, 0.6999999999999999556, 0.7125000000000000222, 0.7249999999999999778, 0.7375000000000000444, 0.7500000000000000000, 0.7624999999999999556, 0.7750000000000000222, 0.7874999999999999778, 0.8000000000000000444, 0.8125000000000000000, 0.8249999999999999556, 0.8375000000000000222, 0.8499999999999999778, 0.8625000000000000444, 0.8750000000000000000, 0.8874999999999999556, 0.9000000000000000222, 0.9124999999999999778, 0.9250000000000000444, 0.9375000000000000000, 0.9499999999999999556, 0.9625000000000000222, 0.9749999999999999778, 0.9875000000000000444, 1.000000000000000000 ),
 .UNSPECIFIED. ) 
 GEOMETRIC_REPRESENTATION_ITEM ( )  RATIONAL_B_SPLINE_SURFACE ( (
 ( 1.000000000000000000, 0.9238795325112869605, 1.000000000000000000, 0.9238795325112869605, 1.000000000000000000, 0.9238795325112869605, 1.000000000000000000, 0.9238795325112869605, 1.000000000000000000, 0.9238795325112869605, 1.000000000000000000, 0.9238795325112869605, 1.000000000000000000, 0.9238795325112869605, 1.000000000000000000, 0.9238795325112869605, 1.000000000000000000, 0.9238795325112869605, 1.000000000000000000, 0.9238795325112869605, 1.000000000000000000, 0.9238795325112869605, 1.000000000000000000, 0.9238795325112869605, 1.000000000000000000, 0.9238795325112869605, 1.000000000000000000, 0.9238795325112869605, 1.000000000000000000, 0.9238795325112869605, 1.000000000000000000, 0.9238795325112869605, 1.000000000000000000, 0.9238795325112869605, 1.000000000000000000, 0.9238795325112869605, 1.000000000000000000, 0.9238795325112869605, 1.000000000000000000, 0.9238795325112869605, 1.000000000000000000, 0.9238795325112869605, 1.000000000000000000, 0.9238795325112869605, 1.000000000000000000, 0.9238795325112869605, 1.000000000000000000, 0.9238795325112869605, 1.000000000000000000, 0.9238795325112869605, 1.000000000000000000, 0.9238795325112869605, 1.000000000000000000, 0.9238795325112869605, 1.000000000000000000, 0.9238795325112869605, 1.000000000000000000, 0.9238795325112869605, 1.000000000000000000, 0.9238795325112869605, 1.000000000000000000, 0.9238795325112869605, 1.000000000000000000, 0.9238795325112869605, 1.000000000000000000, 0.9238795325112869605, 1.000000000000000000, 0.9238795325112869605, 1.000000000000000000, 0.9238795325112869605, 1.000000000000000000, 0.9238795325112869605, 1.000000000000000000, 0.9238795325112869605, 1.000000000000000000, 0.9238795325112869605, 1.000000000000000000, 0.9238795325112869605, 1.000000000000000000, 0.9238795325112869605, 1.000000000000000000, 0.9238795325112869605, 1.000000000000000000, 0.9238795325112869605, 1.000000000000000000, 0.9238795325112869605, 1.000000000000000000, 0.9238795325112869605, 1.000000000000000000, 0.9238795325112869605, 1.000000000000000000, 0.9238795325112869605, 1.000000000000000000, 0.9238795325112869605, 1.000000000000000000, 0.9238795325112869605, 1.000000000000000000, 0.9238795325112869605, 1.000000000000000000, 0.9238795325112869605, 1.000000000000000000, 0.9238795325112869605, 1.000000000000000000, 0.9238795325112869605, 1.000000000000000000, 0.9238795325112869605, 1.000000000000000000, 0.9238795325112869605, 1.000000000000000000, 0.9238795325112869605, 1.000000000000000000, 0.9238795325112869605, 1.000000000000000000, 0.9238795325112869605, 1.000000000000000000, 0.9238795325112869605, 1.000000000000000000, 0.9238795325112869605, 1.000000000000000000, 0.9238795325112869605, 1.000000000000000000, 0.9238795325112869605, 1.000000000000000000, 0.9238795325112869605, 1.000000000000000000, 0.9238795325112869605, 1.000000000000000000, 0.9238795325112869605, 1.000000000000000000, 0.9238795325112869605, 1.000000000000000000, 0.9238795325112869605, 1.000000000000000000, 0.9238795325112869605, 1.000000000000000000, 0.9238795325112869605, 1.000000000000000000, 0.9238795325112869605, 1.000000000000000000, 0.9238795325112869605, 1.000000000000000000, 0.9238795325112869605, 1.000000000000000000, 0.9238795325112869605, 1.000000000000000000, 0.9238795325112869605, 1.000000000000000000, 0.9238795325112869605, 1.000000000000000000, 0.9238795325112869605, 1.000000000000000000, 0.9238795325112869605, 1.000000000000000000, 0.9238795325112869605, 1.000000000000000000, 0.9238795325112869605, 1.000000000000000000, 0.9238795325112869605, 1.000000000000000000, 0.9238795325112869605, 1.000000000000000000),
 ( 1.000000000000000000, 0.9238795325112869605, 1.000000000000000000, 0.9238795325112869605, 1.000000000000000000, 0.9238795325112869605, 1.000000000000000000, 0.9238795325112869605, 1.000000000000000000, 0.9238795325112869605, 1.000000000000000000, 0.9238795325112869605, 1.000000000000000000, 0.9238795325112869605, 1.000000000000000000, 0.9238795325112869605, 1.000000000000000000, 0.9238795325112869605, 1.000000000000000000, 0.9238795325112869605, 1.000000000000000000, 0.9238795325112869605, 1.000000000000000000, 0.9238795325112869605, 1.000000000000000000, 0.9238795325112869605, 1.000000000000000000, 0.9238795325112869605, 1.000000000000000000, 0.9238795325112869605, 1.000000000000000000, 0.9238795325112869605, 1.000000000000000000, 0.9238795325112869605, 1.000000000000000000, 0.9238795325112869605, 1.000000000000000000, 0.9238795325112869605, 1.000000000000000000, 0.9238795325112869605, 1.000000000000000000, 0.9238795325112869605, 1.000000000000000000, 0.9238795325112869605, 1.000000000000000000, 0.9238795325112869605, 1.000000000000000000, 0.9238795325112869605, 1.000000000000000000, 0.9238795325112869605, 1.000000000000000000, 0.9238795325112869605, 1.000000000000000000, 0.9238795325112869605, 1.000000000000000000, 0.9238795325112869605, 1.000000000000000000, 0.9238795325112869605, 1.000000000000000000, 0.9238795325112869605, 1.000000000000000000, 0.9238795325112869605, 1.000000000000000000, 0.9238795325112869605, 1.000000000000000000, 0.9238795325112869605, 1.000000000000000000, 0.9238795325112869605, 1.000000000000000000, 0.9238795325112869605, 1.000000000000000000, 0.9238795325112869605, 1.000000000000000000, 0.9238795325112869605, 1.000000000000000000, 0.9238795325112869605, 1.000000000000000000, 0.9238795325112869605, 1.000000000000000000, 0.9238795325112869605, 1.000000000000000000, 0.9238795325112869605, 1.000000000000000000, 0.9238795325112869605, 1.000000000000000000, 0.9238795325112869605, 1.000000000000000000, 0.9238795325112869605, 1.000000000000000000, 0.9238795325112869605, 1.000000000000000000, 0.9238795325112869605, 1.000000000000000000, 0.9238795325112869605, 1.000000000000000000, 0.9238795325112869605, 1.000000000000000000, 0.9238795325112869605, 1.000000000000000000, 0.9238795325112869605, 1.000000000000000000, 0.9238795325112869605, 1.000000000000000000, 0.9238795325112869605, 1.000000000000000000, 0.9238795325112869605, 1.000000000000000000, 0.9238795325112869605, 1.000000000000000000, 0.9238795325112869605, 1.000000000000000000, 0.9238795325112869605, 1.000000000000000000, 0.9238795325112869605, 1.000000000000000000, 0.9238795325112869605, 1.000000000000000000, 0.9238795325112869605, 1.000000000000000000, 0.9238795325112869605, 1.000000000000000000, 0.9238795325112869605, 1.000000000000000000, 0.9238795325112869605, 1.000000000000000000, 0.9238795325112869605, 1.000000000000000000, 0.9238795325112869605, 1.000000000000000000, 0.9238795325112869605, 1.000000000000000000, 0.9238795325112869605, 1.000000000000000000, 0.9238795325112869605, 1.000000000000000000, 0.9238795325112869605, 1.000000000000000000, 0.9238795325112869605, 1.000000000000000000, 0.9238795325112869605, 1.000000000000000000, 0.9238795325112869605, 1.000000000000000000, 0.9238795325112869605, 1.000000000000000000, 0.9238795325112869605, 1.000000000000000000, 0.9238795325112869605, 1.000000000000000000, 0.9238795325112869605, 1.000000000000000000, 0.9238795325112869605, 1.000000000000000000, 0.9238795325112869605, 1.000000000000000000, 0.9238795325112869605, 1.000000000000000000, 0.9238795325112869605, 1.000000000000000000, 0.9238795325112869605, 1.000000000000000000) ) ) 
 REPRESENTATION_ITEM ( '' )  SURFACE ( )  );
#20059=LINE ( 'NONE', #6824, #18691 ) ;
#20075=ORIENTED_EDGE ( 'NONE', *, *, #12095, .T. ) ;
#20077=CARTESIAN_POINT ( 'NONE',  ( 111.1770983795247787, -0.7896495226426338832, -9.318865927141430916 ) ) ;
#20078=CARTESIAN_POINT ( 'NONE',  ( 105.6903015045248253, -6.936859964151250502, -18.39754474579286025 ) ) ;
#20079=CARTESIAN_POINT ( 'NONE',  ( 105.8986608795248401, -1.325403438956436419, -16.93181055722141792 ) ) ;
#20083=DIRECTION ( 'NONE',  ( 0.000000000000000000, 0.000000000000000000, -1.000000000000000000 ) ) ;
#20084=CARTESIAN_POINT ( 'NONE',  ( 117.2294421295247844, -10.72535413672978599, -21.89321520033831447 ) ) ;
#20089=CARTESIAN_POINT ( 'NONE',  ( 114.4413952545248350, -9.868328341294098749, -15.46607636864997204 ) ) ;
#20110=CARTESIAN_POINT ( 'NONE',  ( 113.4690515045247992, -2.477300249445798297, -7.631215200338321125 ) ) ;
#20118=ADVANCED_FACE ( 'NONE', ( #41473 ), #33707, .T. ) ;
#20121=AXIS2_PLACEMENT_3D ( 'NONE', #10971, #36020, #21898 ) ;
#20129=VECTOR ( 'NONE', #38512, 1000.000000000000000 ) ;
#20133=CARTESIAN_POINT ( 'NONE',  ( 110.0658483795247804, -0.7896495226426338832, -9.318865927141430916 ) ) ;
#20134=CARTESIAN_POINT ( 'NONE',  ( 112.5661608795247872, -1.325403438956436419, -16.93181055722141792 ) ) ;
#20135=CARTESIAN_POINT ( 'NONE',  ( 109.0240515045248202, -2.477300249445798297, -7.631215200338321125 ) ) ;
#20155=CARTESIAN_POINT ( 'NONE',  ( 107.7738952545248310, -9.868328341294098749, -15.46607636864997204 ) ) ;
#20156=CARTESIAN_POINT ( 'NONE',  ( 110.0658483795247804, -8.402594152722688392, -16.93181055722141792 ) ) ;
#20158=DIRECTION ( 'NONE',  ( 0.000000000000000000, 0.000000000000000000, -1.000000000000000000 ) ) ;
#20161=ORIENTED_EDGE ( 'NONE', *, *, #24744, .F. ) ;
#20178=CARTESIAN_POINT ( 'NONE',  ( 109.8574890045247940, -9.868328341294098749, -11.32035403202665869 ) ) ;
#20189=CARTESIAN_POINT ( 'NONE',  ( 114.0502378519202864, 0.2518737723193609224, -12.14321520033831625 ) ) ;
#20195=DIRECTION ( 'NONE',  ( -1.000000000000000000, 0.000000000000000000, 0.000000000000000000 ) ) ;
#20196=CARTESIAN_POINT ( 'NONE',  ( 115.1359265045248605, -7.250697342233347165, -19.15521520033831138 ) ) ;
#20200=CARTESIAN_POINT ( 'NONE',  ( 114.8581140045248361, 0.1403307496149616695, -15.46607636864997204 ) ) ;
#20202=CARTESIAN_POINT ( 'NONE',  ( 109.2295511504564303, -2.582258012937524327, -17.92986911656043247 ) ) ;
#20204=CARTESIAN_POINT ( 'NONE',  ( 105.5513952545248060, 0.8980012041604421569, -11.00651665394454071 ) ) ;
#20206=CARTESIAN_POINT ( 'NONE',  ( 115.5526452545247622, 0.8980012041604421569, -11.00651665394454071 ) ) ;
#20209=CARTESIAN_POINT ( 'NONE',  ( 115.2748327545248657, -2.477300249445798297, -19.15521520033830427 ) ) ;
#20218=ORIENTED_EDGE ( 'NONE', *, *, #7534, .T. ) ;
#20220=CARTESIAN_POINT ( 'NONE',  ( 106.3153796295248412, -4.863998795839590272, -19.15521520033831493 ) ) ;
#20221=CARTESIAN_POINT ( 'NONE',  ( 111.3854577545248645, -2.791137627527939813, -18.39754474579286025 ) ) ;
#20224=CARTESIAN_POINT ( 'NONE',  ( 112.9828796295247884, -4.863998795839590272, -19.15521520033831493 ) ) ;
#20228=CARTESIAN_POINT ( 'NONE',  ( 63.10250807381770244, -31.76310523276723430, -22.89321520033831803 ) ) ;
#20229=CARTESIAN_POINT ( 'NONE',  ( 112.7982045411902163, -0.3595008806742185925, -10.82052240173743130 ) ) ;
#20231=CARTESIAN_POINT ( 'NONE',  ( 116.2048035453898223, 2.307602176693129614, -6.673484833205728606 ) ) ;
#20233=CARTESIAN_POINT ( 'NONE',  ( 107.4266296295248821, -4.863998795839590272, -8.388885654883775800 ) ) ;
#20248=CARTESIAN_POINT ( 'NONE',  ( 112.0799890045248475, 0.8980012041604421569, -15.77991374673208469 ) ) ;
#20249=LINE ( 'NONE', #37330, #38028 ) ;
#20250=CARTESIAN_POINT ( 'NONE',  ( 116.5249890045247980, 0.8980012041604421569, -15.77991374673208469 ) ) ;
#20254=CARTESIAN_POINT ( 'NONE',  ( 112.2188952545247531, -9.868328341294098749, -15.46607636864997204 ) ) ;
#20261=VERTEX_POINT ( 'NONE', #6808 ) ;
#20268=SHAPE_REPRESENTATION_RELATIONSHIP ( 'NONE' , 'NONE' ,  #15458, #41161 ) ;
#20269=DIRECTION ( 'NONE',  ( 0.4649787261689617424, 0.8853218534579895271, 0.000000000000000000 ) ) ;
#20272=CARTESIAN_POINT ( 'NONE',  ( 106.4542858795248179, -8.402594152722688392, -9.854619843455216355 ) ) ;
#20274=PLANE ( 'NONE',  #2419 ) ;
#20285=CARTESIAN_POINT ( 'NONE',  ( 78.46442941731035603, -58.56046118940295742, -0.3236597056445599807 ) ) ;
#20289=CARTESIAN_POINT ( 'NONE',  ( 66.82415148905926117, -40.21211973637273474, -21.89321520033831447 ) ) ;
#20299=CARTESIAN_POINT ( 'NONE',  ( 106.1764733795248219, -8.938348069036489818, -17.46756447353520159 ) ) ;
#20301=CARTESIAN_POINT ( 'NONE',  ( 107.7738952545248310, -9.868328341294098749, -15.46607636864997204 ) ) ;
#20302=CARTESIAN_POINT ( 'NONE',  ( 105.6903015045248253, -6.936859964151250502, -18.39754474579286025 ) ) ;
#20303=CARTESIAN_POINT ( 'NONE',  ( 109.3713171295247832, -10.62599879583958540, -13.39321520033830382 ) ) ;
#20305=VERTEX_POINT ( 'NONE', #3157 ) ;
#20311=EDGE_CURVE ( 'NONE', #40384, #14664, #2695, .T. ) ;
#20312=CARTESIAN_POINT ( 'NONE',  ( 108.0517077545248696, -7.250697342233347165, -7.631215200338321125 ) ) ;
#20325=EDGE_CURVE ( 'NONE', #9951, #31450, #24267, .T. ) ;
#20326=DIRECTION ( 'NONE',  ( 1.000000000000000000, 0.000000000000000000, 0.000000000000000000 ) ) ;
#20336=CARTESIAN_POINT ( 'NONE',  ( 110.3436608795247764, -8.938348069036489818, -9.318865927141430916 ) ) ;
#20339=ORIENTED_EDGE ( 'NONE', *, *, #14202, .T. ) ;
#20357=CARTESIAN_POINT ( 'NONE',  ( 107.4266296295248821, -4.863998795839590272, -19.15521520033831493 ) ) ;
#20358=CARTESIAN_POINT ( 'NONE',  ( 115.4137390045248566, -9.868328341294098749, -11.32035403202665869 ) ) ;
#20359=CARTESIAN_POINT ( 'NONE',  ( 107.6349890045248401, 0.8980012041604421569, -15.77991374673208469 ) ) ;
#20371=CARTESIAN_POINT ( 'NONE',  ( 114.2330358795247776, -8.402594152722688392, -9.854619843455216355 ) ) ;
#20372=ORIENTED_EDGE ( 'NONE', *, *, #7203, .T. ) ;
#20377=CARTESIAN_POINT ( 'NONE',  ( 106.3153796295248412, -4.863998795839590272, -8.388885654883775800 ) ) ;
#20378=CARTESIAN_POINT ( 'NONE',  ( 106.5237390045248418, -9.868328341294098749, -11.32035403202665869 ) ) ;
#20388=ORIENTED_EDGE ( 'NONE', *, *, #35586, .T. ) ;
#20391=EDGE_CURVE ( 'NONE', #25821, #12113, #18580, .T. ) ;
#20393=EDGE_CURVE ( 'NONE', #17270, #34946, #44679, .T. ) ;
#20402=CARTESIAN_POINT ( 'NONE',  ( 106.0375671295248310, 0.1403307496149613920, -13.39321520033831447 ) ) ;
#20411=CARTESIAN_POINT ( 'NONE',  ( 112.5661608795247872, -8.938348069036489818, -9.318865927141430916 ) ) ;
#20413=CARTESIAN_POINT ( 'NONE',  ( 65.68057756587693063, -37.02887214625545909, -5.220056341857074678 ) ) ;
#20417=VECTOR ( 'NONE', #30478, 999.9999999999998863 ) ;
#20420=CARTESIAN_POINT ( 'NONE',  ( 116.4555358795247884, -0.7896495226426338832, -17.46756447353520159 ) ) ;
#20423=DIRECTION ( 'NONE',  ( 1.000000000000000000, 0.000000000000000000, 0.000000000000000000 ) ) ;
#20424=CARTESIAN_POINT ( 'NONE',  ( 114.5803015045248117, -6.936859964151250502, -18.39754474579286025 ) ) ;
#20428=DIRECTION ( 'NONE',  ( 1.000000000000000000, 0.000000000000000000, 0.000000000000000000 ) ) ;
#20430=CARTESIAN_POINT ( 'NONE',  ( 112.9828796295247884, -4.863998795839590272, -19.15521520033831493 ) ) ;
#20433=CARTESIAN_POINT ( 'NONE',  ( 115.0664733795247798, -8.938348069036441856, -17.46756447353520514 ) ) ;
#20444=ORIENTED_EDGE ( 'NONE', *, *, #9982, .T. ) ;
#20450=CARTESIAN_POINT ( 'NONE',  ( 111.5243640045248412, -10.62599879583958717, -11.00651665394454604 ) ) ;
#20455=CARTESIAN_POINT ( 'NONE',  ( 116.3166296295247832, -4.863998795839590272, -8.388885654883775800 ) ) ;
#20456=CARTESIAN_POINT ( 'NONE',  ( 76.69189222814998175, -49.76310523276723785, -19.39321520033831447 ) ) ;
#20459=CARTESIAN_POINT ( 'NONE',  ( 105.1346765045248475, -2.791137627527939813, -8.388885654883777576 ) ) ;
#20460=CARTESIAN_POINT ( 'NONE',  ( 86.50830818076254047, -21.65036132658698520, -21.89321520033831447 ) ) ;
#20464=ADVANCED_FACE ( 'NONE', ( #33840 ), #30083, .F. ) ;
#20473=CARTESIAN_POINT ( 'NONE',  ( 111.5243640045248412, -10.62599879583958717, -11.00651665394454604 ) ) ;
#20474=DIRECTION ( 'NONE',  ( -0.1736481776669309696, -0.9848077530122079093, 0.000000000000000000 ) ) ;
#20475=CARTESIAN_POINT ( 'NONE',  ( 115.4831921295247952, 0.8980012041604618078, -13.39321520033831447 ) ) ;
#20481=CARTESIAN_POINT ( 'NONE',  ( 108.1211608795247798, -1.325403438956436419, -16.93181055722141792 ) ) ;
#20482=ORIENTED_EDGE ( 'NONE', *, *, #45135, .F. ) ;
#20483=CIRCLE ( 'NONE', #16070, 10.00000000000000000 ) ;
#20484=CARTESIAN_POINT ( 'NONE',  ( 87.44708369096657918, -23.44614552640564042, -8.393215200338314474 ) ) ;
#20490=CARTESIAN_POINT ( 'NONE',  ( 113.7468640045248094, -10.62599879583958540, -11.00651665394455492 ) ) ;
#20498=CARTESIAN_POINT ( 'NONE',  ( 107.3571765045248299, -2.791137627527939813, -8.388885654883777576 ) ) ;
#20503=ORIENTED_EDGE ( 'NONE', *, *, #3058, .F. ) ;
#20512=CARTESIAN_POINT ( 'NONE',  ( 78.03418817537199459, -57.63411461863086060, -0.9907621434124950222 ) ) ;
#20524=CARTESIAN_POINT ( 'NONE',  ( 106.1070202545248407, -10.62599879583958717, -15.77991374673208469 ) ) ;
#20525=DIRECTION ( 'NONE',  ( 0.000000000000000000, 0.000000000000000000, 1.000000000000000000 ) ) ;
#20528=CARTESIAN_POINT ( 'NONE',  ( 64.33303459182538120, -36.44494369579175697, -5.635745537283291640 ) ) ;
#20535=CARTESIAN_POINT ( 'NONE',  ( 107.9128015045248219, -2.477300249445798297, -7.631215200338321125 ) ) ;
#20537=ORIENTED_EDGE ( 'NONE', *, *, #9989, .F. ) ;
#20539=CIRCLE ( 'NONE', #6706, 15.90000000000000036 ) ;
#20556=CARTESIAN_POINT ( 'NONE',  ( 109.6491296295247793, -4.863998795839590272, -19.15521520033831493 ) ) ;
#20559=VERTEX_POINT ( 'NONE', #8689 ) ;
#20579=CARTESIAN_POINT ( 'NONE',  ( 106.4542858795248179, -0.7896495226426338832, -17.46756447353520159 ) ) ;
#20580=CARTESIAN_POINT ( 'NONE',  ( 107.3571765045248299, -2.791137627527939813, -8.388885654883777576 ) ) ;
#20581=CARTESIAN_POINT ( 'NONE',  ( 107.8433483795247838, -0.7896495226426338832, -9.318865927141430916 ) ) ;
#20584=VERTEX_POINT ( 'NONE', #30121 ) ;
#20585=EDGE_CURVE ( 'NONE', #14378, #16340, #22073, .T. ) ;
#20587=CARTESIAN_POINT ( 'NONE',  ( 111.1076452545248259, 0.8980012041604421569, -11.00651665394454071 ) ) ;
#20590=( BOUNDED_SURFACE ( )  B_SPLINE_SURFACE ( 1, 2, ( 
 ( #39371, #36604, #19296, #1951, #35933, #4701, #30230, #36825, #40958, #40499, #12460, #16560, #26361, #5594, #6285, #20206, #5820, #43685, #30002, #6515, #12687, #37049, #27041, #16788, #30455, #40268, #9713, #9260, #27271, #19518, #41185, #34091, #16099, #23170, #16328, #37280, #44375, #9035, #22932, #37745, #17014, #13366, #23859, #19740, #23626, #30684, #26586, #9945, #37512, #13137, #33624, #33395, #20430, #6047, #3087, #2169, #2400, #44152, #43918, #2627, #12917, #2857, #19970, #33858, #34314, #26813, #40724, #9481, #23394, #44603, #14472, #27495, #3748, #21312, #41415, #115, #28164, #562, #27719, #21083, #7622, #4199, #7394, #38400, #28380, #34960, #20870, #17670, #13808, #30905, #13585, #24299, #11055, #38186, #10612, #3309, #6745, #44827, #6963, #34531, #10169, #31566, #17232, #34748, #45048, #31123, #41634, #24729, #42074, #10390, #3971, #38617, #42293, #3530, #35195, #14028, #37969, #17446, #31341, #27942, #24076, #335, #35423, #20654, #41852, #31790, #17893, #24515, #7173, #14248, #10832, #24958, #38854, #21536, #18567, #29275, #25189, #4874, #8083, #39759, #18792, #29497, #39087, #14924, #29053, #8529, #15146, #22431, #11727, #26079, #14697, #18117, #42960, #7856, #39983, #15371, #43191, #25853, #1450, #8305, #12178 ),
 ( #39314, #36324, #11955, #5093, #15594, #25641, #1671, #19009, #39544, #21985, #32895, #43411, #4428, #11510, #22207, #36103, #32681, #28835, #8748, #28611, #42520, #22654, #35654, #36550, #21762, #32010, #35874, #774, #18344, #11281, #32237, #1008, #42745, #25414, #4645, #32459, #1234, #2808, #13087, #29952, #44328, #26985, #36772, #40905, #23116, #26764, #19460, #30631, #44099, #15820, #41136, #30181, #1892, #9659, #29719, #23579, #6234, #12864, #19684, #33572, #33343, #36993, #40673, #9895, #5324, #2116, #5763, #22878, #9425, #9207, #5997, #23338, #37223, #27218, #8980, #16046, #2348, #16279, #19920, #34039, #43632, #33806, #37461, #12406, #2577, #16507, #20156, #43867, #30406, #23807, #19240, #16735, #44547, #13311, #33123, #40445, #26307, #12639, #40215, #5543, #26535, #17840, #45000, #17401, #10123, #13537, #11004, #13760, #41367, #38350, #38138, #63, #3485, #24458, #27669, #13976, #10561, #3039, #42017, #31290, #31513, #17183, #16961, #285, #6909, #42240, #44778, #27445, #37695, #6468, #28113, #41582, #21261, #27889, #7126, #20819, #30855, #20378, #10782, #3921, #24245, #34698, #41803, #21037, #24026, #34910, #34479, #34264, #3700, #37915, #6692, #14195, #24678, #10341, #20604, #3258, #507, #31073, #17620, #38566, #7342 ) ),
 .UNSPECIFIED., .F., .F., .T. ) 
 B_SPLINE_SURFACE_WITH_KNOTS ( ( 2, 2 ),
 ( 3, 2, 2, 2, 2, 2, 2, 2, 2, 2, 2, 2, 2, 2, 2, 2, 2, 2, 2, 2, 2, 2, 2, 2, 2, 2, 2, 2, 2, 2, 2, 2, 2, 2, 2, 2, 2, 2, 2, 2, 2, 2, 2, 2, 2, 2, 2, 2, 2, 2, 2, 2, 2, 2, 2, 2, 2, 2, 2, 2, 2, 2, 2, 2, 2, 2, 2, 2, 2, 2, 2, 2, 2, 2, 2, 2, 2, 2, 2, 2, 3 ),
 ( 0.000000000000000000, 1.000000000000000000 ),
 ( 0.000000000000000000, 0.01250000000000000069, 0.02500000000000000139, 0.03749999999999999861, 0.05000000000000000278, 0.06250000000000000000, 0.07499999999999999722, 0.08749999999999999445, 0.1000000000000000056, 0.1125000000000000028, 0.1250000000000000000, 0.1375000000000000111, 0.1499999999999999944, 0.1625000000000000056, 0.1749999999999999889, 0.1875000000000000000, 0.2000000000000000111, 0.2124999999999999944, 0.2250000000000000056, 0.2374999999999999889, 0.2500000000000000000, 0.2625000000000000111, 0.2750000000000000222, 0.2874999999999999778, 0.2999999999999999889, 0.3125000000000000000, 0.3250000000000000111, 0.3375000000000000222, 0.3499999999999999778, 0.3624999999999999889, 0.3750000000000000000, 0.3875000000000000111, 0.4000000000000000222, 0.4124999999999999778, 0.4249999999999999889, 0.4375000000000000000, 0.4500000000000000111, 0.4625000000000000222, 0.4749999999999999778, 0.4874999999999999889, 0.5000000000000000000, 0.5124999999999999556, 0.5250000000000000222, 0.5374999999999999778, 0.5500000000000000444, 0.5625000000000000000, 0.5749999999999999556, 0.5875000000000000222, 0.5999999999999999778, 0.6125000000000000444, 0.6250000000000000000, 0.6374999999999999556, 0.6500000000000000222, 0.6624999999999999778, 0.6750000000000000444, 0.6875000000000000000, 0.6999999999999999556, 0.7125000000000000222, 0.7249999999999999778, 0.7375000000000000444, 0.7500000000000000000, 0.7624999999999999556, 0.7750000000000000222, 0.7874999999999999778, 0.8000000000000000444, 0.8125000000000000000, 0.8249999999999999556, 0.8375000000000000222, 0.8499999999999999778, 0.8625000000000000444, 0.8750000000000000000, 0.8874999999999999556, 0.9000000000000000222, 0.9124999999999999778, 0.9250000000000000444, 0.9375000000000000000, 0.9499999999999999556, 0.9625000000000000222, 0.9749999999999999778, 0.9875000000000000444, 1.000000000000000000 ),
 .UNSPECIFIED. ) 
 GEOMETRIC_REPRESENTATION_ITEM ( )  RATIONAL_B_SPLINE_SURFACE ( (
 ( 1.000000000000000000, 0.9238795325112869605, 1.000000000000000000, 0.9238795325112869605, 1.000000000000000000, 0.9238795325112869605, 1.000000000000000000, 0.9238795325112869605, 1.000000000000000000, 0.9238795325112869605, 1.000000000000000000, 0.9238795325112869605, 1.000000000000000000, 0.9238795325112869605, 1.000000000000000000, 0.9238795325112869605, 1.000000000000000000, 0.9238795325112869605, 1.000000000000000000, 0.9238795325112869605, 1.000000000000000000, 0.9238795325112869605, 1.000000000000000000, 0.9238795325112869605, 1.000000000000000000, 0.9238795325112869605, 1.000000000000000000, 0.9238795325112869605, 1.000000000000000000, 0.9238795325112869605, 1.000000000000000000, 0.9238795325112869605, 1.000000000000000000, 0.9238795325112869605, 1.000000000000000000, 0.9238795325112869605, 1.000000000000000000, 0.9238795325112869605, 1.000000000000000000, 0.9238795325112869605, 1.000000000000000000, 0.9238795325112869605, 1.000000000000000000, 0.9238795325112869605, 1.000000000000000000, 0.9238795325112869605, 1.000000000000000000, 0.9238795325112869605, 1.000000000000000000, 0.9238795325112869605, 1.000000000000000000, 0.9238795325112869605, 1.000000000000000000, 0.9238795325112869605, 1.000000000000000000, 0.9238795325112869605, 1.000000000000000000, 0.9238795325112869605, 1.000000000000000000, 0.9238795325112869605, 1.000000000000000000, 0.9238795325112869605, 1.000000000000000000, 0.9238795325112869605, 1.000000000000000000, 0.9238795325112869605, 1.000000000000000000, 0.9238795325112869605, 1.000000000000000000, 0.9238795325112869605, 1.000000000000000000, 0.9238795325112869605, 1.000000000000000000, 0.9238795325112869605, 1.000000000000000000, 0.9238795325112869605, 1.000000000000000000, 0.9238795325112869605, 1.000000000000000000, 0.9238795325112869605, 1.000000000000000000, 0.9238795325112869605, 1.000000000000000000, 0.9238795325112869605, 1.000000000000000000, 0.9238795325112869605, 1.000000000000000000, 0.9238795325112869605, 1.000000000000000000, 0.9238795325112869605, 1.000000000000000000, 0.9238795325112869605, 1.000000000000000000, 0.9238795325112869605, 1.000000000000000000, 0.9238795325112869605, 1.000000000000000000, 0.9238795325112869605, 1.000000000000000000, 0.9238795325112869605, 1.000000000000000000, 0.9238795325112869605, 1.000000000000000000, 0.9238795325112869605, 1.000000000000000000, 0.9238795325112869605, 1.000000000000000000, 0.9238795325112869605, 1.000000000000000000, 0.9238795325112869605, 1.000000000000000000, 0.9238795325112869605, 1.000000000000000000, 0.9238795325112869605, 1.000000000000000000, 0.9238795325112869605, 1.000000000000000000, 0.9238795325112869605, 1.000000000000000000, 0.9238795325112869605, 1.000000000000000000, 0.9238795325112869605, 1.000000000000000000, 0.9238795325112869605, 1.000000000000000000, 0.9238795325112869605, 1.000000000000000000, 0.9238795325112869605, 1.000000000000000000, 0.9238795325112869605, 1.000000000000000000, 0.9238795325112869605, 1.000000000000000000, 0.9238795325112869605, 1.000000000000000000, 0.9238795325112869605, 1.000000000000000000, 0.9238795325112869605, 1.000000000000000000, 0.9238795325112869605, 1.000000000000000000, 0.9238795325112869605, 1.000000000000000000, 0.9238795325112869605, 1.000000000000000000, 0.9238795325112869605, 1.000000000000000000, 0.9238795325112869605, 1.000000000000000000, 0.9238795325112869605, 1.000000000000000000, 0.9238795325112869605, 1.000000000000000000, 0.9238795325112869605, 1.000000000000000000, 0.9238795325112869605, 1.000000000000000000, 0.9238795325112869605, 1.000000000000000000, 0.9238795325112869605, 1.000000000000000000),
 ( 1.000000000000000000, 0.9238795325112869605, 1.000000000000000000, 0.9238795325112869605, 1.000000000000000000, 0.9238795325112869605, 1.000000000000000000, 0.9238795325112869605, 1.000000000000000000, 0.9238795325112869605, 1.000000000000000000, 0.9238795325112869605, 1.000000000000000000, 0.9238795325112869605, 1.000000000000000000, 0.9238795325112869605, 1.000000000000000000, 0.9238795325112869605, 1.000000000000000000, 0.9238795325112869605, 1.000000000000000000, 0.9238795325112869605, 1.000000000000000000, 0.9238795325112869605, 1.000000000000000000, 0.9238795325112869605, 1.000000000000000000, 0.9238795325112869605, 1.000000000000000000, 0.9238795325112869605, 1.000000000000000000, 0.9238795325112869605, 1.000000000000000000, 0.9238795325112869605, 1.000000000000000000, 0.9238795325112869605, 1.000000000000000000, 0.9238795325112869605, 1.000000000000000000, 0.9238795325112869605, 1.000000000000000000, 0.9238795325112869605, 1.000000000000000000, 0.9238795325112869605, 1.000000000000000000, 0.9238795325112869605, 1.000000000000000000, 0.9238795325112869605, 1.000000000000000000, 0.9238795325112869605, 1.000000000000000000, 0.9238795325112869605, 1.000000000000000000, 0.9238795325112869605, 1.000000000000000000, 0.9238795325112869605, 1.000000000000000000, 0.9238795325112869605, 1.000000000000000000, 0.9238795325112869605, 1.000000000000000000, 0.9238795325112869605, 1.000000000000000000, 0.9238795325112869605, 1.000000000000000000, 0.9238795325112869605, 1.000000000000000000, 0.9238795325112869605, 1.000000000000000000, 0.9238795325112869605, 1.000000000000000000, 0.9238795325112869605, 1.000000000000000000, 0.9238795325112869605, 1.000000000000000000, 0.9238795325112869605, 1.000000000000000000, 0.9238795325112869605, 1.000000000000000000, 0.9238795325112869605, 1.000000000000000000, 0.9238795325112869605, 1.000000000000000000, 0.9238795325112869605, 1.000000000000000000, 0.9238795325112869605, 1.000000000000000000, 0.9238795325112869605, 1.000000000000000000, 0.9238795325112869605, 1.000000000000000000, 0.9238795325112869605, 1.000000000000000000, 0.9238795325112869605, 1.000000000000000000, 0.9238795325112869605, 1.000000000000000000, 0.9238795325112869605, 1.000000000000000000, 0.9238795325112869605, 1.000000000000000000, 0.9238795325112869605, 1.000000000000000000, 0.9238795325112869605, 1.000000000000000000, 0.9238795325112869605, 1.000000000000000000, 0.9238795325112869605, 1.000000000000000000, 0.9238795325112869605, 1.000000000000000000, 0.9238795325112869605, 1.000000000000000000, 0.9238795325112869605, 1.000000000000000000, 0.9238795325112869605, 1.000000000000000000, 0.9238795325112869605, 1.000000000000000000, 0.9238795325112869605, 1.000000000000000000, 0.9238795325112869605, 1.000000000000000000, 0.9238795325112869605, 1.000000000000000000, 0.9238795325112869605, 1.000000000000000000, 0.9238795325112869605, 1.000000000000000000, 0.9238795325112869605, 1.000000000000000000, 0.9238795325112869605, 1.000000000000000000, 0.9238795325112869605, 1.000000000000000000, 0.9238795325112869605, 1.000000000000000000, 0.9238795325112869605, 1.000000000000000000, 0.9238795325112869605, 1.000000000000000000, 0.9238795325112869605, 1.000000000000000000, 0.9238795325112869605, 1.000000000000000000, 0.9238795325112869605, 1.000000000000000000, 0.9238795325112869605, 1.000000000000000000, 0.9238795325112869605, 1.000000000000000000, 0.9238795325112869605, 1.000000000000000000, 0.9238795325112869605, 1.000000000000000000, 0.9238795325112869605, 1.000000000000000000, 0.9238795325112869605, 1.000000000000000000, 0.9238795325112869605, 1.000000000000000000) ) ) 
 REPRESENTATION_ITEM ( '' )  SURFACE ( )  );
#20591=EDGE_CURVE ( 'NONE', #35835, #43568, #5304, .T. ) ;
#20597=CARTESIAN_POINT ( 'NONE',  ( 114.6497546295247929, -4.863998795839590272, -18.39754474579285315 ) ) ;
#20603=CARTESIAN_POINT ( 'NONE',  ( 107.4960827545248350, -6.936859964151250502, -8.388885654883777576 ) ) ;
#20604=CARTESIAN_POINT ( 'NONE',  ( 105.3430358795248338, -8.402594152722688392, -9.854619843455216355 ) ) ;
#20626=CARTESIAN_POINT ( 'NONE',  ( 114.3719421295247827, 0.8980012041604618078, -13.39321520033831447 ) ) ;
#20631=VERTEX_POINT ( 'NONE', #12574 ) ;
#20633=CARTESIAN_POINT ( 'NONE',  ( 115.9947331777918862, -0.01829820670803256055, -14.64321520033831447 ) ) ;
#20637=CARTESIAN_POINT ( 'NONE',  ( 64.98167240748409768, -37.86052959031123777, -4.893215200338314474 ) ) ;
#20642=LINE ( 'NONE', #6732, #25328 ) ;
#20643=CARTESIAN_POINT ( 'NONE',  ( 106.8710046295248759, -4.863998795839590272, -18.39754474579285315 ) ) ;
#20648=CARTESIAN_POINT ( 'NONE',  ( 112.2188952545247531, -9.868328341294098749, -15.46607636864997204 ) ) ;
#20654=CARTESIAN_POINT ( 'NONE',  ( 108.0517077545248696, -7.250697342233347165, -7.631215200338321125 ) ) ;
#20661=ORIENTED_EDGE ( 'NONE', *, *, #11734, .T. ) ;
#20672=CARTESIAN_POINT ( 'NONE',  ( 116.8361907699537880, -1.174466963688203913, -17.11742336975050804 ) ) ;
#20673=CARTESIAN_POINT ( 'NONE',  ( 112.9134265045247645, -7.250697342233347165, -19.15521520033831138 ) ) ;
#20676=CARTESIAN_POINT ( 'NONE',  ( 112.6609831777918913, -0.01829820670813664396, -14.64321520033831447 ) ) ;
#20677=DIRECTION ( 'NONE',  ( 0.000000000000000000, 0.3713878862591650232, -0.9284778069183718952 ) ) ;
#20682=EDGE_CURVE ( 'NONE', #23478, #20559, #35890, .T. ) ;
#20684=CARTESIAN_POINT ( 'NONE',  ( 115.5526452545247622, -9.868328341294098749, -15.46607636864997204 ) ) ;
#20693=CARTESIAN_POINT ( 'NONE',  ( 116.9417077545247992, -2.791137627527939813, -18.39754474579286025 ) ) ;
#20696=CARTESIAN_POINT ( 'NONE',  ( 111.5938171295247940, -10.62599879583958540, -13.39321520033831447 ) ) ;
#20698=CARTESIAN_POINT ( 'NONE',  ( 113.4690515045247992, -2.477300249445798297, -7.631215200338321125 ) ) ;
#20701=EDGE_CURVE ( 'NONE', #32144, #7030, #2408, .T. ) ;
#20704=CARTESIAN_POINT ( 'NONE',  ( 107.7044421295247929, -9.868328341294093420, -13.39321520033831447 ) ) ;
#20705=CARTESIAN_POINT ( 'NONE',  ( 109.2294433505451678, -0.4438500802042310012, -15.88352395893305413 ) ) ;
#20709=VERTEX_POINT ( 'NONE', #12121 ) ;
#20718=AXIS2_PLACEMENT_3D ( 'NONE', #6379, #41930, #41274 ) ;
#20719=CARTESIAN_POINT ( 'NONE',  ( 109.5102233795247884, -1.325403438956436419, -9.854619843455211026 ) ) ;
#20722=ORIENTED_EDGE ( 'NONE', *, *, #27452, .T. ) ;
#20727=CARTESIAN_POINT ( 'NONE',  ( 116.5944421295247793, 0.8980012041604618078, -13.39321520033831447 ) ) ;
#20729=DIRECTION ( 'NONE',  ( 1.000000000000000000, 0.000000000000000000, 0.000000000000000000 ) ) ;
#20736=PLANE ( 'NONE',  #8489 ) ;
#20745=CARTESIAN_POINT ( 'NONE',  ( 108.4684265045247997, -7.250697342233347165, -19.15521520033831138 ) ) ;
#20747=CARTESIAN_POINT ( 'NONE',  ( 87.44708369096655076, -21.99489077589587538, -8.186108419151770121 ) ) ;
#20749=CARTESIAN_POINT ( 'NONE',  ( 113.6792791257774979, 0.2334052082820642360, -12.14321520033833046 ) ) ;
#20757=CARTESIAN_POINT ( 'NONE',  ( 114.1635827545248389, -6.936859964151250502, -8.388885654883777576 ) ) ;
#20764=CARTESIAN_POINT ( 'NONE',  ( 83.02743615869442806, -30.94908174223593633, -21.89321520033831447 ) ) ;
#20778=CARTESIAN_POINT ( 'NONE',  ( 107.1488171295247867, -10.62599879583958540, -13.39321520033831447 ) ) ;
#20780=ORIENTED_EDGE ( 'NONE', *, *, #10299, .F. ) ;
#20793=LINE ( 'NONE', #13951, #5048 ) ;
#20795=EDGE_LOOP ( 'NONE', ( #33217, #39071, #17835, #23917, #26770, #2461, #20161, #27804, #15826, #7578 ) ) ;
#20798=CARTESIAN_POINT ( 'NONE',  ( 107.4960827545248350, -2.477300249445798297, -19.15521520033831138 ) ) ;
#20799=CARTESIAN_POINT ( 'NONE',  ( 109.9963952545248134, -9.868328341294098749, -15.46607636864997204 ) ) ;
#20800=CARTESIAN_POINT ( 'NONE',  ( 109.4407702545248355, -10.62599879583958717, -15.77991374673208469 ) ) ;
#20805=CARTESIAN_POINT ( 'NONE',  ( 113.2606921295247702, 0.8980012041604618078, -13.39321520033831447 ) ) ;
#20806=LINE ( 'NONE', #24666, #31417 ) ;
#20813=CARTESIAN_POINT ( 'NONE',  ( 106.3153796295248412, -4.863998795839590272, -19.15521520033831493 ) ) ;
#20815=CYLINDRICAL_SURFACE ( 'NONE', #13569, 4.500000000000003553 ) ;
#20818=CARTESIAN_POINT ( 'NONE',  ( 115.4137390045248566, 0.8980012041604421569, -15.77991374673208469 ) ) ;
#20819=CARTESIAN_POINT ( 'NONE',  ( 106.6626452545248611, -9.868328341294098749, -15.46607636864997204 ) ) ;
#20833=ADVANCED_FACE ( 'NONE', ( #33746 ), #3132, .F. ) ;
#20834=EDGE_CURVE ( 'NONE', #24866, #1124, #43351, .T. ) ;
#20840=CARTESIAN_POINT ( 'NONE',  ( 106.8015515045248378, -6.936859964151250502, -18.39754474579286025 ) ) ;
#20847=LINE ( 'NONE', #31318, #19336 ) ;
#20849=B_SPLINE_CURVE_WITH_KNOTS ( 'NONE', 3,
 ( #16210, #12490, #9743, #20001, #33885, #2201, #2655, #16587, #30481, #2888 ),
 .UNSPECIFIED., .F., .F.,
 ( 4, 3, 3, 4 ),
 ( 0.000000000000000000, 0.0002476486447138955493, 0.0004952972925464370650, 0.0009604418836934769301 ),
 .UNSPECIFIED. ) ;
#20850=CARTESIAN_POINT ( 'NONE',  ( 85.49677685831618135, -28.45307765865058514, -9.194547833600635656 ) ) ;
#20856=CARTESIAN_POINT ( 'NONE',  ( 109.4627908578216733, 0.04929351793716424401, -12.14321520033835533 ) ) ;
#20857=CARTESIAN_POINT ( 'NONE',  ( 115.0664733795247798, -8.938348069036489818, -17.46756447353520159 ) ) ;
#20861=CARTESIAN_POINT ( 'NONE',  ( 112.3578015045248719, -6.936859964151197211, -18.39754474579287447 ) ) ;
#20862=CARTESIAN_POINT ( 'NONE',  ( 109.2324108795247923, -1.325403438956436419, -16.93181055722141792 ) ) ;
#20865=CARTESIAN_POINT ( 'NONE',  ( 111.5938171295247940, -10.62599879583958540, -13.39321520033832158 ) ) ;
#20866=CARTESIAN_POINT ( 'NONE',  ( 109.2294413173287921, -4.065513199837466729, -18.48415429053572723 ) ) ;
#20868=CARTESIAN_POINT ( 'NONE',  ( 105.8986608795248401, -8.938348069036489818, -9.318865927141430916 ) ) ;
#20870=CARTESIAN_POINT ( 'NONE',  ( 110.6214733795247867, -8.938348069036489818, -17.46756447353520159 ) ) ;
#20873=CARTESIAN_POINT ( 'NONE',  ( 84.39081516114413262, -30.32262605124143562, -4.893215200338314474 ) ) ;
#20878=CIRCLE ( 'NONE', #28906, 5.132259260909266985 ) ;
#20884=VERTEX_POINT ( 'NONE', #6623 ) ;
#20889=CARTESIAN_POINT ( 'NONE',  ( 115.3442858795247759, -0.7896495226426338832, -17.46756447353520159 ) ) ;
#20890=VERTEX_POINT ( 'NONE', #27822 ) ;
#20897=CARTESIAN_POINT ( 'NONE',  ( 61.69189222814998175, -50.16718729050181480, -6.893215200338315363 ) ) ;
#20899=CARTESIAN_POINT ( 'NONE',  ( 68.68839935636916039, -25.95913848132418522, -5.893215200338315363 ) ) ;
#20902=CARTESIAN_POINT ( 'NONE',  ( 61.76986277844709861, -39.32091226840162079, -19.39321520033831447 ) ) ;
#20903=CARTESIAN_POINT ( 'NONE',  ( 115.2748327545248657, -6.936859964151250502, -8.388885654883777576 ) ) ;
#20911=CARTESIAN_POINT ( 'NONE',  ( 61.69189222814998175, -40.21211973637273474, -7.393215200338315363 ) ) ;
#20916=CYLINDRICAL_SURFACE ( 'NONE', #15471, 5.000000000000004441 ) ;
#20917=CARTESIAN_POINT ( 'NONE',  ( 114.4413952545248350, 0.8980012041604421569, -11.00651665394454071 ) ) ;
#20920=CARTESIAN_POINT ( 'NONE',  ( 109.2294426061139774, -0.2561256457631079786, -10.72386383753679340 ) ) ;
#20923=CARTESIAN_POINT ( 'NONE',  ( 107.2877233795247776, -1.325403438956436419, -9.854619843455211026 ) ) ;
#20927=CARTESIAN_POINT ( 'NONE',  ( 113.1217858795247935, -0.7896495226426338832, -17.46756447353520159 ) ) ;
#20928=LINE ( 'NONE', #7228, #15535 ) ;
#20939=CARTESIAN_POINT ( 'NONE',  ( 106.2459265045248173, -2.791137627527939813, -8.388885654883777576 ) ) ;
#20941=CARTESIAN_POINT ( 'NONE',  ( 85.31664890835789095, -21.99489077589589314, -15.39321520033831980 ) ) ;
#20942=ORIENTED_EDGE ( 'NONE', *, *, #17584, .F. ) ;
#20947=CARTESIAN_POINT ( 'NONE',  ( 116.4555358795247884, -0.7896495226426338832, -17.46756447353520159 ) ) ;
#20955=CYLINDRICAL_SURFACE ( 'NONE', #20718, 1.999999999999998668 ) ;
#20965=CARTESIAN_POINT ( 'NONE',  ( 108.7462390045248242, 0.8980012041604421569, -15.77991374673208469 ) ) ;
#20967=CARTESIAN_POINT ( 'NONE',  ( 114.7886608795247696, -1.325403438956436419, -16.93181055722138595 ) ) ;
#20970=ORIENTED_EDGE ( 'NONE', *, *, #28100, .F. ) ;
#20974=CARTESIAN_POINT ( 'NONE',  ( 109.3272331777918822, -0.01829820670803256055, -14.64321520033831447 ) ) ;
#20976=CARTESIAN_POINT ( 'NONE',  ( 113.0523327545247838, -6.936859964151250502, -8.388885654883777576 ) ) ;
#20978=EDGE_LOOP ( 'NONE', ( #43115, #43829, #1014, #16239 ) ) ;
#20991=ORIENTED_EDGE ( 'NONE', *, *, #10543, .T. ) ;
#20994=CARTESIAN_POINT ( 'NONE',  ( 106.1764733795248219, -8.938348069036489818, -17.46756447353520159 ) ) ;
#20996=ORIENTED_EDGE ( 'NONE', *, *, #7822, .F. ) ;
#20999=EDGE_CURVE ( 'NONE', #32579, #40888, #6816, .T. ) ;
#21013=ORIENTED_EDGE ( 'NONE', *, *, #21238, .T. ) ;
#21015=CARTESIAN_POINT ( 'NONE',  ( 113.3301452545248083, -9.868328341294098749, -15.46607636864997204 ) ) ;
#21016=CARTESIAN_POINT ( 'NONE',  ( 107.7738952545248310, -9.868328341294098749, -15.46607636864997204 ) ) ;
#21017=CARTESIAN_POINT ( 'NONE',  ( 107.7738952545248310, 0.8980012041604421569, -11.00651665394454071 ) ) ;
#21023=CARTESIAN_POINT ( 'NONE',  ( 113.4690515045247992, -2.477300249445798297, -7.631215200338321125 ) ) ;
#21029=CARTESIAN_POINT ( 'NONE',  ( 114.2330358795247776, -0.7896495226426338832, -17.46756447353520159 ) ) ;
#21030=CARTESIAN_POINT ( 'NONE',  ( 106.5237390045248418, 0.8980012041604421569, -15.77991374673208469 ) ) ;
#21035=B_SPLINE_CURVE_WITH_KNOTS ( 'NONE', 3,
 ( #11465, #4825, #32637, #22386, #1403, #36281, #38808, #5049, #15544, #39038 ),
 .UNSPECIFIED., .F., .F.,
 ( 4, 3, 3, 4 ),
 ( 0.000000000000000000, 0.0002476487219222790075, 0.0004952974148303609372, 0.0009534114850261630417 ),
 .UNSPECIFIED. ) ;
#21036=CARTESIAN_POINT ( 'NONE',  ( 114.3719421295247827, 0.8980012041604618078, -13.39321520033831447 ) ) ;
#21037=CARTESIAN_POINT ( 'NONE',  ( 106.1070202545248407, 0.1403307496149616695, -11.32035403202665336 ) ) ;
#21047=CARTESIAN_POINT ( 'NONE',  ( 111.2465515045248168, -6.936859964151250502, -18.39754474579286025 ) ) ;
#21048=EDGE_LOOP ( 'NONE', ( #2769, #32833, #41596, #41485 ) ) ;
#21055=CARTESIAN_POINT ( 'NONE',  ( 63.69189222814998175, -74.27079820037398861, -36.22049641875047143 ) ) ;
#21056=CARTESIAN_POINT ( 'NONE',  ( 116.3860827545247787, -2.477300249445798297, -19.15521520033831138 ) ) ;
#21061=ORIENTED_EDGE ( 'NONE', *, *, #14202, .F. ) ;
#21071=DIRECTION ( 'NONE',  ( -1.000000000000000000, 0.000000000000000000, 0.000000000000000000 ) ) ;
#21072=CARTESIAN_POINT ( 'NONE',  ( 110.3436608795247764, -8.938348069036489818, -9.318865927141430916 ) ) ;
#21077=CARTESIAN_POINT ( 'NONE',  ( 112.2883483795247770, -8.402594152722688392, -16.93181055722141792 ) ) ;
#21079=CARTESIAN_POINT ( 'NONE',  ( 109.2294421291290405, -4.119415819779401744, -18.49485328025912878 ) ) ;
#21081=CARTESIAN_POINT ( 'NONE',  ( 106.3848327545248651, -2.477300249445798297, -19.15521520033831138 ) ) ;
#21082=CARTESIAN_POINT ( 'NONE',  ( 116.9417077545247992, -2.791137627527939813, -18.39754474579286025 ) ) ;
#21083=CARTESIAN_POINT ( 'NONE',  ( 111.1076452545248259, 0.8980012041604421569, -11.00651665394454071 ) ) ;
#21089=VERTEX_POINT ( 'NONE', #8590 ) ;
#21099=CARTESIAN_POINT ( 'NONE',  ( 112.8439733795247832, -8.938348069036489818, -17.46756447353520159 ) ) ;
#21103=DIRECTION ( 'NONE',  ( 0.000000000000000000, -0.9284778069183718952, -0.3713878862591650232 ) ) ;
#21113=CARTESIAN_POINT ( 'NONE',  ( 115.2053796295247849, -4.863998795839590272, -8.388885654883775800 ) ) ;
#21117=PLANE ( 'NONE',  #41348 ) ;
#21125=CARTESIAN_POINT ( 'NONE',  ( 114.5108483795247878, -8.402594152722688392, -16.93181055722141792 ) ) ;
#21128=CARTESIAN_POINT ( 'NONE',  ( 85.03101011666282716, -29.58136537014402023, -10.62075117454815043 ) ) ;
#21129=CARTESIAN_POINT ( 'NONE',  ( 110.8298327545248299, -2.477300249445798297, -19.15521520033831138 ) ) ;
#21132=CARTESIAN_POINT ( 'NONE',  ( 74.69189222814998175, -41.76310523276723785, -4.893215200338314474 ) ) ;
#21134=CARTESIAN_POINT ( 'NONE',  ( 109.2294423051889112, -0.2441102078206954518, -10.74723311813985305 ) ) ;
#21136=CARTESIAN_POINT ( 'NONE',  ( 109.0240515045248202, -6.936859964151250502, -18.39754474579286025 ) ) ;
#21137=EDGE_CURVE ( 'NONE', #44361, #4412, #43474, .T. ) ;
#21138=CARTESIAN_POINT ( 'NONE',  ( 116.7096590385446433, 2.077600134054068626, -20.77163152589008632 ) ) ;
#21141=CARTESIAN_POINT ( 'NONE',  ( 110.4825671295247815, -10.62599879583958540, -13.39321520033831447 ) ) ;
#21145=ORIENTED_EDGE ( 'NONE', *, *, #24741, .F. ) ;
#21148=AXIS2_PLACEMENT_3D ( 'NONE', #3247, #17173, #31062 ) ;
#21154=CARTESIAN_POINT ( 'NONE',  ( 108.6767858795247861, -8.402594152722688392, -9.854619843455216355 ) ) ;
#21162=CARTESIAN_POINT ( 'NONE',  ( 116.1082702545247827, -10.62599879583958717, -15.77991374673208469 ) ) ;
#21164=VECTOR ( 'NONE', #37098, 1000.000000000000000 ) ;
#21168=CARTESIAN_POINT ( 'NONE',  ( 77.41180319171111535, -56.67956859520202073, -1.766371313089957651 ) ) ;
#21173=AXIS2_PLACEMENT_3D ( 'NONE', #19973, #6518, #3090 ) ;
#21183=CARTESIAN_POINT ( 'NONE',  ( 108.1211608795247798, -8.938348069036489818, -9.318865927141430916 ) ) ;
#21186=CYLINDRICAL_SURFACE ( 'NONE', #34934, 5.000000000000004441 ) ;
#21195=CARTESIAN_POINT ( 'NONE',  ( 110.4825671295247815, 0.1403307496149613920, -13.39321520033831447 ) ) ;
#21206=CYLINDRICAL_SURFACE ( 'NONE', #6293, 5.132259260909280307 ) ;
#21209=ORIENTED_EDGE ( 'NONE', *, *, #2177, .T. ) ;
#21210=CARTESIAN_POINT ( 'NONE',  ( 116.5944421295247793, -9.863109299026486809, -13.29890625629612622 ) ) ;
#21219=CARTESIAN_POINT ( 'NONE',  ( 105.8292077545248446, -7.250697342233347165, -7.631215200338321125 ) ) ;
#21224=CARTESIAN_POINT ( 'NONE',  ( 79.05243529145373316, 4.793396140045460108, -21.04957699274893557 ) ) ;
#21238=EDGE_CURVE ( 'NONE', #23757, #13343, #4706, .T. ) ;
#21239=CARTESIAN_POINT ( 'NONE',  ( 116.0850743346829859, -0.02132060320154255395, -12.14321520033831625 ) ) ;
#21240=CARTESIAN_POINT ( 'NONE',  ( 115.2053796295247849, -4.863998795839590272, -8.388885654883775800 ) ) ;
#21241=CARTESIAN_POINT ( 'NONE',  ( 110.8992858795247827, -8.402594152722688392, -9.854619843455216355 ) ) ;
#21242=CARTESIAN_POINT ( 'NONE',  ( 113.9552233795247815, -1.325403438956436419, -9.854619843455211026 ) ) ;
#21247=CARTESIAN_POINT ( 'NONE',  ( 113.3995983795247895, -0.7896495226426338832, -9.318865927141430916 ) ) ;
#21253=CARTESIAN_POINT ( 'NONE',  ( 114.5803015045248117, -2.477300249445798297, -7.631215200338321125 ) ) ;
#21254=CARTESIAN_POINT ( 'NONE',  ( 115.1359265045248605, -2.791137627527939813, -8.388885654883777576 ) ) ;
#21260=CARTESIAN_POINT ( 'NONE',  ( 114.1635827545248389, -2.477300249445798297, -19.15521520033831138 ) ) ;
#21261=CARTESIAN_POINT ( 'NONE',  ( 106.8710046295248759, -4.863998795839590272, -18.39754474579285315 ) ) ;
#21271=LINE ( 'NONE', #6529, #16167 ) ;
#21272=CARTESIAN_POINT ( 'NONE',  ( 110.6909265045248247, -2.791137627527939813, -8.388885654883777576 ) ) ;
#21278=VERTEX_POINT ( 'NONE', #29107 ) ;
#21280=CARTESIAN_POINT ( 'NONE',  ( 114.8581140045248361, -10.62599879583958717, -11.00651665394454604 ) ) ;
#21285=B_SPLINE_CURVE_WITH_KNOTS ( 'NONE', 3,
 ( #30934, #27521, #20231, #24102, #23884, #27068, #12942, #30708, #26840, #34118, #40752, #34339, #13165, #37768, #9509, #23425, #13395, #37311, #44857, #6078, #44631, #6541, #41437, #26612, #27298, #33884, #2654, #37995, #16586, #41212, #9973, #38875, #11078, #24981, #39110 ),
 .UNSPECIFIED., .F., .F.,
 ( 4, 2, 2, 1, 1, 1, 2, 2, 2, 2, 1, 1, 2, 2, 2, 2, 1, 1, 2, 2, 4 ),
 ( 0.000000000000000000, 0.1249999999996228572, 0.1874999999994343414, 0.2187499999993456345, 0.2343749999992951194, 0.2421874999992763844, 0.2460937499992742750, 0.2499999999992721378, 0.3749999999993665067, 0.4374999999994138022, 0.4687499999994378941, 0.4843749999994453881, 0.4921874999994536592, 0.4999999999994618749, 0.6249999999996362909, 0.6874999999997234434, 0.7187499999997635225, 0.7343749999997836175, 0.7421874999997902789, 0.7499999999997970512, 1.000000000000000000 ),
 .UNSPECIFIED. ) ;
#21291=CARTESIAN_POINT ( 'NONE',  ( 84.51109360120207725, -29.99489077589584696, -11.85273644461004672 ) ) ;
#21292=CARTESIAN_POINT ( 'NONE',  ( 115.6915515045247531, -2.477300249445798297, -7.631215200338321125 ) ) ;
#21298=CARTESIAN_POINT ( 'NONE',  ( 110.7603796295247918, -4.863998795839590272, -19.15521520033831493 ) ) ;
#21301=( GEOMETRIC_REPRESENTATION_CONTEXT ( 3 ) GLOBAL_UNCERTAINTY_ASSIGNED_CONTEXT ( ( #35598 ) ) GLOBAL_UNIT_ASSIGNED_CONTEXT ( ( #33697, #10012, #37802 ) ) REPRESENTATION_CONTEXT ( 'NONE', 'WORKASPACE' ) );
#21304=CARTESIAN_POINT ( 'NONE',  ( 111.5243640045248412, 0.1403307496149616695, -15.46607636864997204 ) ) ;
#21307=CARTESIAN_POINT ( 'NONE',  ( 109.2294940316331662, -8.917758382726240995, -16.95199246166307461 ) ) ;
#21311=CARTESIAN_POINT ( 'NONE',  ( 115.7610046295247912, -4.863998795839590272, -18.39754474579285315 ) ) ;
#21312=CARTESIAN_POINT ( 'NONE',  ( 111.5243640045248412, -10.62599879583958717, -11.00651665394454604 ) ) ;
#21325=B_SPLINE_CURVE_WITH_KNOTS ( 'NONE', 3,
 ( #5233, #32812, #5452, #43096, #32594, #11865, #8888, #22346, #36240, #33480 ),
 .UNSPECIFIED., .F., .F.,
 ( 4, 3, 3, 4 ),
 ( 0.000000000000000000, 0.0002476486447138720221, 0.0004952972925464129957, 0.0009604418836934600166 ),
 .UNSPECIFIED. ) ;
#21329=CARTESIAN_POINT ( 'NONE',  ( 110.0658483795247804, -0.7896495226426338832, -9.318865927141430916 ) ) ;
#21332=CARTESIAN_POINT ( 'NONE',  ( 116.6638952545248031, -9.868328341294098749, -15.46607636864997204 ) ) ;
#21339=CARTESIAN_POINT ( 'NONE',  ( 116.6638952545248031, -9.868328341294098749, -15.46607636864997204 ) ) ;
#21341=( LENGTH_UNIT ( ) NAMED_UNIT ( * ) SI_UNIT ( .MILLI., .METRE. ) );
#21342=DIRECTION ( 'NONE',  ( 1.000000000000000000, 0.000000000000000000, 0.000000000000000000 ) ) ;
#21350=CARTESIAN_POINT ( 'NONE',  ( 113.8857702545248003, 0.1403307496149616695, -11.32035403202665336 ) ) ;
#21353=CARTESIAN_POINT ( 'NONE',  ( 86.44458416315558225, -26.15744216582745452, -8.393215200338314474 ) ) ;
#21354=CARTESIAN_POINT ( 'NONE',  ( 112.6356140045247827, -10.62599879583958717, -11.00651665394454604 ) ) ;
#21359=CARTESIAN_POINT ( 'NONE',  ( 109.2294668341613288, -0.5633236648423508575, -10.20431573512175483 ) ) ;
#21361=CARTESIAN_POINT ( 'NONE',  ( 108.8851452545248151, -9.868328341294098749, -15.46607636864997204 ) ) ;
#21362=CARTESIAN_POINT ( 'NONE',  ( 117.2190380802938137, 1.225124243697611526, -21.63543231393177280 ) ) ;
#21365=CARTESIAN_POINT ( 'NONE',  ( 109.0935046295247872, -4.863998795839590272, -7.631215200338315796 ) ) ;
#21367=ORIENTED_EDGE ( 'NONE', *, *, #13999, .T. ) ;
#21376=CARTESIAN_POINT ( 'NONE',  ( 115.1359265045248605, -7.250697342233347165, -19.15521520033831138 ) ) ;
#21385=CARTESIAN_POINT ( 'NONE',  ( 115.3442858795247759, -0.7896495226426338832, -17.46756447353520159 ) ) ;
#21386=AXIS2_PLACEMENT_3D ( 'NONE', #22148, #35589, #18508 ) ;
#21390=ADVANCED_FACE ( 'NONE', ( #16793 ), #26366, .F. ) ;
#21397=AXIS2_PLACEMENT_3D ( 'NONE', #12435, #43659, #1476 ) ;
#21403=CARTESIAN_POINT ( 'NONE',  ( 78.69189222814998175, -82.08636712479707853, -32.64558696907351987 ) ) ;
#21407=CARTESIAN_POINT ( 'NONE',  ( 112.1494421295248003, -9.868328341294093420, -13.39321520033831447 ) ) ;
#21413=CARTESIAN_POINT ( 'NONE',  ( 87.44708369096657918, -21.99489077589588604, -7.893215200338315363 ) ) ;
#21417=CARTESIAN_POINT ( 'NONE',  ( 112.9134265045247645, -2.791137627527939813, -8.388885654883777576 ) ) ;
#21424=DIRECTION ( 'NONE',  ( 0.000000000000000000, 0.000000000000000000, -1.000000000000000000 ) ) ;
#21432=ORIENTED_EDGE ( 'NONE', *, *, #41306, .T. ) ;
#21435=CARTESIAN_POINT ( 'NONE',  ( 116.2471765045247594, -2.791137627527939813, -8.388885654883777576 ) ) ;
#21438=EDGE_LOOP ( 'NONE', ( #14422, #11185, #40731, #33356 ) ) ;
#21439=CARTESIAN_POINT ( 'NONE',  ( 76.69189222814998175, -50.16718729050181480, 3.106784799661685526 ) ) ;
#21441=CARTESIAN_POINT ( 'NONE',  ( 106.8015515045248378, -2.477300249445798297, -7.631215200338321125 ) ) ;
#21452=CARTESIAN_POINT ( 'NONE',  ( 69.69189222814998175, -41.76310523276723785, -20.39321520033831447 ) ) ;
#21453=FACE_OUTER_BOUND ( 'NONE', #43644, .T. ) ;
#21458=CARTESIAN_POINT ( 'NONE',  ( 68.68839935636916039, -25.95913848132418522, -5.893215200338315363 ) ) ;
#21462=CARTESIAN_POINT ( 'NONE',  ( 113.2226630180080775, 0.7607806665038616689, -14.64321520033831447 ) ) ;
#21464=CARTESIAN_POINT ( 'NONE',  ( 112.4967077545247633, -2.791137627527939813, -18.39754474579286025 ) ) ;
#21465=CARTESIAN_POINT ( 'NONE',  ( 107.4960827545248350, -6.936859964151250502, -8.388885654883777576 ) ) ;
#21466=CARTESIAN_POINT ( 'NONE',  ( 114.5108483795247878, -8.402594152722688392, -16.93181055722141792 ) ) ;
#21469=VERTEX_POINT ( 'NONE', #18242 ) ;
#21471=CARTESIAN_POINT ( 'NONE',  ( 110.4825671295247815, -10.62599879583958540, -13.39321520033831447 ) ) ;
#21475=FACE_OUTER_BOUND ( 'NONE', #31141, .T. ) ;
#21477=CARTESIAN_POINT ( 'NONE',  ( 114.6497546295247929, -4.863998795839590272, -7.631215200338315796 ) ) ;
#21478=CARTESIAN_POINT ( 'NONE',  ( 113.1217858795247935, -8.402594152722688392, -9.854619843455216355 ) ) ;
#21495=CARTESIAN_POINT ( 'NONE',  ( 106.3848327545248651, -2.477300249445798297, -19.15521520033831138 ) ) ;
#21496=CARTESIAN_POINT ( 'NONE',  ( 111.5243640045248412, 0.1403307496149616695, -15.46607636864997204 ) ) ;
#21498=ORIENTED_EDGE ( 'NONE', *, *, #43714, .F. ) ;
#21501=( BOUNDED_SURFACE ( )  B_SPLINE_SURFACE ( 1, 2, ( 
 ( #33878, #12705, #37305, #8601, #43488, #6071, #22722, #5166, #19083, #8821, #32969, #41651, #10409, #24094, #38420, #38202, #41431, #41205, #20889, #45063, #34549, #9966, #3546, #27513, #6981, #44851, #24318, #132, #31359, #13822, #13604, #34333, #3107, #30924, #14044, #27737, #34110, #37533, #37988, #10188, #6764, #17461, #23877, #6306, #34767, #13388, #30474, #3331, #44394, #44622, #27962, #41869, #20224, #20673, #21099, #7191, #17252, #37763, #31140, #10629, #2880, #24533, #30702, #34977, #16579, #13158, #27060, #9736, #16809, #40980, #23646, #27292, #6532, #20450, #17034, #794, #7873, #3987, #21553, #11296, #32028, #35441, #11526, #7409, #35894, #1023, #21781, #18583, #24975, #38635, #14716, #38870, #32255, #10850, #21329, #35215, #17910, #11071, #35672, #28851, #42763, #17687, #28627, #25432, #31807, #39333, #7639, #28399, #8100, #4217, #24748, #42536, #25206, #31585, #18363, #18133, #39103, #4445, #22001, #4663, #579, #14488, #42090, #14940, #3764, #353, #14266, #28183, #42311, #6462, #44994, #34691, #3033, #37689, #34472, #3251, #41575, #10335, #34258, #17395, #56, #13970, #34903, #24672, #38131, #21030, #3479, #41796, #20813, #30848, #27882, #27662, #10554, #13753, #17833, #7120, #28107, #44541, #42011, #41360, #13304 ),
 ( #31283, #6686, #9889, #44771, #7335, #37908, #27211, #41129, #16954, #24238, #24452, #38343, #6902, #21254, #3692, #17614, #24020, #31506, #278, #14188, #20597, #10776, #38559, #35133, #3914, #23799, #20371, #13531, #27438, #10117, #17177, #31066, #948, #15307, #28998, #4138, #7564, #8016, #25357, #21923, #32626, #11224, #21478, #8244, #28554, #500, #4588, #14412, #14636, #29215, #1392, #35363, #11451, #36269, #22373, #5037, #39480, #43125, #31730, #11894, #42459, #28322, #11668, #35816, #42234, #24899, #10998, #38792, #18059, #31950, #14866, #25796, #18511, #32401, #22151, #39705, #28775, #36043, #32178, #8470, #4362, #35592, #25130, #4812, #1172, #42906, #715, #15087, #25576, #39025, #18733, #7796, #21705, #18282, #42683, #39251, #6081, #9290, #5851, #2656, #17042, #30710, #19773, #23198, #9744, #27070, #23656, #34341, #12944, #37077, #9975, #30257, #2202, #6314, #16130, #16355, #30936, #3117, #33655, #13167, #37997, #24104, #16589, #9511, #20233, #44859, #2431, #44403, #44183, #13614, #16818, #27523, #41439, #26614, #26842, #40992, #40528, #40754, #10197, #23428, #37313, #37542, #44633, #20002, #30482, #34120, #2889, #13398, #6772, #33886, #33424, #6543, #27300, #30033, #41215, #23886, #37770, #20459, #43947, #12714, #38430 ) ),
 .UNSPECIFIED., .F., .F., .F. ) 
 B_SPLINE_SURFACE_WITH_KNOTS ( ( 2, 2 ),
 ( 3, 2, 2, 2, 2, 2, 2, 2, 2, 2, 2, 2, 2, 2, 2, 2, 2, 2, 2, 2, 2, 2, 2, 2, 2, 2, 2, 2, 2, 2, 2, 2, 2, 2, 2, 2, 2, 2, 2, 2, 2, 2, 2, 2, 2, 2, 2, 2, 2, 2, 2, 2, 2, 2, 2, 2, 2, 2, 2, 2, 2, 2, 2, 2, 2, 2, 2, 2, 2, 2, 2, 2, 2, 2, 2, 2, 2, 2, 2, 2, 3 ),
 ( 0.000000000000000000, 1.000000000000000000 ),
 ( 0.000000000000000000, 0.01250000000000000069, 0.02500000000000000139, 0.03749999999999999861, 0.05000000000000000278, 0.06250000000000000000, 0.07499999999999999722, 0.08749999999999999445, 0.1000000000000000056, 0.1125000000000000028, 0.1250000000000000000, 0.1375000000000000111, 0.1499999999999999944, 0.1625000000000000056, 0.1749999999999999889, 0.1875000000000000000, 0.2000000000000000111, 0.2124999999999999944, 0.2250000000000000056, 0.2374999999999999889, 0.2500000000000000000, 0.2625000000000000111, 0.2750000000000000222, 0.2874999999999999778, 0.2999999999999999889, 0.3125000000000000000, 0.3250000000000000111, 0.3375000000000000222, 0.3499999999999999778, 0.3624999999999999889, 0.3750000000000000000, 0.3875000000000000111, 0.4000000000000000222, 0.4124999999999999778, 0.4249999999999999889, 0.4375000000000000000, 0.4500000000000000111, 0.4625000000000000222, 0.4749999999999999778, 0.4874999999999999889, 0.5000000000000000000, 0.5124999999999999556, 0.5250000000000000222, 0.5374999999999999778, 0.5500000000000000444, 0.5625000000000000000, 0.5749999999999999556, 0.5875000000000000222, 0.5999999999999999778, 0.6125000000000000444, 0.6250000000000000000, 0.6374999999999999556, 0.6500000000000000222, 0.6624999999999999778, 0.6750000000000000444, 0.6875000000000000000, 0.6999999999999999556, 0.7125000000000000222, 0.7249999999999999778, 0.7375000000000000444, 0.7500000000000000000, 0.7624999999999999556, 0.7750000000000000222, 0.7874999999999999778, 0.8000000000000000444, 0.8125000000000000000, 0.8249999999999999556, 0.8375000000000000222, 0.8499999999999999778, 0.8625000000000000444, 0.8750000000000000000, 0.8874999999999999556, 0.9000000000000000222, 0.9124999999999999778, 0.9250000000000000444, 0.9375000000000000000, 0.9499999999999999556, 0.9625000000000000222, 0.9749999999999999778, 0.9875000000000000444, 1.000000000000000000 ),
 .UNSPECIFIED. ) 
 GEOMETRIC_REPRESENTATION_ITEM ( )  RATIONAL_B_SPLINE_SURFACE ( (
 ( 1.000000000000000000, 0.9238795325112869605, 1.000000000000000000, 0.9238795325112869605, 1.000000000000000000, 0.9238795325112869605, 1.000000000000000000, 0.9238795325112869605, 1.000000000000000000, 0.9238795325112869605, 1.000000000000000000, 0.9238795325112869605, 1.000000000000000000, 0.9238795325112869605, 1.000000000000000000, 0.9238795325112869605, 1.000000000000000000, 0.9238795325112869605, 1.000000000000000000, 0.9238795325112869605, 1.000000000000000000, 0.9238795325112869605, 1.000000000000000000, 0.9238795325112869605, 1.000000000000000000, 0.9238795325112869605, 1.000000000000000000, 0.9238795325112869605, 1.000000000000000000, 0.9238795325112869605, 1.000000000000000000, 0.9238795325112869605, 1.000000000000000000, 0.9238795325112869605, 1.000000000000000000, 0.9238795325112869605, 1.000000000000000000, 0.9238795325112869605, 1.000000000000000000, 0.9238795325112869605, 1.000000000000000000, 0.9238795325112869605, 1.000000000000000000, 0.9238795325112869605, 1.000000000000000000, 0.9238795325112869605, 1.000000000000000000, 0.9238795325112869605, 1.000000000000000000, 0.9238795325112869605, 1.000000000000000000, 0.9238795325112869605, 1.000000000000000000, 0.9238795325112869605, 1.000000000000000000, 0.9238795325112869605, 1.000000000000000000, 0.9238795325112869605, 1.000000000000000000, 0.9238795325112869605, 1.000000000000000000, 0.9238795325112869605, 1.000000000000000000, 0.9238795325112869605, 1.000000000000000000, 0.9238795325112869605, 1.000000000000000000, 0.9238795325112869605, 1.000000000000000000, 0.9238795325112869605, 1.000000000000000000, 0.9238795325112869605, 1.000000000000000000, 0.9238795325112869605, 1.000000000000000000, 0.9238795325112869605, 1.000000000000000000, 0.9238795325112869605, 1.000000000000000000, 0.9238795325112869605, 1.000000000000000000, 0.9238795325112869605, 1.000000000000000000, 0.9238795325112869605, 1.000000000000000000, 0.9238795325112869605, 1.000000000000000000, 0.9238795325112869605, 1.000000000000000000, 0.9238795325112869605, 1.000000000000000000, 0.9238795325112869605, 1.000000000000000000, 0.9238795325112869605, 1.000000000000000000, 0.9238795325112869605, 1.000000000000000000, 0.9238795325112869605, 1.000000000000000000, 0.9238795325112869605, 1.000000000000000000, 0.9238795325112869605, 1.000000000000000000, 0.9238795325112869605, 1.000000000000000000, 0.9238795325112869605, 1.000000000000000000, 0.9238795325112869605, 1.000000000000000000, 0.9238795325112869605, 1.000000000000000000, 0.9238795325112869605, 1.000000000000000000, 0.9238795325112869605, 1.000000000000000000, 0.9238795325112869605, 1.000000000000000000, 0.9238795325112869605, 1.000000000000000000, 0.9238795325112869605, 1.000000000000000000, 0.9238795325112869605, 1.000000000000000000, 0.9238795325112869605, 1.000000000000000000, 0.9238795325112869605, 1.000000000000000000, 0.9238795325112869605, 1.000000000000000000, 0.9238795325112869605, 1.000000000000000000, 0.9238795325112869605, 1.000000000000000000, 0.9238795325112869605, 1.000000000000000000, 0.9238795325112869605, 1.000000000000000000, 0.9238795325112869605, 1.000000000000000000, 0.9238795325112869605, 1.000000000000000000, 0.9238795325112869605, 1.000000000000000000, 0.9238795325112869605, 1.000000000000000000, 0.9238795325112869605, 1.000000000000000000, 0.9238795325112869605, 1.000000000000000000, 0.9238795325112869605, 1.000000000000000000, 0.9238795325112869605, 1.000000000000000000, 0.9238795325112869605, 1.000000000000000000, 0.9238795325112869605, 1.000000000000000000, 0.9238795325112869605, 1.000000000000000000, 0.9238795325112869605, 1.000000000000000000),
 ( 1.000000000000000000, 0.9238795325112869605, 1.000000000000000000, 0.9238795325112869605, 1.000000000000000000, 0.9238795325112869605, 1.000000000000000000, 0.9238795325112869605, 1.000000000000000000, 0.9238795325112869605, 1.000000000000000000, 0.9238795325112869605, 1.000000000000000000, 0.9238795325112869605, 1.000000000000000000, 0.9238795325112869605, 1.000000000000000000, 0.9238795325112869605, 1.000000000000000000, 0.9238795325112869605, 1.000000000000000000, 0.9238795325112869605, 1.000000000000000000, 0.9238795325112869605, 1.000000000000000000, 0.9238795325112869605, 1.000000000000000000, 0.9238795325112869605, 1.000000000000000000, 0.9238795325112869605, 1.000000000000000000, 0.9238795325112869605, 1.000000000000000000, 0.9238795325112869605, 1.000000000000000000, 0.9238795325112869605, 1.000000000000000000, 0.9238795325112869605, 1.000000000000000000, 0.9238795325112869605, 1.000000000000000000, 0.9238795325112869605, 1.000000000000000000, 0.9238795325112869605, 1.000000000000000000, 0.9238795325112869605, 1.000000000000000000, 0.9238795325112869605, 1.000000000000000000, 0.9238795325112869605, 1.000000000000000000, 0.9238795325112869605, 1.000000000000000000, 0.9238795325112869605, 1.000000000000000000, 0.9238795325112869605, 1.000000000000000000, 0.9238795325112869605, 1.000000000000000000, 0.9238795325112869605, 1.000000000000000000, 0.9238795325112869605, 1.000000000000000000, 0.9238795325112869605, 1.000000000000000000, 0.9238795325112869605, 1.000000000000000000, 0.9238795325112869605, 1.000000000000000000, 0.9238795325112869605, 1.000000000000000000, 0.9238795325112869605, 1.000000000000000000, 0.9238795325112869605, 1.000000000000000000, 0.9238795325112869605, 1.000000000000000000, 0.9238795325112869605, 1.000000000000000000, 0.9238795325112869605, 1.000000000000000000, 0.9238795325112869605, 1.000000000000000000, 0.9238795325112869605, 1.000000000000000000, 0.9238795325112869605, 1.000000000000000000, 0.9238795325112869605, 1.000000000000000000, 0.9238795325112869605, 1.000000000000000000, 0.9238795325112869605, 1.000000000000000000, 0.9238795325112869605, 1.000000000000000000, 0.9238795325112869605, 1.000000000000000000, 0.9238795325112869605, 1.000000000000000000, 0.9238795325112869605, 1.000000000000000000, 0.9238795325112869605, 1.000000000000000000, 0.9238795325112869605, 1.000000000000000000, 0.9238795325112869605, 1.000000000000000000, 0.9238795325112869605, 1.000000000000000000, 0.9238795325112869605, 1.000000000000000000, 0.9238795325112869605, 1.000000000000000000, 0.9238795325112869605, 1.000000000000000000, 0.9238795325112869605, 1.000000000000000000, 0.9238795325112869605, 1.000000000000000000, 0.9238795325112869605, 1.000000000000000000, 0.9238795325112869605, 1.000000000000000000, 0.9238795325112869605, 1.000000000000000000, 0.9238795325112869605, 1.000000000000000000, 0.9238795325112869605, 1.000000000000000000, 0.9238795325112869605, 1.000000000000000000, 0.9238795325112869605, 1.000000000000000000, 0.9238795325112869605, 1.000000000000000000, 0.9238795325112869605, 1.000000000000000000, 0.9238795325112869605, 1.000000000000000000, 0.9238795325112869605, 1.000000000000000000, 0.9238795325112869605, 1.000000000000000000, 0.9238795325112869605, 1.000000000000000000, 0.9238795325112869605, 1.000000000000000000, 0.9238795325112869605, 1.000000000000000000, 0.9238795325112869605, 1.000000000000000000, 0.9238795325112869605, 1.000000000000000000, 0.9238795325112869605, 1.000000000000000000, 0.9238795325112869605, 1.000000000000000000, 0.9238795325112869605, 1.000000000000000000, 0.9238795325112869605, 1.000000000000000000) ) ) 
 REPRESENTATION_ITEM ( '' )  SURFACE ( )  );
#21504=EDGE_LOOP ( 'NONE', ( #34870, #36556, #5537, #22541, #1196, #44251 ) ) ;
#21508=CARTESIAN_POINT ( 'NONE',  ( 112.2188952545247531, 0.8980012041604421569, -11.00651665394454071 ) ) ;
#21516=CYLINDRICAL_SURFACE ( 'NONE', #18981, 6.000000000000003553 ) ;
#21517=CARTESIAN_POINT ( 'NONE',  ( 85.21058564945587932, -28.08891145889253593, -8.461176451080145711 ) ) ;
#21518=CARTESIAN_POINT ( 'NONE',  ( 115.1359265045248605, -7.250697342233347165, -19.15521520033831138 ) ) ;
#21523=CARTESIAN_POINT ( 'NONE',  ( 112.4272546295247821, -4.863998795839590272, -7.631215200338315796 ) ) ;
#21528=CARTESIAN_POINT ( 'NONE',  ( 110.0658483795247804, -8.402594152722688392, -16.93181055722141792 ) ) ;
#21531=CARTESIAN_POINT ( 'NONE',  ( 109.2295669185610194, -6.591008720997902692, -18.37361123771471227 ) ) ;
#21535=CARTESIAN_POINT ( 'NONE',  ( 116.8722546295247895, -4.863998795839590272, -18.39754474579285315 ) ) ;
#21536=CARTESIAN_POINT ( 'NONE',  ( 107.3571765045248299, -7.250697342233347165, -19.15521520033831138 ) ) ;
#21553=CARTESIAN_POINT ( 'NONE',  ( 111.1770983795247787, -0.7896495226426338832, -9.318865927141430916 ) ) ;
#21556=CARTESIAN_POINT ( 'NONE',  ( 113.6079577545248043, -2.791137627527939813, -18.39754474579286025 ) ) ;
#21564=CARTESIAN_POINT ( 'NONE',  ( 116.7333483795247844, -8.402594152722688392, -16.93181055722141792 ) ) ;
#21576=CARTESIAN_POINT ( 'NONE',  ( 112.7050671295247923, 0.1403307496149613920, -13.39321520033831447 ) ) ;
#21581=CARTESIAN_POINT ( 'NONE',  ( 113.1912390045248031, 0.8980012041604421569, -15.77991374673208469 ) ) ;
#21585=CARTESIAN_POINT ( 'NONE',  ( 109.2295156139914383, -1.481211192124197051, -9.165827887151388964 ) ) ;
#21587=CARTESIAN_POINT ( 'NONE',  ( 114.0941296295247867, -4.863998795839590272, -19.15521520033831493 ) ) ;
#21589=CYLINDRICAL_SURFACE ( 'NONE', #16041, 2.000000000000001776 ) ;
#21592=CARTESIAN_POINT ( 'NONE',  ( 111.1076452545248259, 0.8980012041604421569, -11.00651665394454071 ) ) ;
#21603=CARTESIAN_POINT ( 'NONE',  ( 114.7886608795247696, -8.938348069036489818, -9.318865927141430916 ) ) ;
#21609=VECTOR ( 'NONE', #44234, 1000.000000000000000 ) ;
#21613=CARTESIAN_POINT ( 'NONE',  ( 106.6626452545248611, -9.868328341294098749, -15.46607636864997204 ) ) ;
#21616=CARTESIAN_POINT ( 'NONE',  ( 66.21962885992722647, -37.11159810974177731, -4.893215200338314474 ) ) ;
#21617=CARTESIAN_POINT ( 'NONE',  ( 64.85649322025210495, -35.54674243456235416, -5.785566283887345840 ) ) ;
#21631=CARTESIAN_POINT ( 'NONE',  ( 111.8021765045248372, -2.791137627527939813, -8.388885654883777576 ) ) ;
#21634=CARTESIAN_POINT ( 'NONE',  ( 114.3024890045248156, -9.868328341294150263, -11.32035403202669777 ) ) ;
#21642=CARTESIAN_POINT ( 'NONE',  ( 110.3436608795247764, -1.325403438956436419, -16.93181055722141792 ) ) ;
#21643=VERTEX_POINT ( 'NONE', #33932 ) ;
#21649=DIRECTION ( 'NONE',  ( 0.000000000000000000, 0.000000000000000000, 1.000000000000000000 ) ) ;
#21652=CARTESIAN_POINT ( 'NONE',  ( 78.69189222814998175, -50.16718729050182191, -6.893215200338315363 ) ) ;
#21653=CARTESIAN_POINT ( 'NONE',  ( 110.1099666496844804, 0.5600166689815611054, -12.14321520033828428 ) ) ;
#21658=CARTESIAN_POINT ( 'NONE',  ( 114.1635827545248389, -6.936859964151250502, -8.388885654883777576 ) ) ;
#21686=ORIENTED_EDGE ( 'NONE', *, *, #5520, .F. ) ;
#21689=CARTESIAN_POINT ( 'NONE',  ( 115.1359265045248605, -7.250697342233347165, -19.15521520033831138 ) ) ;
#21690=CARTESIAN_POINT ( 'NONE',  ( 105.8986608795248401, -8.938348069036489818, -9.318865927141430916 ) ) ;
#21691=CARTESIAN_POINT ( 'NONE',  ( 114.1635827545248389, -6.936859964151250502, -8.388885654883777576 ) ) ;
#21697=CARTESIAN_POINT ( 'NONE',  ( 106.1070202545248407, -10.62599879583958717, -15.77991374673208469 ) ) ;
#21699=CARTESIAN_POINT ( 'NONE',  ( 90.93679655599923706, -18.80572346544368756, -6.893215200338315363 ) ) ;
#21700=CARTESIAN_POINT ( 'NONE',  ( 109.2294759059926008, -0.3400322672942256985, -15.71119955778137545 ) ) ;
#21704=CARTESIAN_POINT ( 'NONE',  ( 112.9828796295247884, -4.863998795839590272, -19.15521520033831493 ) ) ;
#21705=CARTESIAN_POINT ( 'NONE',  ( 109.6491296295247793, -4.863998795839590272, -8.388885654883775800 ) ) ;
#21710=DIRECTION ( 'NONE',  ( 0.000000000000000000, 0.3713878862591638574, -0.9284778069183724503 ) ) ;
#21711=EDGE_CURVE ( 'NONE', #5648, #15833, #34474, .T. ) ;
#21720=EDGE_LOOP ( 'NONE', ( #45018, #16611 ) ) ;
#21723=CARTESIAN_POINT ( 'NONE',  ( 114.9275671295247889, -10.62599879583958540, -13.39321520033831447 ) ) ;
#21724=LINE ( 'NONE', #35611, #38985 ) ;
#21725=ORIENTED_EDGE ( 'NONE', *, *, #10952, .F. ) ;
#21733=DIRECTION ( 'NONE',  ( -0.9659258262890687563, -0.2588190451025194627, 0.000000000000000000 ) ) ;
#21735=CARTESIAN_POINT ( 'NONE',  ( 108.9545983795247821, -0.7896495226426338832, -9.318865927141430916 ) ) ;
#21740=VERTEX_POINT ( 'NONE', #26205 ) ;
#21742=DIRECTION ( 'NONE',  ( 0.000000000000000000, -0.8069730661766900681, 0.5905882410490337353 ) ) ;
#21743=CARTESIAN_POINT ( 'NONE',  ( 84.55230152525003007, -29.88260722510756651, -11.30949563633199162 ) ) ;
#21744=CARTESIAN_POINT ( 'NONE',  ( 115.4137390045248566, 0.8980012041604421569, -15.77991374673208469 ) ) ;
#21748=LINE ( 'NONE', #28366, #658 ) ;
#21749=CARTESIAN_POINT ( 'NONE',  ( 113.9552233795247815, -8.938348069036489818, -17.46756447353520159 ) ) ;
#21754=CARTESIAN_POINT ( 'NONE',  ( 106.9404577545248145, -2.791137627527939813, -18.39754474579286025 ) ) ;
#21756=VERTEX_POINT ( 'NONE', #9556 ) ;
#21758=CARTESIAN_POINT ( 'NONE',  ( 109.2295854867894320, -5.018741757313862628, -18.58799787790541558 ) ) ;
#21762=CARTESIAN_POINT ( 'NONE',  ( 114.3719421295247827, -9.868328341294093420, -13.39321520033831447 ) ) ;
#21776=ADVANCED_FACE ( 'NONE', ( #24583, #27566 ), #6584, .T. ) ;
#21778=( BOUNDED_CURVE ( )  B_SPLINE_CURVE ( 2, ( #13200, #27330, #40785, #9543, #27100, #10006, #9776, #23915, #23690, #20490, #34369, #17072, #27774, #34588, #3372, #17291, #31184 ),
 .UNSPECIFIED., .F., .F. ) 
 B_SPLINE_CURVE_WITH_KNOTS ( ( 3, 2, 2, 2, 2, 2, 2, 2, 3 ),
 ( 0.2035091206787220108, 0.2124999999999999944, 0.2250000000000000056, 0.2374999999999999889, 0.2500000000000000000, 0.2625000000000000111, 0.2750000000000000222, 0.2874999999999999778, 0.2964908793212779892 ),
 .UNSPECIFIED. ) 
 CURVE ( )  GEOMETRIC_REPRESENTATION_ITEM ( )  RATIONAL_B_SPLINE_CURVE ( ( 0.9692594319298230010, 0.9452488050343769155, 1.000000000000000000, 0.9238795325112869605, 1.000000000000000000, 0.9238795325112869605, 1.000000000000000000, 0.9238795325112869605, 1.000000000000000000, 0.9238795325112869605, 1.000000000000000000, 0.9238795325112869605, 1.000000000000000000, 0.9238795325112869605, 1.000000000000000000, 0.9452488050343769155, 0.9692594319298220018 ) ) 
 REPRESENTATION_ITEM ( '' )  );
#21781=CARTESIAN_POINT ( 'NONE',  ( 110.6214733795247867, -8.938348069036489818, -17.46756447353520159 ) ) ;
#21784=CARTESIAN_POINT ( 'NONE',  ( 114.3719421295247827, -9.868328341294093420, -13.39321520033831447 ) ) ;
#21790=CARTESIAN_POINT ( 'NONE',  ( 110.2047546295247855, -4.863998795839590272, -18.39754474579285315 ) ) ;
#21799=CARTESIAN_POINT ( 'NONE',  ( 113.3301452545248083, -9.868328341294098749, -15.46607636864997204 ) ) ;
#21803=CARTESIAN_POINT ( 'NONE',  ( 85.34650993476388692, -28.81703154067693617, -9.558501715626988471 ) ) ;
#21804=CARTESIAN_POINT ( 'NONE',  ( 109.7880358795247986, -0.7896495226426338832, -17.46756447353520159 ) ) ;
#21808=CARTESIAN_POINT ( 'NONE',  ( 109.2294421292701543, -7.690995191147263377, -8.440827004729632321 ) ) ;
#21810=CARTESIAN_POINT ( 'NONE',  ( 115.9693640045247776, -10.62599879583958717, -11.00651665394454604 ) ) ;
#21812=CARTESIAN_POINT ( 'NONE',  ( 117.2294421295248270, 0.7813447578650477565, -21.83687654715277304 ) ) ;
#21815=CARTESIAN_POINT ( 'NONE',  ( 112.4967077545247633, -7.250697342233347165, -7.631215200338321125 ) ) ;
#21821=AXIS2_PLACEMENT_3D ( 'NONE', #942, #14861, #15525 ) ;
#21827=CARTESIAN_POINT ( 'NONE',  ( 114.0246765045248196, -7.250697342233347165, -19.15521520033831138 ) ) ;
#21840=CARTESIAN_POINT ( 'NONE',  ( 77.59349808546981819, -56.93324028847530371, -1.549987343799404726 ) ) ;
#21841=CARTESIAN_POINT ( 'NONE',  ( 64.06704089363852006, -35.12954632779501907, -5.893215200338315363 ) ) ;
#21851=LINE ( 'NONE', #3837, #28605 ) ;
#21853=VERTEX_POINT ( 'NONE', #13658 ) ;
#21855=CARTESIAN_POINT ( 'NONE',  ( 112.0105358795248804, -8.402594152722688392, -9.854619843455216355 ) ) ;
#21857=CARTESIAN_POINT ( 'NONE',  ( 114.0246765045248196, -2.791137627527939813, -8.388885654883754484 ) ) ;
#21868=CARTESIAN_POINT ( 'NONE',  ( 105.8986608795248401, -1.325403438956436419, -16.93181055722141792 ) ) ;
#21869=ORIENTED_EDGE ( 'NONE', *, *, #23779, .F. ) ;
#21874=EDGE_CURVE ( 'NONE', #30236, #25264, #24146, .T. ) ;
#21890=VECTOR ( 'NONE', #6514, 1000.000000000000000 ) ;
#21898=DIRECTION ( 'NONE',  ( 1.000000000000000000, 0.000000000000000000, 0.000000000000000000 ) ) ;
#21901=CARTESIAN_POINT ( 'NONE',  ( 116.6387481731040481, -9.478760661942724042, -15.43013221979977700 ) ) ;
#21903=CYLINDRICAL_SURFACE ( 'NONE', #5831, 0.9999999999999952260 ) ;
#21909=CARTESIAN_POINT ( 'NONE',  ( 105.7597546295248350, -4.863998795839590272, -7.631215200338315796 ) ) ;
#21910=CARTESIAN_POINT ( 'NONE',  ( 112.9828796295247884, -4.863998795839590272, -8.388885654883775800 ) ) ;
#21914=ORIENTED_EDGE ( 'NONE', *, *, #8067, .T. ) ;
#21916=CARTESIAN_POINT ( 'NONE',  ( 106.3153796295248412, -4.863998795839590272, -19.15521520033831493 ) ) ;
#21917=CARTESIAN_POINT ( 'NONE',  ( 70.19691569158496236, 3.834886253390165756, -4.893215200338314474 ) ) ;
#21919=DIRECTION ( 'NONE',  ( -0.9387755102040816757, 0.3445294493088600918, 0.000000000000000000 ) ) ;
#21922=CARTESIAN_POINT ( 'NONE',  ( 114.9970202545248412, -10.62599879583958717, -15.77991374673208469 ) ) ;
#21923=CARTESIAN_POINT ( 'NONE',  ( 113.3301452545248083, -9.868328341294098749, -15.46607636864997204 ) ) ;
#21939=CARTESIAN_POINT ( 'NONE',  ( 110.7640389883689807, 0.3193521225029610777, -12.14321520033833224 ) ) ;
#21942=CARTESIAN_POINT ( 'NONE',  ( 107.8433483795247838, -8.402594152722688392, -16.93181055722141792 ) ) ;
#21953=CARTESIAN_POINT ( 'NONE',  ( 71.67504600870660170, -26.72445618319088823, -4.893215200338314474 ) ) ;
#21954=CARTESIAN_POINT ( 'NONE',  ( 113.0523327545247838, -2.477300249445798297, -19.15521520033831138 ) ) ;
#21958=ADVANCED_FACE ( 'NONE', ( #31410 ), #41262, .F. ) ;
#21962=EDGE_CURVE ( 'NONE', #12848, #30236, #16273, .T. ) ;
#21968=CARTESIAN_POINT ( 'NONE',  ( 117.0174177730625900, 0.4131681913238580139, -12.14321520033831625 ) ) ;
#21973=CARTESIAN_POINT ( 'NONE',  ( 113.7468640045248236, -10.62599879583958717, -11.00651665394454604 ) ) ;
#21978=CARTESIAN_POINT ( 'NONE',  ( 105.3430358795248338, -8.402594152722688392, -9.854619843455216355 ) ) ;
#21980=CARTESIAN_POINT ( 'NONE',  ( 116.5564130180080866, 0.7607806665037644134, -14.64321520033833401 ) ) ;
#21981=CARTESIAN_POINT ( 'NONE',  ( 109.2294421291983184, -10.01537527712310549, -11.01699420138576180 ) ) ;
#21984=CARTESIAN_POINT ( 'NONE',  ( 111.5938171295247940, 0.1403307496149613920, -13.39321520033831447 ) ) ;
#21985=CARTESIAN_POINT ( 'NONE',  ( 115.4137390045248566, -9.868328341294098749, -11.32035403202665869 ) ) ;
#21992=ADVANCED_FACE ( 'NONE', ( #14092 ), #20274, .F. ) ;
#22001=CARTESIAN_POINT ( 'NONE',  ( 108.3989733795248753, -8.938348069036489818, -17.46756447353520159 ) ) ;
#22003=CYLINDRICAL_SURFACE ( 'NONE', #30270, 8.000000000000000000 ) ;
#22004=CARTESIAN_POINT ( 'NONE',  ( 112.5661608795247872, -1.325403438956436419, -16.93181055722141792 ) ) ;
#22011=EDGE_CURVE ( 'NONE', #29903, #32851, #13385, .T. ) ;
#22013=CARTESIAN_POINT ( 'NONE',  ( 110.4131140045248287, 0.1403307496149616695, -15.46607636864997204 ) ) ;
#22024=EDGE_CURVE ( 'NONE', #41199, #424, #24280, .T. ) ;
#22026=CARTESIAN_POINT ( 'NONE',  ( 115.2053796295247849, -4.863998795839590272, -8.388885654883775800 ) ) ;
#22031=CARTESIAN_POINT ( 'NONE',  ( 109.9269421295247753, 0.8980012041604618078, -13.39321520033831447 ) ) ;
#22037=CARTESIAN_POINT ( 'NONE',  ( 115.2748327545248657, -2.477300249445798297, -19.15521520033831138 ) ) ;
#22038=CARTESIAN_POINT ( 'NONE',  ( 117.1512660175612126, 1.479770359400331747, -21.46523989841215396 ) ) ;
#22039=CARTESIAN_POINT ( 'NONE',  ( 83.83011982744213242, -31.85041140898378487, -20.99942768933297543 ) ) ;
#22043=( BOUNDED_CURVE ( )  B_SPLINE_CURVE ( 3, ( #9291, #23200, #9976, #13615 ),
 .UNSPECIFIED., .F., .F. ) 
 B_SPLINE_CURVE_WITH_KNOTS ( ( 4, 4 ),
 ( 0.6164973811836809148, 1.570796326794899889 ),
 .UNSPECIFIED. ) 
 CURVE ( )  GEOMETRIC_REPRESENTATION_ITEM ( )  RATIONAL_B_SPLINE_CURVE ( ( 1.000000000000000000, 0.9255384209705479481, 0.9255384209705479481, 1.000000000000000000 ) ) 
 REPRESENTATION_ITEM ( '' )  );
#22047=LINE ( 'NONE', #1958, #10153 ) ;
#22048=VECTOR ( 'NONE', #42954, 1000.000000000000000 ) ;
#22054=CARTESIAN_POINT ( 'NONE',  ( 115.3442858795247759, -0.7896495226426338832, -17.46756447353520159 ) ) ;
#22060=EDGE_CURVE ( 'NONE', #11967, #30697, #4040, .T. ) ;
#22064=LINE ( 'NONE', #15447, #13123 ) ;
#22066=CARTESIAN_POINT ( 'NONE',  ( 115.2566360982116862, 0.3867979994853637526, -12.14321520033831625 ) ) ;
#22073=CIRCLE ( 'NONE', #38084, 2.999999999999998224 ) ;
#22087=CARTESIAN_POINT ( 'NONE',  ( 113.8857702545248003, 0.1403307496149616695, -11.32035403202665336 ) ) ;
#22088=CARTESIAN_POINT ( 'NONE',  ( 82.53726425729240646, -31.76580277050288004, -22.96761734921603448 ) ) ;
#22092=CARTESIAN_POINT ( 'NONE',  ( 115.8999108795247821, -1.325403438956436419, -16.93181055722141792 ) ) ;
#22098=CARTESIAN_POINT ( 'NONE',  ( 107.4266296295248821, -4.863998795839590272, -8.388885654883775800 ) ) ;
#22101=LINE ( 'NONE', #25972, #7269 ) ;
#22106=FACE_OUTER_BOUND ( 'NONE', #34860, .T. ) ;
#22109=CARTESIAN_POINT ( 'NONE',  ( 115.1359265045248605, -2.791137627527939813, -8.388885654883777576 ) ) ;
#22110=AXIS2_PLACEMENT_3D ( 'NONE', #41309, #41742, #24190 ) ;
#22113=ORIENTED_EDGE ( 'NONE', *, *, #35208, .F. ) ;
#22116=CARTESIAN_POINT ( 'NONE',  ( 105.6208483795248299, -0.7896495226426338832, -9.318865927141430916 ) ) ;
#22130=CARTESIAN_POINT ( 'NONE',  ( 116.6466789632009835, -9.331272246221795186, -15.78281339210872680 ) ) ;
#22137=CARTESIAN_POINT ( 'NONE',  ( 70.19189222814998175, -40.46710316615127567, -32.62080435916936239 ) ) ;
#22138=CARTESIAN_POINT ( 'NONE',  ( 109.7880358795247986, -8.402594152722688392, -9.854619843455216355 ) ) ;
#22139=CARTESIAN_POINT ( 'NONE',  ( 113.8857702545248003, 0.1403307496149616695, -11.32035403202665336 ) ) ;
#22144=CARTESIAN_POINT ( 'NONE',  ( 109.0935046295247872, -4.863998795839590272, -7.631215200338315796 ) ) ;
#22148=CARTESIAN_POINT ( 'NONE',  ( 87.44708369096657918, -25.99489077589588604, -12.39321520033831447 ) ) ;
#22150=CARTESIAN_POINT ( 'NONE',  ( 112.1494421295248003, 0.8980012041604618078, -13.39321520033831447 ) ) ;
#22151=CARTESIAN_POINT ( 'NONE',  ( 110.8992858795247827, -8.402594152722688392, -9.854619843455216355 ) ) ;
#22162=CARTESIAN_POINT ( 'NONE',  ( 64.84865456828643460, -21.86021636429758530, -5.893215200338315363 ) ) ;
#22164=ORIENTED_EDGE ( 'NONE', *, *, #24471, .F. ) ;
#22167=CARTESIAN_POINT ( 'NONE',  ( 108.1906140045248037, 0.1403307496149616695, -15.46607636864997204 ) ) ;
#22175=ORIENTED_EDGE ( 'NONE', *, *, #35777, .T. ) ;
#22177=CARTESIAN_POINT ( 'NONE',  ( 62.56519830863885545, -64.88825862050514104, -45.66019302834368432 ) ) ;
#22178=CARTESIAN_POINT ( 'NONE',  ( 109.8574890045247940, 0.8980012041604421569, -15.77991374673208469 ) ) ;
#22183=DIRECTION ( 'NONE',  ( 0.000000000000000000, -0.7876185884367603585, 0.6161630946014904353 ) ) ;
#22189=CARTESIAN_POINT ( 'NONE',  ( 116.7333483795247844, -8.402594152722688392, -16.93181055722141792 ) ) ;
#22190=CARTESIAN_POINT ( 'NONE',  ( 114.2330358795247776, -0.7896495226426338832, -17.46756447353520159 ) ) ;
#22195=CARTESIAN_POINT ( 'NONE',  ( 106.0375671295248310, -10.62599879583958540, -13.39321520033831447 ) ) ;
#22200=LINE ( 'NONE', #8522, #41011 ) ;
#22204=CARTESIAN_POINT ( 'NONE',  ( 109.2294476533355692, -10.02000977116478708, -15.26446378573822038 ) ) ;
#22206=CARTESIAN_POINT ( 'NONE',  ( 110.7603796295247918, -4.863998795839590272, -8.388885654883775800 ) ) ;
#22207=CARTESIAN_POINT ( 'NONE',  ( 115.0664733795247798, -1.325403438956436419, -9.854619843455211026 ) ) ;
#22216=B_SPLINE_CURVE_WITH_KNOTS ( 'NONE', 3,
 ( #21210, #2983, #38085, #27835, #41314, #41748, #10509, #13488, #14369, #24410, #28283, #24634, #38300 ),
 .UNSPECIFIED., .F., .F.,
 ( 4, 3, 3, 3, 4 ),
 ( 2.934973642780345169E-16, 1.132108791046253874E-05, 5.660632326038089941E-05, 0.0001397594989357112019, 0.0002229354582960460030 ),
 .UNSPECIFIED. ) ;
#22218=VERTEX_POINT ( 'NONE', #28683 ) ;
#22220=EDGE_CURVE ( 'NONE', #31523, #39064, #4722, .T. ) ;
#22221=CIRCLE ( 'NONE', #28059, 5.000000000000004441 ) ;
#22227=CARTESIAN_POINT ( 'NONE',  ( 112.0105358795247810, -8.402594152722688392, -9.854619843455216355 ) ) ;
#22232=CARTESIAN_POINT ( 'NONE',  ( 117.0111608795247946, -1.325403438956436419, -16.93181055722141792 ) ) ;
#22233=CARTESIAN_POINT ( 'NONE',  ( 111.8716296295247901, -4.863998795839590272, -8.388885654883775800 ) ) ;
#22240=VECTOR ( 'NONE', #32937, 1000.000000000000000 ) ;
#22245=CARTESIAN_POINT ( 'NONE',  ( 108.8851452545248151, -9.868328341294098749, -15.46607636864997204 ) ) ;
#22252=CARTESIAN_POINT ( 'NONE',  ( 107.2877233795247776, -8.938348069036489818, -17.46756447353520159 ) ) ;
#22256=CARTESIAN_POINT ( 'NONE',  ( 109.2294421295247844, 7.836001204160461420, -12.14321520033831625 ) ) ;
#22259=CARTESIAN_POINT ( 'NONE',  ( 116.3166296295247832, -4.863998795839590272, -19.15521520033831493 ) ) ;
#22261=CARTESIAN_POINT ( 'NONE',  ( 83.86185565543740950, -31.76393747133379009, -22.76090678561018521 ) ) ;
#22264=CARTESIAN_POINT ( 'NONE',  ( 105.9681140045248355, -10.62599879583958717, -11.00651665394454604 ) ) ;
#22268=DIRECTION ( 'NONE',  ( 1.000000000000000000, 0.000000000000000000, 0.000000000000000000 ) ) ;
#22270=EDGE_CURVE ( 'NONE', #27865, #35613, #31859, .T. ) ;
#22279=CARTESIAN_POINT ( 'NONE',  ( 113.0523327545247838, -2.477300249445798297, -19.15521520033831138 ) ) ;
#22281=FACE_OUTER_BOUND ( 'NONE', #21720, .T. ) ;
#22290=DIRECTION ( 'NONE',  ( -1.000000000000000000, 0.000000000000000000, 0.000000000000000000 ) ) ;
#22304=( BOUNDED_SURFACE ( )  B_SPLINE_SURFACE ( 1, 2, ( 
 ( #40013, #32926, #36128, #29529, #2377, #40476, #5356, #1927, #19272, #16307, #5123, #12665, #8778, #33151, #1478, #1702, #40701 ),
 ( #16075, #15853, #22232, #15399, #19494, #8557, #43661, #22458, #36352, #26336, #40243, #22909, #43896, #36802, #5570, #3066, #17426 ) ),
 .UNSPECIFIED., .F., .F., .T. ) 
 B_SPLINE_SURFACE_WITH_KNOTS ( ( 2, 2 ),
 ( 3, 2, 2, 2, 2, 2, 2, 2, 3 ),
 ( 0.000000000000000000, 1.000000000000000000 ),
 ( 0.000000000000000000, 0.1250000000000000000, 0.2500000000000000000, 0.3750000000000000000, 0.5000000000000000000, 0.6250000000000000000, 0.7500000000000000000, 0.8750000000000000000, 1.000000000000000000 ),
 .UNSPECIFIED. ) 
 GEOMETRIC_REPRESENTATION_ITEM ( )  RATIONAL_B_SPLINE_SURFACE ( (
 ( 1.000000000000000000, 0.9238795325112869605, 1.000000000000000000, 0.9238795325112869605, 1.000000000000000000, 0.9238795325112869605, 1.000000000000000000, 0.9238795325112869605, 1.000000000000000000, 0.9238795325112869605, 1.000000000000000000, 0.9238795325112869605, 1.000000000000000000, 0.9238795325112869605, 1.000000000000000000, 0.9238795325112869605, 1.000000000000000000),
 ( 1.000000000000000000, 0.9238795325112869605, 1.000000000000000000, 0.9238795325112869605, 1.000000000000000000, 0.9238795325112869605, 1.000000000000000000, 0.9238795325112869605, 1.000000000000000000, 0.9238795325112869605, 1.000000000000000000, 0.9238795325112869605, 1.000000000000000000, 0.9238795325112869605, 1.000000000000000000, 0.9238795325112869605, 1.000000000000000000) ) ) 
 REPRESENTATION_ITEM ( '' )  SURFACE ( )  );
#22308=CARTESIAN_POINT ( 'NONE',  ( 106.6626452545248611, -9.868328341294098749, -15.46607636864997204 ) ) ;
#22309=CARTESIAN_POINT ( 'NONE',  ( 112.9828796295247884, -4.863998795839590272, -8.388885654883775800 ) ) ;
#22320=CARTESIAN_POINT ( 'NONE',  ( 105.7597546295248350, -4.863998795839590272, -18.39754474579285315 ) ) ;
#22322=VERTEX_POINT ( 'NONE', #39156 ) ;
#22330=VERTEX_POINT ( 'NONE', #18185 ) ;
#22332=CARTESIAN_POINT ( 'NONE',  ( 117.0806140045248185, 0.1403307496149616695, -15.46607636864997204 ) ) ;
#22335=ORIENTED_EDGE ( 'NONE', *, *, #29791, .T. ) ;
#22343=AXIS2_PLACEMENT_3D ( 'NONE', #5777, #19474, #30418 ) ;
#22346=CARTESIAN_POINT ( 'NONE',  ( 115.0646051332721811, 0.2334052082820642360, -14.64321520033831447 ) ) ;
#22353=CARTESIAN_POINT ( 'NONE',  ( 116.6382829425946284, -9.487340216247861946, -15.40942383360363799 ) ) ;
#22361=CARTESIAN_POINT ( 'NONE',  ( 109.1629577545248395, -2.791137627527939813, -18.39754474579286025 ) ) ;
#22362=CARTESIAN_POINT ( 'NONE',  ( 107.9822546295247889, -4.863998795839590272, -18.39754474579285315 ) ) ;
#22366=CARTESIAN_POINT ( 'NONE',  ( 106.8015515045248378, -2.477300249445798297, -7.631215200338321125 ) ) ;
#22369=CARTESIAN_POINT ( 'NONE',  ( 109.2294421295247844, 0.1210096558822565393, -14.64321520034217805 ) ) ;
#22372=CARTESIAN_POINT ( 'NONE',  ( 108.9545983795247821, -0.7896495226426338832, -9.318865927141430916 ) ) ;
#22373=CARTESIAN_POINT ( 'NONE',  ( 112.2883483795247770, -8.402594152722688392, -16.93181055722141792 ) ) ;
#22386=CARTESIAN_POINT ( 'NONE',  ( 113.6298959279789784, 0.1843591316377651834, -14.64321520033831447 ) ) ;
#22388=VERTEX_POINT ( 'NONE', #43032 ) ;
#22392=CARTESIAN_POINT ( 'NONE',  ( 115.8304577545247582, -7.250697342233347165, -7.631215200338321125 ) ) ;
#22401=CARTESIAN_POINT ( 'NONE',  ( 71.79922130029189020, -25.12209812792223929, -4.893215200338314474 ) ) ;
#22402=CARTESIAN_POINT ( 'NONE',  ( 112.0799890045248475, 0.8980012041604421569, -15.77991374673208469 ) ) ;
#22404=AXIS2_PLACEMENT_3D ( 'NONE', #44585, #19720, #23609 ) ;
#22409=DIRECTION ( 'NONE',  ( 0.000000000000000000, 1.000000000000000000, 0.000000000000000000 ) ) ;
#22413=CARTESIAN_POINT ( 'NONE',  ( 111.3160046295247838, -4.863998795839590272, -7.631215200338315796 ) ) ;
#22415=CARTESIAN_POINT ( 'NONE',  ( 110.9687390045248350, 0.8980012041604421569, -15.77991374673208469 ) ) ;
#22420=CARTESIAN_POINT ( 'NONE',  ( 109.0240515045248202, -2.477300249445798297, -7.631215200338321125 ) ) ;
#22425=DIRECTION ( 'NONE',  ( 0.000000000000000000, 0.000000000000000000, 1.000000000000000000 ) ) ;
#22428=CARTESIAN_POINT ( 'NONE',  ( 109.2294419231370597, -10.34583128743581426, -14.16414405063035531 ) ) ;
#22430=CARTESIAN_POINT ( 'NONE',  ( 112.1494421295248003, -9.868328341294093420, -13.39321520033831447 ) ) ;
#22431=CARTESIAN_POINT ( 'NONE',  ( 106.3848327545248651, -2.477300249445798297, -19.15521520033831138 ) ) ;
#22434=CARTESIAN_POINT ( 'NONE',  ( 68.96715889846213088, -25.99505776776173960, -5.893215200338315363 ) ) ;
#22451=CARTESIAN_POINT ( 'NONE',  ( 114.5803015045248117, -6.936859964151250502, -18.39754474579286025 ) ) ;
#22453=FACE_OUTER_BOUND ( 'NONE', #26799, .T. ) ;
#22458=CARTESIAN_POINT ( 'NONE',  ( 116.6638952545248031, -9.868328341294098749, -15.46607636864997204 ) ) ;
#22459=CARTESIAN_POINT ( 'NONE',  ( 111.8021765045248372, -2.791137627527939813, -8.388885654883777576 ) ) ;
#22467=ORIENTED_EDGE ( 'NONE', *, *, #44574, .F. ) ;
#22470=CARTESIAN_POINT ( 'NONE',  ( 107.9822546295247889, -4.863998795839590272, -18.39754474579285315 ) ) ;
#22476=CARTESIAN_POINT ( 'NONE',  ( 107.4266296295248821, -4.863998795839590272, -19.15521520033831493 ) ) ;
#22479=DIRECTION ( 'NONE',  ( 0.000000000000000000, 0.000000000000000000, -1.000000000000000000 ) ) ;
#22480=DIRECTION ( 'NONE',  ( 0.000000000000000000, 0.9284778069183718952, 0.3713878862591650232 ) ) ;
#22481=CARTESIAN_POINT ( 'NONE',  ( 114.2330358795247776, -0.7896495226426338832, -17.46756447353520159 ) ) ;
#22483=CARTESIAN_POINT ( 'NONE',  ( 83.86641712191145359, -31.75150836541887145, -22.59176852388810630 ) ) ;
#22486=CARTESIAN_POINT ( 'NONE',  ( 106.5931921295248372, 0.8980012041604618078, -13.39321520033831447 ) ) ;
#22490=CARTESIAN_POINT ( 'NONE',  ( 116.3892577545247491, -6.935066607705044461, -8.393215200338321580 ) ) ;
#22497=CARTESIAN_POINT ( 'NONE',  ( 109.3713171295247832, -10.62599879583958540, -13.39321520033831447 ) ) ;
#22498=VECTOR ( 'NONE', #11337, 1000.000000000000000 ) ;
#22500=CARTESIAN_POINT ( 'NONE',  ( 116.7819514645520940, -3.568899806858861101, -18.41715839113304298 ) ) ;
#22507=DIRECTION ( 'NONE',  ( 0.000000000000000000, 0.000000000000000000, 1.000000000000000000 ) ) ;
#22511=CARTESIAN_POINT ( 'NONE',  ( 64.18561586838816879, -35.08338226378547375, -5.893215200338315363 ) ) ;
#22513=CARTESIAN_POINT ( 'NONE',  ( 109.5990301496069748, 0.3591747506842615789, -14.64321520033828605 ) ) ;
#22522=CARTESIAN_POINT ( 'NONE',  ( 115.8304577545247582, -2.791137627527939813, -18.39754474579286025 ) ) ;
#22524=EDGE_CURVE ( 'NONE', #20631, #29947, #2861, .T. ) ;
#22528=CARTESIAN_POINT ( 'NONE',  ( 116.5944421295247793, 0.8980012041604618078, -13.39321520033831447 ) ) ;
#22529=CARTESIAN_POINT ( 'NONE',  ( 108.1211608795247798, -1.325403438956436419, -16.93181055722141792 ) ) ;
#22540=CARTESIAN_POINT ( 'NONE',  ( 109.5796765045248122, -2.791137627527939813, -8.388885654883777576 ) ) ;
#22541=ORIENTED_EDGE ( 'NONE', *, *, #43404, .F. ) ;
#22549=CARTESIAN_POINT ( 'NONE',  ( 111.4549108795247747, -1.325403438956436419, -16.93181055722141792 ) ) ;
#22561=FACE_OUTER_BOUND ( 'NONE', #44956, .T. ) ;
#22562=CARTESIAN_POINT ( 'NONE',  ( 109.4644545411903209, -0.3595008806742185925, -10.82052240173742419 ) ) ;
#22566=DIRECTION ( 'NONE',  ( 0.000000000000000000, 0.000000000000000000, 1.000000000000000000 ) ) ;
#22567=VECTOR ( 'NONE', #35476, 1000.000000000000000 ) ;
#22572=CARTESIAN_POINT ( 'NONE',  ( 116.6670768749042821, -8.779456523914790367, -16.62141271327601899 ) ) ;
#22580=CARTESIAN_POINT ( 'NONE',  ( 110.2047546295247855, -4.863998795839590272, -7.631215200338315796 ) ) ;
#22581=CARTESIAN_POINT ( 'NONE',  ( 109.5102233795247884, -1.325403438956436419, -9.854619843455211026 ) ) ;
#22582=CARTESIAN_POINT ( 'NONE',  ( 109.5102233795247884, -1.325403438956436419, -9.854619843455211026 ) ) ;
#22587=CARTESIAN_POINT ( 'NONE',  ( 108.0517077545248696, -7.250697342233347165, -7.631215200338321125 ) ) ;
#22588=DIRECTION ( 'NONE',  ( 0.000000000000000000, 0.000000000000000000, 1.000000000000000000 ) ) ;
#22593=CARTESIAN_POINT ( 'NONE',  ( 109.0935046295247872, -4.863998795839590272, -7.631215200338315796 ) ) ;
#22594=CARTESIAN_POINT ( 'NONE',  ( 71.37572422742091760, -11.86958442233774313, -21.39321520033831447 ) ) ;
#22613=CARTESIAN_POINT ( 'NONE',  ( 115.7610046295247912, -4.863998795839590272, -7.631215200338315796 ) ) ;
#22614=DIRECTION ( 'NONE',  ( -0.6836572958096076569, 0.7298031939408696767, 0.000000000000000000 ) ) ;
#22619=LINE ( 'NONE', #8495, #43287 ) ;
#22624=CARTESIAN_POINT ( 'NONE',  ( 106.7320983795247855, -0.7896495226426338832, -9.318865927141430916 ) ) ;
#22625=AXIS2_PLACEMENT_3D ( 'NONE', #4973, #8630, #1327 ) ;
#22634=CARTESIAN_POINT ( 'NONE',  ( 110.8298327545248299, -2.477300249445798297, -19.15521520033831138 ) ) ;
#22637=CARTESIAN_POINT ( 'NONE',  ( 112.4272546295247821, -4.863998795839590272, -7.631215200338315796 ) ) ;
#22643=CARTESIAN_POINT ( 'NONE',  ( 62.99487470011365531, -37.68830414585190169, -5.018140281204638953 ) ) ;
#22644=CARTESIAN_POINT ( 'NONE',  ( 108.5378796295247810, -4.863998795839590272, -19.15521520033831493 ) ) ;
#22648=CARTESIAN_POINT ( 'NONE',  ( 116.5432357643689727, -11.91225050823456755, -6.526147773411142161 ) ) ;
#22651=CARTESIAN_POINT ( 'NONE',  ( 109.2294422610953291, -10.06140057338842020, -15.16114099083124778 ) ) ;
#22653=CARTESIAN_POINT ( 'NONE',  ( 110.9687390045248350, -9.868328341294098749, -11.32035403202665869 ) ) ;
#22654=CARTESIAN_POINT ( 'NONE',  ( 114.5803015045248117, -6.936859964151250502, -18.39754474579286025 ) ) ;
#22657=CARTESIAN_POINT ( 'NONE',  ( 69.18853725737697857, -25.71063077209354120, -5.871568482255375976 ) ) ;
#22666=EDGE_LOOP ( 'NONE', ( #14440, #5062, #13520, #18129, #10647, #38378, #29063, #34068, #37989, #7348, #7679, #19796, #29270, #21432, #3537, #25378 ) ) ;
#22672=CARTESIAN_POINT ( 'NONE',  ( 107.1488171295247867, -10.62599879583958540, -13.39321520033831447 ) ) ;
#22675=CARTESIAN_POINT ( 'NONE',  ( 107.2182702545248105, 0.1403307496149616695, -11.32035403202665336 ) ) ;
#22676=DIRECTION ( 'NONE',  ( 0.000000000000000000, 1.000000000000000000, 0.000000000000000000 ) ) ;
#22681=ORIENTED_EDGE ( 'NONE', *, *, #26130, .T. ) ;
#22683=CARTESIAN_POINT ( 'NONE',  ( 112.4967077545247633, -2.791137627527939813, -18.39754474579286025 ) ) ;
#22689=DIRECTION ( 'NONE',  ( -0.9387755102040796773, 0.3445294493088653653, 0.000000000000000000 ) ) ;
#22691=ADVANCED_FACE ( 'NONE', ( #12027 ), #21501, .T. ) ;
#22696=CARTESIAN_POINT ( 'NONE',  ( 109.7185827545247889, -6.936859964151250502, -8.388885654883777576 ) ) ;
#22701=CARTESIAN_POINT ( 'NONE',  ( 107.4960827545248350, -2.477300249445798297, -19.15521520033831138 ) ) ;
#22702=DIRECTION ( 'NONE',  ( 0.000000000000000000, -1.000000000000000000, 0.000000000000000000 ) ) ;
#22704=CARTESIAN_POINT ( 'NONE',  ( 110.2047546295247855, -4.863998795839590272, -7.631215200338315796 ) ) ;
#22706=CARTESIAN_POINT ( 'NONE',  ( 82.42940256598244275, -31.76384415549768292, -22.80862274410626256 ) ) ;
#22719=CARTESIAN_POINT ( 'NONE',  ( 107.1488171295247867, -10.62599879583958540, -13.39321520033831447 ) ) ;
#22721=CARTESIAN_POINT ( 'NONE',  ( 69.69189222814998175, -41.76310523276723785, -24.89321520033831447 ) ) ;
#22722=CARTESIAN_POINT ( 'NONE',  ( 116.1777233795247781, -8.938348069036489818, -17.46756447353520159 ) ) ;
#22724=B_SPLINE_CURVE_WITH_KNOTS ( 'NONE', 3,
 ( #15547, #39497, #29452, #25372, #39041, #21939, #8706, #39944, #28793, #8260 ),
 .UNSPECIFIED., .F., .F.,
 ( 4, 3, 3, 4 ),
 ( 0.000000000000000000, 0.0002476487219222849707, 0.0004952974148303729719, 0.0009534114850261750764 ),
 .UNSPECIFIED. ) ;
#22743=CARTESIAN_POINT ( 'NONE',  ( 113.3301452545248083, -9.868328341294098749, -15.46607636864997204 ) ) ;
#22748=CARTESIAN_POINT ( 'NONE',  ( 114.4413952545248350, 0.8980012041604421569, -11.00651665394454071 ) ) ;
#22749=CARTESIAN_POINT ( 'NONE',  ( 110.7603796295247918, -4.863998795839590272, -8.388885654883775800 ) ) ;
#22754=CARTESIAN_POINT ( 'NONE',  ( 112.9828796295247884, -4.863998795839590272, -8.388885654883775800 ) ) ;
#22761=CARTESIAN_POINT ( 'NONE',  ( 106.4542858795248179, -8.402594152722688392, -9.854619843455216355 ) ) ;
#22771=CARTESIAN_POINT ( 'NONE',  ( 112.9828796295247884, -4.863998795839590272, -8.388885654883775800 ) ) ;
#22775=VERTEX_POINT ( 'NONE', #7198 ) ;
#22779=EDGE_CURVE ( 'NONE', #970, #28048, #19942, .T. ) ;
#22781=VECTOR ( 'NONE', #29663, 1000.000000000000000 ) ;
#22784=ORIENTED_EDGE ( 'NONE', *, *, #1026, .F. ) ;
#22791=DIRECTION ( 'NONE',  ( -0.6383198453882292789, -0.7697712484781092934, 0.000000000000000000 ) ) ;
#22792=VECTOR ( 'NONE', #32256, 1000.000000000000000 ) ;
#22803=CARTESIAN_POINT ( 'NONE',  ( 109.7880358795247986, -0.7896495226426338832, -17.46756447353520159 ) ) ;
#22805=CARTESIAN_POINT ( 'NONE',  ( 109.0240515045248202, -6.936859964151250502, -18.39754474579286025 ) ) ;
#22806=CARTESIAN_POINT ( 'NONE',  ( 108.0517077545248696, -2.791137627527939813, -18.39754474579286025 ) ) ;
#22809=ORIENTED_EDGE ( 'NONE', *, *, #25664, .T. ) ;
#22818=CARTESIAN_POINT ( 'NONE',  ( 109.7880358795247986, -0.7896495226426338832, -17.46756447353520159 ) ) ;
#22830=ORIENTED_EDGE ( 'NONE', *, *, #18972, .T. ) ;
#22836=EDGE_CURVE ( 'NONE', #44158, #32023, #39432, .T. ) ;
#22841=CARTESIAN_POINT ( 'NONE',  ( 113.3995983795247895, -0.7896495226426338832, -9.318865927141430916 ) ) ;
#22844=ORIENTED_EDGE ( 'NONE', *, *, #16974, .F. ) ;
#22850=CARTESIAN_POINT ( 'NONE',  ( 61.80622722289361093, -65.84395357266009796, -43.65918878370688105 ) ) ;
#22861=CARTESIAN_POINT ( 'NONE',  ( 112.9828796295247884, -4.863998795839590272, -19.15521520033831493 ) ) ;
#22863=CARTESIAN_POINT ( 'NONE',  ( 113.7468640045248236, -10.62599879583958717, -11.00651665394454604 ) ) ;
#22868=CARTESIAN_POINT ( 'NONE',  ( 107.6349890045248401, 0.8980012041604421569, -15.77991374673208469 ) ) ;
#22872=LINE ( 'NONE', #18560, #22048 ) ;
#22875=CARTESIAN_POINT ( 'NONE',  ( 109.2295804820058436, -10.43592689531145190, -13.30118990145861702 ) ) ;
#22877=CARTESIAN_POINT ( 'NONE',  ( 113.6774108795247997, -1.325403438956436419, -16.93181055722141792 ) ) ;
#22878=CARTESIAN_POINT ( 'NONE',  ( 111.3854577545248645, -2.791137627527939813, -18.39754474579286025 ) ) ;
#22881=CARTESIAN_POINT ( 'NONE',  ( 71.20716749095201692, -24.93145248074033660, -5.218938316983485315 ) ) ;
#22884=ADVANCED_FACE ( 'NONE', ( #12206 ), #32705, .F. ) ;
#22885=ORIENTED_EDGE ( 'NONE', *, *, #1868, .T. ) ;
#22886=CIRCLE ( 'NONE', #1807, 5.132259260909266985 ) ;
#22897=CARTESIAN_POINT ( 'NONE',  ( 107.2877233795247776, -8.938348069036489818, -17.46756447353520159 ) ) ;
#22898=B_SPLINE_CURVE_WITH_KNOTS ( 'NONE', 3,
 ( #44863, #41443, #41667, #44637, #37316, #6087, #31157, #13619, #27527, #27075 ),
 .UNSPECIFIED., .F., .F.,
 ( 4, 3, 3, 4 ),
 ( 0.000000000000000000, 0.0002476486447138875262, 0.0004952972925464290419, 0.0009604418836934499335 ),
 .UNSPECIFIED. ) ;
#22902=CARTESIAN_POINT ( 'NONE',  ( 108.6767858795247861, -8.402594152722688392, -9.854619843455216355 ) ) ;
#22909=CARTESIAN_POINT ( 'NONE',  ( 116.3860827545247787, -6.936859964151250502, -8.388885654883777576 ) ) ;
#22910=CARTESIAN_POINT ( 'NONE',  ( 107.9822546295247889, -4.863998795839590272, -18.39754474579285315 ) ) ;
#22916=CARTESIAN_POINT ( 'NONE',  ( 69.04371756932381743, -26.05018752390734349, -5.893215200338321580 ) ) ;
#22919=ORIENTED_EDGE ( 'NONE', *, *, #36970, .T. ) ;
#22920=CARTESIAN_POINT ( 'NONE',  ( 84.87879901378997261, -30.44422003934618814, -8.393215200338314474 ) ) ;
#22922=CARTESIAN_POINT ( 'NONE',  ( 108.4684265045247997, -2.791137627527939813, -8.388885654883777576 ) ) ;
#22926=CARTESIAN_POINT ( 'NONE',  ( 116.0388171295248014, 0.1403307496149613920, -13.39321520033831447 ) ) ;
#22929=DIRECTION ( 'NONE',  ( 1.000000000000000000, 2.439015257082815255E-15, 0.000000000000000000 ) ) ;
#22930=CARTESIAN_POINT ( 'NONE',  ( 109.3018640045248304, -10.62599879583958717, -11.00651665394454604 ) ) ;
#22931=CARTESIAN_POINT ( 'NONE',  ( 116.3539803407245046, 2.267523965085636917, -20.30237287253366674 ) ) ;
#22932=CARTESIAN_POINT ( 'NONE',  ( 113.9552233795247815, -8.938348069036489818, -17.46756447353520159 ) ) ;
#22935=CARTESIAN_POINT ( 'NONE',  ( 108.5378796295247810, -4.863998795839590272, -19.15521520033831493 ) ) ;
#22940=B_SPLINE_CURVE_WITH_KNOTS ( 'NONE', 3,
 ( #30665, #26569, #12443, #19953, #20189, #23151, #16543, #2840, #19500, #44134 ),
 .UNSPECIFIED., .F., .F.,
 ( 4, 3, 3, 4 ),
 ( 0.000000000000000000, 0.0002476487219222810133, 0.0004952974148303670087, 0.0009534114850261750764 ),
 .UNSPECIFIED. ) ;
#22950=CARTESIAN_POINT ( 'NONE',  ( 109.9963952545248134, 0.8980012041604421569, -11.00651665394454071 ) ) ;
#22951=EDGE_CURVE ( 'NONE', #31774, #25264, #27242, .T. ) ;
#22953=DIRECTION ( 'NONE',  ( 0.000000000000000000, 0.000000000000000000, 1.000000000000000000 ) ) ;
#22963=( BOUNDED_CURVE ( )  B_SPLINE_CURVE ( 3, ( #44101, #34643, #12866, #26537 ),
 .UNSPECIFIED., .F., .F. ) 
 B_SPLINE_CURVE_WITH_KNOTS ( ( 4, 4 ),
 ( 4.712388980384689674, 6.283185307179590673 ),
 .UNSPECIFIED. ) 
 CURVE ( )  GEOMETRIC_REPRESENTATION_ITEM ( )  RATIONAL_B_SPLINE_CURVE ( ( 1.000000000000000000, 0.8047378541243649375, 0.8047378541243649375, 1.000000000000000000 ) ) 
 REPRESENTATION_ITEM ( '' )  );
#22976=CARTESIAN_POINT ( 'NONE',  ( 114.9970202545248412, 0.1403307496149616695, -11.32035403202665336 ) ) ;
#22981=CARTESIAN_POINT ( 'NONE',  ( 116.3166296295247832, -4.863998795839590272, -19.15521520033831493 ) ) ;
#22982=CARTESIAN_POINT ( 'NONE',  ( 109.4407702545248355, 0.1403307496149616695, -11.32035403202665336 ) ) ;
#22987=CARTESIAN_POINT ( 'NONE',  ( 115.4831921295247952, -9.868328341294093420, -13.39321520033831447 ) ) ;
#22994=CARTESIAN_POINT ( 'NONE',  ( 116.9101653964060858, -11.61644908211846605, -21.52136771687170480 ) ) ;
#23000=FACE_OUTER_BOUND ( 'NONE', #17572, .T. ) ;
#23002=CARTESIAN_POINT ( 'NONE',  ( 113.0523327545247838, -6.936859964151250502, -8.388885654883777576 ) ) ;
#23010=CARTESIAN_POINT ( 'NONE',  ( 70.36267391504962632, -5.685877709920933221, -4.893215200338314474 ) ) ;
#23034=CARTESIAN_POINT ( 'NONE',  ( 112.2188952545247531, 0.8980012041604421569, -11.00651665394454071 ) ) ;
#23035=CIRCLE ( 'NONE', #9939, 5.000000000000004441 ) ;
#23036=CARTESIAN_POINT ( 'NONE',  ( 107.9822546295247889, -4.863998795839590272, -18.39754474579285315 ) ) ;
#23037=CARTESIAN_POINT ( 'NONE',  ( 109.6491296295247793, -4.863998795839590272, -8.388885654883775800 ) ) ;
#23038=CARTESIAN_POINT ( 'NONE',  ( 109.5796765045248264, -7.250697342233347165, -19.15521520033832203 ) ) ;
#23042=CARTESIAN_POINT ( 'NONE',  ( 109.2294421295247275, -8.715624763370474426, -9.113786294776467400 ) ) ;
#23046=CARTESIAN_POINT ( 'NONE',  ( 107.5655358795247736, -8.402594152722688392, -9.854619843455216355 ) ) ;
#23049=CARTESIAN_POINT ( 'NONE',  ( 112.0105358795247810, -0.7896495226426338832, -17.46756447353520159 ) ) ;
#23061=ORIENTED_EDGE ( 'NONE', *, *, #36448, .F. ) ;
#23062=LINE ( 'NONE', #23754, #11797 ) ;
#23063=VECTOR ( 'NONE', #3049, 1000.000000000000000 ) ;
#23069=CARTESIAN_POINT ( 'NONE',  ( 111.1770983795247787, -0.7896495226426338832, -9.318865927141430916 ) ) ;
#23071=EDGE_CURVE ( 'NONE', #28016, #9382, #8776, .T. ) ;
#23082=CARTESIAN_POINT ( 'NONE',  ( 108.3295202545248657, -10.62599879583958717, -15.77991374673208469 ) ) ;
#23087=LINE ( 'NONE', #33321, #41513 ) ;
#23088=EDGE_LOOP ( 'NONE', ( #44058, #14991, #31441, #44469, #20780, #20218, #31635, #10118, #31397 ) ) ;
#23093=CARTESIAN_POINT ( 'NONE',  ( 113.6079577545248043, -7.250697342233347165, -7.631215200338321125 ) ) ;
#23094=CARTESIAN_POINT ( 'NONE',  ( 115.3442858795247759, -8.402594152722688392, -9.854619843455216355 ) ) ;
#23095=CARTESIAN_POINT ( 'NONE',  ( 110.7603796295247918, -4.863998795839590272, -19.15521520033831493 ) ) ;
#23098=ORIENTED_EDGE ( 'NONE', *, *, #34492, .F. ) ;
#23102=CARTESIAN_POINT ( 'NONE',  ( 108.3989733795248753, -8.938348069036489818, -17.46756447353520159 ) ) ;
#23110=VECTOR ( 'NONE', #9062, 1000.000000000000000 ) ;
#23115=CARTESIAN_POINT ( 'NONE',  ( 116.3166296295247832, -4.863998795839590272, -19.15521520033831493 ) ) ;
#23116=CARTESIAN_POINT ( 'NONE',  ( 112.9828796295247884, -4.863998795839590272, -8.388885654883775800 ) ) ;
#23119=CARTESIAN_POINT ( 'NONE',  ( 68.96620373265562876, -25.90251568920598757, -5.893215200338315363 ) ) ;
#23123=( GEOMETRIC_REPRESENTATION_CONTEXT ( 3 ) GLOBAL_UNCERTAINTY_ASSIGNED_CONTEXT ( ( #17726 ) ) GLOBAL_UNIT_ASSIGNED_CONTEXT ( ( #21341, #17475, #31598 ) ) REPRESENTATION_CONTEXT ( 'NONE', 'WORKASPACE' ) );
#23135=CARTESIAN_POINT ( 'NONE',  ( 108.0517077545248696, -7.250697342233347165, -7.631215200338321125 ) ) ;
#23140=CARTESIAN_POINT ( 'NONE',  ( 109.5102233795247884, -1.325403438956436419, -9.854619843455211026 ) ) ;
#23141=FACE_OUTER_BOUND ( 'NONE', #7598, .T. ) ;
#23151=CARTESIAN_POINT ( 'NONE',  ( 114.0977889883689897, 0.3193521225029610777, -12.14321520033831625 ) ) ;
#23154=VERTEX_POINT ( 'NONE', #6939 ) ;
#23157=CARTESIAN_POINT ( 'NONE',  ( 110.1353015045248469, -6.936859964151250502, -18.39754474579286025 ) ) ;
#23162=CARTESIAN_POINT ( 'NONE',  ( 112.9828796295247884, -4.863998795839590272, -8.388885654883775800 ) ) ;
#23168=CARTESIAN_POINT ( 'NONE',  ( 110.4131140045248287, -10.62599879583958717, -11.00651665394454604 ) ) ;
#23170=CARTESIAN_POINT ( 'NONE',  ( 114.3024890045248156, 0.8980012041604421569, -15.77991374673208469 ) ) ;
#23176=DIRECTION ( 'NONE',  ( 0.000000000000000000, 0.9284778069183717841, 0.3713878862591654673 ) ) ;
#23186=CARTESIAN_POINT ( 'NONE',  ( 108.6073327545248048, -2.477300249445798297, -19.15521520033831138 ) ) ;
#23188=CARTESIAN_POINT ( 'NONE',  ( 116.8211612789303473, -1.788438657886855632, -17.61956049856755158 ) ) ;
#23193=CARTESIAN_POINT ( 'NONE',  ( 112.9134265045247787, -2.791137627527939813, -8.388885654883754484 ) ) ;
#23198=CARTESIAN_POINT ( 'NONE',  ( 108.8851452545248151, -9.868328341294098749, -15.46607636864997204 ) ) ;
#23200=CARTESIAN_POINT ( 'NONE',  ( 78.75330084444993872, 4.432659906640606273, -21.58937828823235350 ) ) ;
#23209=CARTESIAN_POINT ( 'NONE',  ( 116.5249890045247980, -9.868328341294098749, -11.32035403202665869 ) ) ;
#23213=CARTESIAN_POINT ( 'NONE',  ( 106.2459265045248173, -2.791137627527939813, -8.388885654883777576 ) ) ;
#23214=CARTESIAN_POINT ( 'NONE',  ( 111.1770983795247787, -8.402594152722688392, -16.93181055722141792 ) ) ;
#23219=CARTESIAN_POINT ( 'NONE',  ( 113.2987212410415765, 0.7607806665037644134, -12.14321520033829493 ) ) ;
#23220=CARTESIAN_POINT ( 'NONE',  ( 111.8716296295247901, -4.863998795839590272, -8.388885654883775800 ) ) ;
#23227=CARTESIAN_POINT ( 'NONE',  ( 116.6117576306022841, -11.86965430100211805, -21.21901607071682605 ) ) ;
#23232=FACE_OUTER_BOUND ( 'NONE', #39602, .T. ) ;
#23233=FACE_OUTER_BOUND ( 'NONE', #37570, .T. ) ;
#23235=CARTESIAN_POINT ( 'NONE',  ( 110.2047546295247855, -4.863998795839590272, -18.39754474579285315 ) ) ;
#23243=LINE ( 'NONE', #23010, #14729 ) ;
#23248=CARTESIAN_POINT ( 'NONE',  ( 64.69189222814998175, -41.76310523276723785, -47.71602681600972318 ) ) ;
#23249=CARTESIAN_POINT ( 'NONE',  ( 77.92559343843963404, -57.44393871073324931, -1.136555471121397209 ) ) ;
#23265=CARTESIAN_POINT ( 'NONE',  ( 110.0658483795247804, -0.7896495226426338832, -9.318865927141430916 ) ) ;
#23266=CARTESIAN_POINT ( 'NONE',  ( 107.0099108795247815, -1.325403438956436419, -16.93181055722141792 ) ) ;
#23268=CARTESIAN_POINT ( 'NONE',  ( 64.58043734853313822, -37.66840613803912419, -5.037594184586155599 ) ) ;
#23274=CARTESIAN_POINT ( 'NONE',  ( 106.1764733795248219, -1.325403438956436419, -9.854619843455211026 ) ) ;
#23276=CARTESIAN_POINT ( 'NONE',  ( 105.9681140045248355, -10.62599879583958717, -11.00651665394454604 ) ) ;
#23277=CARTESIAN_POINT ( 'NONE',  ( 70.19189222814998175, -57.62004466406306591, -36.25082616574646721 ) ) ;
#23279=PLANE ( 'NONE',  #4100 ) ;
#23287=ORIENTED_EDGE ( 'NONE', *, *, #18088, .T. ) ;
#23295=CARTESIAN_POINT ( 'NONE',  ( 111.9410827545248708, -2.477300249445798297, -19.15521520033831138 ) ) ;
#23299=CIRCLE ( 'NONE', #29222, 8.000000000000000000 ) ;
#23306=CARTESIAN_POINT ( 'NONE',  ( 108.8156921295247912, 0.8980012041604618078, -13.39321520033831447 ) ) ;
#23312=ORIENTED_EDGE ( 'NONE', *, *, #30730, .F. ) ;
#23316=CARTESIAN_POINT ( 'NONE',  ( 114.2330358795247776, -0.7896495226426338832, -17.46756447353520159 ) ) ;
#23317=CARTESIAN_POINT ( 'NONE',  ( 114.9970202545248412, 0.1403307496149616695, -11.32035403202665336 ) ) ;
#23318=CARTESIAN_POINT ( 'NONE',  ( 110.6909265045248247, -7.250697342233347165, -19.15521520033831138 ) ) ;
#23330=CARTESIAN_POINT ( 'NONE',  ( 70.19189222814998175, -41.58126682492877535, -29.83537093841426469 ) ) ;
#23333=EDGE_LOOP ( 'NONE', ( #45033, #5254, #4758, #4422 ) ) ;
#23337=CARTESIAN_POINT ( 'NONE',  ( 108.1906140045248037, 0.1403307496149616695, -15.46607636864997204 ) ) ;
#23338=CARTESIAN_POINT ( 'NONE',  ( 111.1076452545248259, -9.868328341294098749, -15.46607636864997204 ) ) ;
#23341=CARTESIAN_POINT ( 'NONE',  ( 70.00926641990830035, -26.29760602141568526, -5.721420406450495655 ) ) ;
#23345=EDGE_CURVE ( 'NONE', #17886, #930, #3507, .T. ) ;
#23350=ORIENTED_EDGE ( 'NONE', *, *, #25920, .T. ) ;
#23357=CARTESIAN_POINT ( 'NONE',  ( 107.0793640045248196, -10.62599879583958717, -11.00651665394454604 ) ) ;
#23359=EDGE_CURVE ( 'NONE', #2225, #29882, #8056, .T. ) ;
#23363=CARTESIAN_POINT ( 'NONE',  ( 108.1906140045248037, 0.1403307496149616695, -15.46607636864997204 ) ) ;
#23364=AXIS2_PLACEMENT_3D ( 'NONE', #30233, #26816, #44830 ) ;
#23365=CARTESIAN_POINT ( 'NONE',  ( 70.19189222814998175, -49.76310523276723785, -36.33917278160906505 ) ) ;
#23371=CARTESIAN_POINT ( 'NONE',  ( 61.69189222814998175, -49.76310523276723785, -7.393215200338315363 ) ) ;
#23381=DIRECTION ( 'NONE',  ( -0.3445294493088594256, -0.9387755102040817867, 0.000000000000000000 ) ) ;
#23382=CARTESIAN_POINT ( 'NONE',  ( 109.2294421295247844, -1.388378309844742642, -16.99368411936019641 ) ) ;
#23383=CARTESIAN_POINT ( 'NONE',  ( 106.1070202545248407, 0.1403307496149616695, -11.32035403202665336 ) ) ;
#23387=CARTESIAN_POINT ( 'NONE',  ( 115.5526452545247622, -9.868328341294098749, -15.46607636864997204 ) ) ;
#23390=CARTESIAN_POINT ( 'NONE',  ( 113.7722331777918896, -0.01829820670813664396, -14.64321520033831447 ) ) ;
#23392=CARTESIAN_POINT ( 'NONE',  ( 110.1353015045248469, -2.477300249445798297, -7.631215200338321125 ) ) ;
#23394=CARTESIAN_POINT ( 'NONE',  ( 111.8716296295247901, -4.863998795839590272, -19.15521520033831493 ) ) ;
#23397=CARTESIAN_POINT ( 'NONE',  ( 112.0147320646196789, 0.6269505268395592079, -14.64321520033831447 ) ) ;
#23405=VECTOR ( 'NONE', #39657, 1000.000000000000114 ) ;
#23413=CARTESIAN_POINT ( 'NONE',  ( 109.9269421295247753, 0.8980012041604618078, -13.39321520033831447 ) ) ;
#23414=CARTESIAN_POINT ( 'NONE',  ( 109.6491296295247793, -4.863998795839590272, -8.388885654883775800 ) ) ;
#23420=DIRECTION ( 'NONE',  ( -1.000000000000000000, 1.091021054073464066E-15, 0.000000000000000000 ) ) ;
#23424=CARTESIAN_POINT ( 'NONE',  ( 78.69189222814998175, -69.76310523276724496, -16.89321520033831447 ) ) ;
#23425=CARTESIAN_POINT ( 'NONE',  ( 116.7079629495975155, 2.076812647898142572, -6.016578692477766666 ) ) ;
#23428=CARTESIAN_POINT ( 'NONE',  ( 106.3848327545248651, -6.936859964151250502, -8.388885654883777576 ) ) ;
#23431=AXIS2_PLACEMENT_3D ( 'NONE', #1604, #8914, #25568 ) ;
#23443=CARTESIAN_POINT ( 'NONE',  ( 110.8992858795247827, -0.7896495226426338832, -17.46756447353520159 ) ) ;
#23444=CARTESIAN_POINT ( 'NONE',  ( 107.4266296295248821, -4.863998795839590272, -8.388885654883775800 ) ) ;
#23445=CARTESIAN_POINT ( 'NONE',  ( 83.55688843573754809, -32.40901487178031459, -23.84144039813870464 ) ) ;
#23450=CARTESIAN_POINT ( 'NONE',  ( 113.8857702545248003, 0.1403307496149616695, -11.32035403202665336 ) ) ;
#23468=EDGE_CURVE ( 'NONE', #41318, #20584, #32436, .T. ) ;
#23469=CARTESIAN_POINT ( 'NONE',  ( 112.0105358795247810, -8.402594152722688392, -9.854619843455216355 ) ) ;
#23478=VERTEX_POINT ( 'NONE', #29472 ) ;
#23488=CARTESIAN_POINT ( 'NONE',  ( 113.1217858795247935, -8.402594152722688392, -9.854619843455216355 ) ) ;
#23500=CARTESIAN_POINT ( 'NONE',  ( 111.3854577545248645, -7.250697342233347165, -7.631215200338321125 ) ) ;
#23501=CARTESIAN_POINT ( 'NONE',  ( 106.0375671295248310, 0.1403307496149613920, -13.39321520033831447 ) ) ;
#23512=CARTESIAN_POINT ( 'NONE',  ( 115.9693640045247776, 0.1403307496149616695, -15.46607636864997204 ) ) ;
#23513=CARTESIAN_POINT ( 'NONE',  ( 78.69189222814998175, -69.76310523276724496, -16.89321520033831447 ) ) ;
#23514=VERTEX_POINT ( 'NONE', #32875 ) ;
#23521=( BOUNDED_SURFACE ( )  B_SPLINE_SURFACE ( 1, 2, ( 
 ( #39292, #35173, #4626, #31991, #15127, #38597, #32215, #35402, #29034, #988, #42944, #31769, #11036, #11261, #8285, #28590, #10812, #541, #24936, #38832, #7601, #18095, #14676, #25834, #40651, #16026, #29934, #26518, #2099, #8962, #12843, #5743, #9187, #5306, #23316, #40427, #39966, #36975, #43848, #19663, #16258, #12389, #2329, #23093, #29702, #8728, #33550, #30160, #5074, #12159, #40195, #43615, #22861, #15573, #9406, #15350, #29258, #36754, #36306, #26287, #39741, #12616, #36533, #5522, #8509, #19442, #33325, #11937, #44079, #26744, #37201, #18773, #32662, #1430, #43168, #43392, #22413, #18991, #32879, #1652, #19222, #29479, #26062, #22634, #33103, #1873, #15800, #30833, #2556, #10320, #30385, #44980, #6888, #13515, #20133, #13955, #41115, #10536, #16485, #41345, #23558, #44525, #34019, #6212, #2788, #13738, #3237, #37440, #24224, #27647, #34678, #13289, #41561, #34243, #13063, #16715, #6449, #30608, #33785, #10102, #24438, #5974, #19899, #27424, #41780, #24006, #27196, #9874, #23784, #38113, #40883, #20798, #20357, #17163, #26962, #37893, #37673, #3463, #6671, #17380, #9637, #3015, #16938, #31269, #44756, #42, #20579, #27867, #34458, #31051, #44308, #11438, #25115, #34889, #21690, #35117, #21909, #14172, #35803, #14853, #10761 ),
 ( #3678, #32388, #11654, #8001, #18498, #3899, #35576, #25343, #7319, #4573, #4349, #7782, #21240, #38329, #1157, #31936, #42892, #7105, #17818, #24884, #24658, #42445, #42220, #39012, #702, #14622, #15073, #41998, #31715, #35347, #10981, #11211, #28985, #17598, #18269, #28762, #31492, #7548, #32164, #21015, #484, #28539, #262, #28089, #42668, #933, #38544, #39237, #28308, #14397, #38778, #21464, #4122, #18041, #5693, #32828, #5250, #43111, #1378, #44023, #1598, #29201, #26233, #26012, #33047, #36482, #12333, #5023, #8231, #36923, #19167, #29878, #1821, #19388, #18939, #4799, #33277, #39916, #30107, #32611, #15293, #25560, #39467, #15975, #15518, #9132, #15749, #40142, #8678, #18720, #22138, #43794, #19612, #12109, #22581, #29650, #43564, #8906, #33496, #22361, #36030, #22805, #11881, #25784, #2051, #12559, #29425, #39692, #8457, #2274, #36256, #43339, #36700, #5468, #26465, #40369, #23036, #16204, #6393, #20301, #34625, #16431, #40830, #9819, #30551, #30779, #41508, #9356, #44704, #3186, #23266, #27139, #10050, #27595, #9585, #2960, #3412, #31218, #34405, #34186, #10264, #16887, #2732, #13465, #23501, #12785, #40598, #6159, #38062, #20078, #37620, #30329, #33733, #26688, #33964, #44255, #27367, #13237, #41289, #23729, #23954 ) ),
 .UNSPECIFIED., .F., .F., .T. ) 
 B_SPLINE_SURFACE_WITH_KNOTS ( ( 2, 2 ),
 ( 3, 2, 2, 2, 2, 2, 2, 2, 2, 2, 2, 2, 2, 2, 2, 2, 2, 2, 2, 2, 2, 2, 2, 2, 2, 2, 2, 2, 2, 2, 2, 2, 2, 2, 2, 2, 2, 2, 2, 2, 2, 2, 2, 2, 2, 2, 2, 2, 2, 2, 2, 2, 2, 2, 2, 2, 2, 2, 2, 2, 2, 2, 2, 2, 2, 2, 2, 2, 2, 2, 2, 2, 2, 2, 2, 2, 2, 2, 2, 2, 3 ),
 ( 0.000000000000000000, 1.000000000000000000 ),
 ( 0.000000000000000000, 0.01250000000000000069, 0.02500000000000000139, 0.03749999999999999861, 0.05000000000000000278, 0.06250000000000000000, 0.07499999999999999722, 0.08749999999999999445, 0.1000000000000000056, 0.1125000000000000028, 0.1250000000000000000, 0.1375000000000000111, 0.1499999999999999944, 0.1625000000000000056, 0.1749999999999999889, 0.1875000000000000000, 0.2000000000000000111, 0.2124999999999999944, 0.2250000000000000056, 0.2374999999999999889, 0.2500000000000000000, 0.2625000000000000111, 0.2750000000000000222, 0.2874999999999999778, 0.2999999999999999889, 0.3125000000000000000, 0.3250000000000000111, 0.3375000000000000222, 0.3499999999999999778, 0.3624999999999999889, 0.3750000000000000000, 0.3875000000000000111, 0.4000000000000000222, 0.4124999999999999778, 0.4249999999999999889, 0.4375000000000000000, 0.4500000000000000111, 0.4625000000000000222, 0.4749999999999999778, 0.4874999999999999889, 0.5000000000000000000, 0.5124999999999999556, 0.5250000000000000222, 0.5374999999999999778, 0.5500000000000000444, 0.5625000000000000000, 0.5749999999999999556, 0.5875000000000000222, 0.5999999999999999778, 0.6125000000000000444, 0.6250000000000000000, 0.6374999999999999556, 0.6500000000000000222, 0.6624999999999999778, 0.6750000000000000444, 0.6875000000000000000, 0.6999999999999999556, 0.7125000000000000222, 0.7249999999999999778, 0.7375000000000000444, 0.7500000000000000000, 0.7624999999999999556, 0.7750000000000000222, 0.7874999999999999778, 0.8000000000000000444, 0.8125000000000000000, 0.8249999999999999556, 0.8375000000000000222, 0.8499999999999999778, 0.8625000000000000444, 0.8750000000000000000, 0.8874999999999999556, 0.9000000000000000222, 0.9124999999999999778, 0.9250000000000000444, 0.9375000000000000000, 0.9499999999999999556, 0.9625000000000000222, 0.9749999999999999778, 0.9875000000000000444, 1.000000000000000000 ),
 .UNSPECIFIED. ) 
 GEOMETRIC_REPRESENTATION_ITEM ( )  RATIONAL_B_SPLINE_SURFACE ( (
 ( 1.000000000000000000, 0.9238795325112869605, 1.000000000000000000, 0.9238795325112869605, 1.000000000000000000, 0.9238795325112869605, 1.000000000000000000, 0.9238795325112869605, 1.000000000000000000, 0.9238795325112869605, 1.000000000000000000, 0.9238795325112869605, 1.000000000000000000, 0.9238795325112869605, 1.000000000000000000, 0.9238795325112869605, 1.000000000000000000, 0.9238795325112869605, 1.000000000000000000, 0.9238795325112869605, 1.000000000000000000, 0.9238795325112869605, 1.000000000000000000, 0.9238795325112869605, 1.000000000000000000, 0.9238795325112869605, 1.000000000000000000, 0.9238795325112869605, 1.000000000000000000, 0.9238795325112869605, 1.000000000000000000, 0.9238795325112869605, 1.000000000000000000, 0.9238795325112869605, 1.000000000000000000, 0.9238795325112869605, 1.000000000000000000, 0.9238795325112869605, 1.000000000000000000, 0.9238795325112869605, 1.000000000000000000, 0.9238795325112869605, 1.000000000000000000, 0.9238795325112869605, 1.000000000000000000, 0.9238795325112869605, 1.000000000000000000, 0.9238795325112869605, 1.000000000000000000, 0.9238795325112869605, 1.000000000000000000, 0.9238795325112869605, 1.000000000000000000, 0.9238795325112869605, 1.000000000000000000, 0.9238795325112869605, 1.000000000000000000, 0.9238795325112869605, 1.000000000000000000, 0.9238795325112869605, 1.000000000000000000, 0.9238795325112869605, 1.000000000000000000, 0.9238795325112869605, 1.000000000000000000, 0.9238795325112869605, 1.000000000000000000, 0.9238795325112869605, 1.000000000000000000, 0.9238795325112869605, 1.000000000000000000, 0.9238795325112869605, 1.000000000000000000, 0.9238795325112869605, 1.000000000000000000, 0.9238795325112869605, 1.000000000000000000, 0.9238795325112869605, 1.000000000000000000, 0.9238795325112869605, 1.000000000000000000, 0.9238795325112869605, 1.000000000000000000, 0.9238795325112869605, 1.000000000000000000, 0.9238795325112869605, 1.000000000000000000, 0.9238795325112869605, 1.000000000000000000, 0.9238795325112869605, 1.000000000000000000, 0.9238795325112869605, 1.000000000000000000, 0.9238795325112869605, 1.000000000000000000, 0.9238795325112869605, 1.000000000000000000, 0.9238795325112869605, 1.000000000000000000, 0.9238795325112869605, 1.000000000000000000, 0.9238795325112869605, 1.000000000000000000, 0.9238795325112869605, 1.000000000000000000, 0.9238795325112869605, 1.000000000000000000, 0.9238795325112869605, 1.000000000000000000, 0.9238795325112869605, 1.000000000000000000, 0.9238795325112869605, 1.000000000000000000, 0.9238795325112869605, 1.000000000000000000, 0.9238795325112869605, 1.000000000000000000, 0.9238795325112869605, 1.000000000000000000, 0.9238795325112869605, 1.000000000000000000, 0.9238795325112869605, 1.000000000000000000, 0.9238795325112869605, 1.000000000000000000, 0.9238795325112869605, 1.000000000000000000, 0.9238795325112869605, 1.000000000000000000, 0.9238795325112869605, 1.000000000000000000, 0.9238795325112869605, 1.000000000000000000, 0.9238795325112869605, 1.000000000000000000, 0.9238795325112869605, 1.000000000000000000, 0.9238795325112869605, 1.000000000000000000, 0.9238795325112869605, 1.000000000000000000, 0.9238795325112869605, 1.000000000000000000, 0.9238795325112869605, 1.000000000000000000, 0.9238795325112869605, 1.000000000000000000, 0.9238795325112869605, 1.000000000000000000, 0.9238795325112869605, 1.000000000000000000, 0.9238795325112869605, 1.000000000000000000, 0.9238795325112869605, 1.000000000000000000, 0.9238795325112869605, 1.000000000000000000, 0.9238795325112869605, 1.000000000000000000, 0.9238795325112869605, 1.000000000000000000),
 ( 1.000000000000000000, 0.9238795325112869605, 1.000000000000000000, 0.9238795325112869605, 1.000000000000000000, 0.9238795325112869605, 1.000000000000000000, 0.9238795325112869605, 1.000000000000000000, 0.9238795325112869605, 1.000000000000000000, 0.9238795325112869605, 1.000000000000000000, 0.9238795325112869605, 1.000000000000000000, 0.9238795325112869605, 1.000000000000000000, 0.9238795325112869605, 1.000000000000000000, 0.9238795325112869605, 1.000000000000000000, 0.9238795325112869605, 1.000000000000000000, 0.9238795325112869605, 1.000000000000000000, 0.9238795325112869605, 1.000000000000000000, 0.9238795325112869605, 1.000000000000000000, 0.9238795325112869605, 1.000000000000000000, 0.9238795325112869605, 1.000000000000000000, 0.9238795325112869605, 1.000000000000000000, 0.9238795325112869605, 1.000000000000000000, 0.9238795325112869605, 1.000000000000000000, 0.9238795325112869605, 1.000000000000000000, 0.9238795325112869605, 1.000000000000000000, 0.9238795325112869605, 1.000000000000000000, 0.9238795325112869605, 1.000000000000000000, 0.9238795325112869605, 1.000000000000000000, 0.9238795325112869605, 1.000000000000000000, 0.9238795325112869605, 1.000000000000000000, 0.9238795325112869605, 1.000000000000000000, 0.9238795325112869605, 1.000000000000000000, 0.9238795325112869605, 1.000000000000000000, 0.9238795325112869605, 1.000000000000000000, 0.9238795325112869605, 1.000000000000000000, 0.9238795325112869605, 1.000000000000000000, 0.9238795325112869605, 1.000000000000000000, 0.9238795325112869605, 1.000000000000000000, 0.9238795325112869605, 1.000000000000000000, 0.9238795325112869605, 1.000000000000000000, 0.9238795325112869605, 1.000000000000000000, 0.9238795325112869605, 1.000000000000000000, 0.9238795325112869605, 1.000000000000000000, 0.9238795325112869605, 1.000000000000000000, 0.9238795325112869605, 1.000000000000000000, 0.9238795325112869605, 1.000000000000000000, 0.9238795325112869605, 1.000000000000000000, 0.9238795325112869605, 1.000000000000000000, 0.9238795325112869605, 1.000000000000000000, 0.9238795325112869605, 1.000000000000000000, 0.9238795325112869605, 1.000000000000000000, 0.9238795325112869605, 1.000000000000000000, 0.9238795325112869605, 1.000000000000000000, 0.9238795325112869605, 1.000000000000000000, 0.9238795325112869605, 1.000000000000000000, 0.9238795325112869605, 1.000000000000000000, 0.9238795325112869605, 1.000000000000000000, 0.9238795325112869605, 1.000000000000000000, 0.9238795325112869605, 1.000000000000000000, 0.9238795325112869605, 1.000000000000000000, 0.9238795325112869605, 1.000000000000000000, 0.9238795325112869605, 1.000000000000000000, 0.9238795325112869605, 1.000000000000000000, 0.9238795325112869605, 1.000000000000000000, 0.9238795325112869605, 1.000000000000000000, 0.9238795325112869605, 1.000000000000000000, 0.9238795325112869605, 1.000000000000000000, 0.9238795325112869605, 1.000000000000000000, 0.9238795325112869605, 1.000000000000000000, 0.9238795325112869605, 1.000000000000000000, 0.9238795325112869605, 1.000000000000000000, 0.9238795325112869605, 1.000000000000000000, 0.9238795325112869605, 1.000000000000000000, 0.9238795325112869605, 1.000000000000000000, 0.9238795325112869605, 1.000000000000000000, 0.9238795325112869605, 1.000000000000000000, 0.9238795325112869605, 1.000000000000000000, 0.9238795325112869605, 1.000000000000000000, 0.9238795325112869605, 1.000000000000000000, 0.9238795325112869605, 1.000000000000000000, 0.9238795325112869605, 1.000000000000000000, 0.9238795325112869605, 1.000000000000000000, 0.9238795325112869605, 1.000000000000000000, 0.9238795325112869605, 1.000000000000000000) ) ) 
 REPRESENTATION_ITEM ( '' )  SURFACE ( )  );
#23536=CARTESIAN_POINT ( 'NONE',  ( 110.7603796295247918, -4.863998795839590272, -19.15521520033831493 ) ) ;
#23540=ORIENTED_EDGE ( 'NONE', *, *, #1337, .T. ) ;
#23542=EDGE_CURVE ( 'NONE', #13571, #40078, #33097, .T. ) ;
#23547=CARTESIAN_POINT ( 'NONE',  ( 108.4684265045247997, -7.250697342233347165, -19.15521520033831138 ) ) ;
#23558=CARTESIAN_POINT ( 'NONE',  ( 109.6491296295247793, -4.863998795839590272, -19.15521520033831493 ) ) ;
#23560=CARTESIAN_POINT ( 'NONE',  ( 111.8021765045248372, -2.791137627527939813, -8.388885654883777576 ) ) ;
#23561=CARTESIAN_POINT ( 'NONE',  ( 108.1906140045248463, -10.62599879583958717, -11.00651665394454604 ) ) ;
#23564=ORIENTED_EDGE ( 'NONE', *, *, #9005, .F. ) ;
#23572=DIRECTION ( 'NONE',  ( -0.9659258262890689783, -0.2588190451025185190, 0.000000000000000000 ) ) ;
#23578=CARTESIAN_POINT ( 'NONE',  ( 109.8574890045247940, -9.868328341294098749, -11.32035403202665869 ) ) ;
#23579=CARTESIAN_POINT ( 'NONE',  ( 112.2188952545247531, -9.868328341294098749, -15.46607636864997204 ) ) ;
#23598=CARTESIAN_POINT ( 'NONE',  ( 110.5520202545248054, 0.1403307496149616695, -11.32035403202665336 ) ) ;
#23608=CARTESIAN_POINT ( 'NONE',  ( 111.6852908578216983, 0.04929351793716424401, -12.14321520033834467 ) ) ;
#23609=DIRECTION ( 'NONE',  ( -1.000000000000000000, 0.000000000000000000, 0.000000000000000000 ) ) ;
#23616=CARTESIAN_POINT ( 'NONE',  ( 107.7044421295247929, -9.868328341294093420, -13.39321520033831447 ) ) ;
#23620=CARTESIAN_POINT ( 'NONE',  ( 115.6915515045247531, -6.936859964151250502, -18.39754474579286025 ) ) ;
#23621=CARTESIAN_POINT ( 'NONE',  ( 109.2296334740164809, -2.305094363982043593, -17.76548269841391203 ) ) ;
#23623=CARTESIAN_POINT ( 'NONE',  ( 108.8156921295247912, 0.8980012041604618078, -13.39321520033831447 ) ) ;
#23626=CARTESIAN_POINT ( 'NONE',  ( 113.5385046295247804, -4.863998795839590272, -7.631215200338315796 ) ) ;
#23643=CARTESIAN_POINT ( 'NONE',  ( 109.3713171295247832, 0.1403307496149613920, -13.39321520033831447 ) ) ;
#23645=CARTESIAN_POINT ( 'NONE',  ( 116.8582369479724719, -0.4338739127440741083, -16.23602533977254581 ) ) ;
#23646=CARTESIAN_POINT ( 'NONE',  ( 111.7327233795247849, -8.938348069036489818, -17.46756447353520159 ) ) ;
#23650=CARTESIAN_POINT ( 'NONE',  ( 112.8421051332721845, 0.2334052082820642360, -14.64321520033830026 ) ) ;
#23651=EDGE_CURVE ( 'NONE', #31450, #10427, #8281, .T. ) ;
#23656=CARTESIAN_POINT ( 'NONE',  ( 108.6767858795247861, -8.402594152722688392, -9.854619843455216355 ) ) ;
#23660=ADVANCED_FACE ( 'NONE', ( #39962, #28811 ), #25392, .T. ) ;
#23665=ORIENTED_EDGE ( 'NONE', *, *, #14501, .T. ) ;
#23672=CARTESIAN_POINT ( 'NONE',  ( 109.9963952545248134, 0.8980012041604421569, -11.00651665394454071 ) ) ;
#23673=CARTESIAN_POINT ( 'NONE',  ( 106.3153796295248412, -4.863998795839590272, -8.388885654883775800 ) ) ;
#23674=CARTESIAN_POINT ( 'NONE',  ( 83.25049447561245586, -31.94586068832097681, -23.46952294068349332 ) ) ;
#23679=CARTESIAN_POINT ( 'NONE',  ( 114.1635827545248389, -6.936859964151250502, -8.388885654883777576 ) ) ;
#23684=CARTESIAN_POINT ( 'NONE',  ( 79.39504145264901069, 5.044464786489276875, -6.294580001266408154 ) ) ;
#23687=EDGE_CURVE ( 'NONE', #21740, #25821, #23087, .T. ) ;
#23689=ORIENTED_EDGE ( 'NONE', *, *, #3274, .T. ) ;
#23690=CARTESIAN_POINT ( 'NONE',  ( 113.8163171295247764, -10.62599879583958540, -13.39321520033831803 ) ) ;
#23700=CARTESIAN_POINT ( 'NONE',  ( 109.3713171295247832, 0.1403307496149613920, -13.39321520033831447 ) ) ;
#23702=CARTESIAN_POINT ( 'NONE',  ( 83.82415148905927538, -46.76310523276723785, -23.89321520033831803 ) ) ;
#23707=AXIS2_PLACEMENT_3D ( 'NONE', #1753, #4952, #15677 ) ;
#23714=CARTESIAN_POINT ( 'NONE',  ( 74.19189222814998175, -41.76310523276723785, -4.893215200338314474 ) ) ;
#23728=CARTESIAN_POINT ( 'NONE',  ( 109.4407702545248355, -10.62599879583958717, -15.77991374673208469 ) ) ;
#23729=CARTESIAN_POINT ( 'NONE',  ( 104.9957702545248566, 0.1403307496149616695, -11.32035403202665336 ) ) ;
#23731=CARTESIAN_POINT ( 'NONE',  ( 109.8889130180080826, 0.7607806665037644134, -14.64321520033833757 ) ) ;
#23735=PLANE ( 'NONE',  #27791 ) ;
#23740=CARTESIAN_POINT ( 'NONE',  ( 115.6915515045247531, -6.936859964151250502, -18.39754474579286025 ) ) ;
#23742=ORIENTED_EDGE ( 'NONE', *, *, #6657, .F. ) ;
#23743=PLANE ( 'NONE',  #10697 ) ;
#23754=CARTESIAN_POINT ( 'NONE',  ( 85.70315449690899356, -26.74675748045603996, -18.39321520033831803 ) ) ;
#23757=VERTEX_POINT ( 'NONE', #43037 ) ;
#23761=CARTESIAN_POINT ( 'NONE',  ( 112.3578015045248861, -2.477300249445798297, -7.631215200338321125 ) ) ;
#23779=EDGE_CURVE ( 'NONE', #13698, #15215, #38404, .T. ) ;
#23784=CARTESIAN_POINT ( 'NONE',  ( 107.7044421295247929, 0.8980012041604618078, -13.39321520033831447 ) ) ;
#23785=CARTESIAN_POINT ( 'NONE',  ( 113.8857702545248003, 0.1403307496149616695, -11.32035403202665336 ) ) ;
#23786=CARTESIAN_POINT ( 'NONE',  ( 108.7462390045248242, 0.8980012041604421569, -15.77991374673208469 ) ) ;
#23799=CARTESIAN_POINT ( 'NONE',  ( 114.3024890045248156, -9.868328341294098749, -11.32035403202665869 ) ) ;
#23804=EDGE_CURVE ( 'NONE', #1801, #14918, #22064, .T. ) ;
#23806=CARTESIAN_POINT ( 'NONE',  ( 107.1488171295247867, 0.1403307496149613920, -13.39321520033831447 ) ) ;
#23807=CARTESIAN_POINT ( 'NONE',  ( 109.8574890045248509, -9.868328341294098749, -11.32035403202665869 ) ) ;
#23809=LINE ( 'NONE', #24627, #39030 ) ;
#23830=CARTESIAN_POINT ( 'NONE',  ( 115.3442858795247759, -0.7896495226426338832, -17.46756447353520159 ) ) ;
#23831=TOROIDAL_SURFACE ( 'NONE', #36904, 6.132259260909269649, 1.000000000000000000 ) ;
#23838=VECTOR ( 'NONE', #39591, 1000.000000000000000 ) ;
#23841=CARTESIAN_POINT ( 'NONE',  ( 66.04840902401572578, -36.51491089899629827, -5.214988841577086198 ) ) ;
#23847=CARTESIAN_POINT ( 'NONE',  ( 107.5655358795247736, -8.402594152722688392, -9.854619843455216355 ) ) ;
#23852=CARTESIAN_POINT ( 'NONE',  ( 114.0246765045248196, -2.791137627527939813, -8.388885654883777576 ) ) ;
#23857=CARTESIAN_POINT ( 'NONE',  ( 108.4684265045247997, -7.250697342233347165, -19.15521520033831138 ) ) ;
#23859=CARTESIAN_POINT ( 'NONE',  ( 113.6774108795247997, -8.938348069036489818, -9.318865927141430916 ) ) ;
#23862=CARTESIAN_POINT ( 'NONE',  ( 115.1359265045248321, -7.250697342233347165, -19.15521520033830427 ) ) ;
#23864=CARTESIAN_POINT ( 'NONE',  ( 70.19189222814998175, -84.91840466455968794, -47.17007500872661296 ) ) ;
#23865=ORIENTED_EDGE ( 'NONE', *, *, #23937, .T. ) ;
#23874=CARTESIAN_POINT ( 'NONE',  ( 106.5237390045248418, 0.8980012041604421569, -15.77991374673208469 ) ) ;
#23876=CARTESIAN_POINT ( 'NONE',  ( 116.8280838815325495, -1.500009456265160912, -17.40504711518565628 ) ) ;
#23877=CARTESIAN_POINT ( 'NONE',  ( 113.6774108795247997, -8.938348069036489818, -9.318865927141430916 ) ) ;
#23884=CARTESIAN_POINT ( 'NONE',  ( 116.3388580172722584, 2.269312398334672132, -6.503032629903105821 ) ) ;
#23886=CARTESIAN_POINT ( 'NONE',  ( 105.2735827545248810, -6.936859964151250502, -8.388885654883777576 ) ) ;
#23900=CARTESIAN_POINT ( 'NONE',  ( 109.2324108795247923, -8.938348069036489818, -9.318865927141430916 ) ) ;
#23901=CARTESIAN_POINT ( 'NONE',  ( 105.6208483795248299, -8.402594152722688392, -16.93181055722141792 ) ) ;
#23902=CARTESIAN_POINT ( 'NONE',  ( 115.6915515045247531, -2.477300249445798297, -7.631215200338321125 ) ) ;
#23907=CARTESIAN_POINT ( 'NONE',  ( 108.3989733795247759, -1.325403438956436419, -9.854619843455211026 ) ) ;
#23909=DIRECTION ( 'NONE',  ( 0.000000000000000000, 0.000000000000000000, -1.000000000000000000 ) ) ;
#23915=CARTESIAN_POINT ( 'NONE',  ( 113.8857702545248145, -10.62599879583958540, -15.77991374673209179 ) ) ;
#23917=ORIENTED_EDGE ( 'NONE', *, *, #34668, .F. ) ;
#23921=SURFACE_STYLE_FILL_AREA ( #2694 ) ;
#23926=CARTESIAN_POINT ( 'NONE',  ( 107.0793640045248196, 0.1403307496149616695, -15.46607636864997204 ) ) ;
#23927=TOROIDAL_SURFACE ( 'NONE', #10092, 1.500000000000000000, 0.5000000000000000000 ) ;
#23934=ORIENTED_EDGE ( 'NONE', *, *, #30046, .T. ) ;
#23937=EDGE_CURVE ( 'NONE', #13343, #6245, #26156, .T. ) ;
#23938=CARTESIAN_POINT ( 'NONE',  ( 78.10590893225656828, -57.76403841489356239, -0.8923062931455548741 ) ) ;
#23940=EDGE_CURVE ( 'NONE', #29903, #17270, #4503, .T. ) ;
#23953=CARTESIAN_POINT ( 'NONE',  ( 107.0793640045248196, -10.62599879583958717, -11.00651665394454604 ) ) ;
#23954=CARTESIAN_POINT ( 'NONE',  ( 104.9263171295248327, 0.1403307496149613920, -13.39321520033831447 ) ) ;
#23955=CARTESIAN_POINT ( 'NONE',  ( 72.75524511225664526, -29.99489077589588959, -12.39321520033834645 ) ) ;
#23961=DIRECTION ( 'NONE',  ( -1.000000000000000000, 1.156482317317869950E-15, 0.000000000000000000 ) ) ;
#23963=CARTESIAN_POINT ( 'NONE',  ( 106.7320983795247855, -0.7896495226426338832, -9.318865927141430916 ) ) ;
#23969=CARTESIAN_POINT ( 'NONE',  ( 82.89134431723762475, -31.13449359622123680, -21.94632144483577818 ) ) ;
#23974=ORIENTED_EDGE ( 'NONE', *, *, #36448, .T. ) ;
#23975=EDGE_CURVE ( 'NONE', #2531, #24941, #4727, .T. ) ;
#23984=CARTESIAN_POINT ( 'NONE',  ( 109.7185827545247889, -2.477300249445798297, -19.15521520033831138 ) ) ;
#23987=ORIENTED_EDGE ( 'NONE', *, *, #12196, .T. ) ;
#23995=DIRECTION ( 'NONE',  ( 0.000000000000000000, 0.000000000000000000, 1.000000000000000000 ) ) ;
#24000=EDGE_CURVE ( 'NONE', #34550, #19575, #43078, .T. ) ;
#24006=CARTESIAN_POINT ( 'NONE',  ( 107.9128015045248219, -2.477300249445798297, -7.631215200338321125 ) ) ;
#24007=CARTESIAN_POINT ( 'NONE',  ( 110.7603796295247918, -4.863998795839590272, -8.388885654883775800 ) ) ;
#24008=CARTESIAN_POINT ( 'NONE',  ( 106.8710046295248759, -4.863998795839590272, -7.631215200338315796 ) ) ;
#24013=CARTESIAN_POINT ( 'NONE',  ( 110.2742077545248094, -7.250697342233347165, -7.631215200338321125 ) ) ;
#24020=CARTESIAN_POINT ( 'NONE',  ( 114.9275671295247889, 0.1403307496149613920, -13.39321520033831447 ) ) ;
#24022=DIRECTION ( 'NONE',  ( 0.000000000000000000, -0.3713878862591650232, 0.9284778069183718952 ) ) ;
#24025=CARTESIAN_POINT ( 'NONE',  ( 109.7185827545247889, -6.936859964151250502, -8.388885654883777576 ) ) ;
#24026=CARTESIAN_POINT ( 'NONE',  ( 106.0375671295248310, 0.1403307496149613920, -13.39321520033831447 ) ) ;
#24035=ORIENTED_EDGE ( 'NONE', *, *, #10852, .T. ) ;
#24047=CARTESIAN_POINT ( 'NONE',  ( 106.6626452545248611, -9.868328341294098749, -15.46607636864997204 ) ) ;
#24050=DIRECTION ( 'NONE',  ( 0.000000000000000000, 1.000000000000000000, 0.000000000000000000 ) ) ;
#24058=CARTESIAN_POINT ( 'NONE',  ( 61.69189222814998175, -40.21211973637273474, -4.893215200338314474 ) ) ;
#24059=CARTESIAN_POINT ( 'NONE',  ( 116.5944421295247793, -4.863998795839590272, -8.393215200338314474 ) ) ;
#24066=DIRECTION ( 'NONE',  ( 0.000000000000000000, 0.000000000000000000, -1.000000000000000000 ) ) ;
#24067=CARTESIAN_POINT ( 'NONE',  ( 115.2748327545248657, -2.477300249445798297, -19.15521520033831138 ) ) ;
#24070=CARTESIAN_POINT ( 'NONE',  ( 110.7603796295247918, -4.863998795839590272, -8.388885654883775800 ) ) ;
#24074=CARTESIAN_POINT ( 'NONE',  ( 106.6626452545248611, 0.8980012041604421569, -11.00651665394454071 ) ) ;
#24075=CARTESIAN_POINT ( 'NONE',  ( 117.2294421295247844, -9.690077956319688823, -4.893215200338314474 ) ) ;
#24076=CARTESIAN_POINT ( 'NONE',  ( 108.2600671295247992, -10.62599879583958540, -13.39321520033831447 ) ) ;
#24079=CARTESIAN_POINT ( 'NONE',  ( 72.69189222814998175, -41.76310523276723785, -24.39321520033831447 ) ) ;
#24085=AXIS2_PLACEMENT_3D ( 'NONE', #17111, #6613, #31001 ) ;
#24090=CIRCLE ( 'NONE', #8061, 2.999999999999998224 ) ;
#24093=CARTESIAN_POINT ( 'NONE',  ( 116.8579880548923029, -0.4409650872748420158, -16.24658638300725499 ) ) ;
#24094=CARTESIAN_POINT ( 'NONE',  ( 115.6915515045247531, -2.477300249445798297, -7.631215200338321125 ) ) ;
#24095=VERTEX_POINT ( 'NONE', #34115 ) ;
#24099=CARTESIAN_POINT ( 'NONE',  ( 116.5944421295247793, -9.868328341294093420, -13.39321520033831447 ) ) ;
#24102=CARTESIAN_POINT ( 'NONE',  ( 116.3077641307500301, 2.279349991481241400, -6.542802709738571920 ) ) ;
#24104=CARTESIAN_POINT ( 'NONE',  ( 107.6349890045248401, -9.868328341294098749, -11.32035403202665869 ) ) ;
#24105=LINE ( 'NONE', #20902, #27331 ) ;
#24118=CARTESIAN_POINT ( 'NONE',  ( 109.4407702545248355, -10.62599879583958717, -15.77991374673208469 ) ) ;
#24119=CARTESIAN_POINT ( 'NONE',  ( 105.6903015045248253, -6.936859964151250502, -18.39754474579286025 ) ) ;
#24120=CARTESIAN_POINT ( 'NONE',  ( 82.78592324864024476, -31.79260405195279304, -23.13461678765773044 ) ) ;
#24126=CARTESIAN_POINT ( 'NONE',  ( 107.7738952545248310, -9.868328341294098749, -15.46607636864997204 ) ) ;
#24128=CARTESIAN_POINT ( 'NONE',  ( 65.19189222814998175, -41.76310523276723785, -4.893215200338314474 ) ) ;
#24142=CARTESIAN_POINT ( 'NONE',  ( 109.6491296295247793, -4.863998795839590272, -8.388885654883775800 ) ) ;
#24146=LINE ( 'NONE', #7241, #36652 ) ;
#24151=ORIENTED_EDGE ( 'NONE', *, *, #42337, .F. ) ;
#24152=CARTESIAN_POINT ( 'NONE',  ( 106.4542858795248179, -8.402594152722688392, -9.854619843455216355 ) ) ;
#24169=CARTESIAN_POINT ( 'NONE',  ( 109.3018640045248304, -10.62599879583958717, -11.00651665394454604 ) ) ;
#24171=LINE ( 'NONE', #23955, #44396 ) ;
#24172=CARTESIAN_POINT ( 'NONE',  ( 61.69189222814998175, -49.76310523276723785, -19.39321520033831447 ) ) ;
#24180=CARTESIAN_POINT ( 'NONE',  ( 111.8716296295247901, -4.863998795839590272, -8.388885654883775800 ) ) ;
#24189=EDGE_CURVE ( 'NONE', #38773, #37700, #16583, .T. ) ;
#24190=DIRECTION ( 'NONE',  ( 1.000000000000000000, 0.000000000000000000, 0.000000000000000000 ) ) ;
#24200=CARTESIAN_POINT ( 'NONE',  ( 61.69189222814998175, -57.16572941273946640, -4.036072343195455936 ) ) ;
#24202=CARTESIAN_POINT ( 'NONE',  ( 107.4960827545248350, -2.477300249445798297, -19.15521520033831138 ) ) ;
#24217=CARTESIAN_POINT ( 'NONE',  ( 69.87170781386352303, -25.28162009068048732, -5.721420406450495655 ) ) ;
#24224=CARTESIAN_POINT ( 'NONE',  ( 109.0935046295247872, -4.863998795839590272, -7.631215200338315796 ) ) ;
#24225=CARTESIAN_POINT ( 'NONE',  ( 108.1211608795247798, -1.325403438956436419, -16.93181055722141792 ) ) ;
#24226=CARTESIAN_POINT ( 'NONE',  ( 107.1488171295247867, -10.62599879583958540, -13.39321520033831447 ) ) ;
#24227=CARTESIAN_POINT ( 'NONE',  ( 79.79010115959992788, 5.106172230548759572, -19.89321520033831447 ) ) ;
#24231=CARTESIAN_POINT ( 'NONE',  ( 110.3436608795247764, -8.938348069036489818, -9.318865927141430916 ) ) ;
#24235=CARTESIAN_POINT ( 'NONE',  ( 70.19189222814998175, -65.04786711941002864, -39.22192925581976652 ) ) ;
#24238=CARTESIAN_POINT ( 'NONE',  ( 115.4137390045248566, -9.868328341294098749, -11.32035403202665869 ) ) ;
#24244=CARTESIAN_POINT ( 'NONE',  ( 115.3442858795247759, -0.7896495226426338832, -17.46756447353520159 ) ) ;
#24245=CARTESIAN_POINT ( 'NONE',  ( 106.3153796295248412, -4.863998795839590272, -8.388885654883775800 ) ) ;
#24260=ORIENTED_EDGE ( 'NONE', *, *, #21137, .T. ) ;
#24264=CARTESIAN_POINT ( 'NONE',  ( 69.69189222814998175, -41.76310523276723785, -6.393215200338315363 ) ) ;
#24267=CIRCLE ( 'NONE', #15529, 20.00000000000000355 ) ;
#24270=CARTESIAN_POINT ( 'NONE',  ( 106.5237390045248418, -9.868328341294098749, -11.32035403202665869 ) ) ;
#24271=VECTOR ( 'NONE', #6267, 1000.000000000000000 ) ;
#24277=DIRECTION ( 'NONE',  ( 0.000000000000000000, 0.000000000000000000, 1.000000000000000000 ) ) ;
#24280=CIRCLE ( 'NONE', #6067, 15.90000000000000036 ) ;
#24287=CARTESIAN_POINT ( 'NONE',  ( 107.0099108795247815, -1.325403438956436419, -16.93181055722141792 ) ) ;
#24292=CARTESIAN_POINT ( 'NONE',  ( 112.6609831777918913, -0.01829820670813664396, -14.64321520033831447 ) ) ;
#24293=CARTESIAN_POINT ( 'NONE',  ( 109.4407702545248355, 0.1403307496149616695, -11.32035403202665336 ) ) ;
#24294=CARTESIAN_POINT ( 'NONE',  ( 111.1770983795247787, -0.7896495226427380221, -9.318865927141420258 ) ) ;
#24295=CARTESIAN_POINT ( 'NONE',  ( 109.2294563837206312, -5.167320247529568533, -18.58757576157646696 ) ) ;
#24299=CARTESIAN_POINT ( 'NONE',  ( 110.2742077545248094, -7.250697342233347165, -7.631215200338321125 ) ) ;
#24318=CARTESIAN_POINT ( 'NONE',  ( 114.7886608795247696, -8.938348069036489818, -9.318865927141430916 ) ) ;
#24320=LINE ( 'NONE', #9738, #16240 ) ;
#24327=CARTESIAN_POINT ( 'NONE',  ( 74.19189222814998175, -41.76310523276723785, -24.39321520033831447 ) ) ;
#24328=CARTESIAN_POINT ( 'NONE',  ( 116.5249890045247980, -9.868328341294098749, -11.32035403202665869 ) ) ;
#24330=AXIS2_PLACEMENT_3D ( 'NONE', #3223, #31699, #24870 ) ;
#24338=CARTESIAN_POINT ( 'NONE',  ( 116.8028015045247940, -6.936859964151250502, -18.39754474579286025 ) ) ;
#24341=DIRECTION ( 'NONE',  ( 1.000000000000000000, 0.000000000000000000, 0.000000000000000000 ) ) ;
#24342=CARTESIAN_POINT ( 'NONE',  ( 112.0105358795247810, -0.7896495226426338832, -17.46756447353520159 ) ) ;
#24345=CARTESIAN_POINT ( 'NONE',  ( 109.2294627447761144, -0.4939093571603179744, -10.30950732205088016 ) ) ;
#24347=CARTESIAN_POINT ( 'NONE',  ( 107.4266296295248821, -4.863998795839590272, -8.388885654883775800 ) ) ;
#24350=CARTESIAN_POINT ( 'NONE',  ( 61.76986277844709861, -39.32091226840162079, -23.89321520033831803 ) ) ;
#24351=VERTEX_POINT ( 'NONE', #31146 ) ;
#24352=CARTESIAN_POINT ( 'NONE',  ( 61.69189222814998175, -49.76310523276723785, -19.39321520033831447 ) ) ;
#24357=B_SPLINE_CURVE_WITH_KNOTS ( 'NONE', 3,
 ( #9745, #3119, #44634, #6544, #41216, #34560, #2657, #141, #44404, #27524 ),
 .UNSPECIFIED., .F., .F.,
 ( 4, 3, 3, 4 ),
 ( 0.000000000000000000, 0.0002476487219222849707, 0.0004952974148303580099, 0.0009534114850261900384 ),
 .UNSPECIFIED. ) ;
#24361=CARTESIAN_POINT ( 'NONE',  ( 109.0240515045248202, -6.936859964151250502, -18.39754474579286025 ) ) ;
#24363=DIRECTION ( 'NONE',  ( 0.000000000000000000, 0.000000000000000000, 1.000000000000000000 ) ) ;
#24369=CARTESIAN_POINT ( 'NONE',  ( 106.5237390045248418, -9.868328341294098749, -11.32035403202665869 ) ) ;
#24371=EDGE_CURVE ( 'NONE', #13043, #5648, #17468, .T. ) ;
#24372=DIRECTION ( 'NONE',  ( 0.9387755102040818977, -0.3445294493088592036, 0.000000000000000000 ) ) ;
#24379=DIRECTION ( 'NONE',  ( 0.000000000000000000, 0.000000000000000000, 1.000000000000000000 ) ) ;
#24387=CARTESIAN_POINT ( 'NONE',  ( 109.1629577545248395, -7.250697342233347165, -7.631215200338321125 ) ) ;
#24389=CARTESIAN_POINT ( 'NONE',  ( 76.69189222814998175, -40.21211973637274184, -6.893215200338315363 ) ) ;
#24398=CARTESIAN_POINT ( 'NONE',  ( 113.1217858795247935, -8.402594152722688392, -9.854619843455216355 ) ) ;
#24407=CARTESIAN_POINT ( 'NONE',  ( 87.44708369096657918, -25.99489077589588604, -13.39321520033831447 ) ) ;
#24410=CARTESIAN_POINT ( 'NONE',  ( 116.5971529312752892, -9.866503804269289191, -13.43859147813565436 ) ) ;
#24418=CARTESIAN_POINT ( 'NONE',  ( 109.7880358795247986, -0.7896495226426338832, -17.46756447353520159 ) ) ;
#24426=CARTESIAN_POINT ( 'NONE',  ( 109.3272331777918822, -0.01829820670803256055, -14.64321520033831447 ) ) ;
#24433=DIRECTION ( 'NONE',  ( 0.000000000000000000, 1.000000000000000000, 0.000000000000000000 ) ) ;
#24435=EDGE_CURVE ( 'NONE', #16272, #816, #13826, .T. ) ;
#24438=CARTESIAN_POINT ( 'NONE',  ( 108.2600671295247992, -10.62599879583958540, -13.39321520033831447 ) ) ;
#24439=CARTESIAN_POINT ( 'NONE',  ( 106.8710046295248759, -4.863998795839590272, -18.39754474579285315 ) ) ;
#24440=CARTESIAN_POINT ( 'NONE',  ( 108.4684265045247997, -7.250697342233347165, -19.15521520033831138 ) ) ;
#24445=CARTESIAN_POINT ( 'NONE',  ( 110.6214733795247867, -8.938348069036489818, -17.46756447353520159 ) ) ;
#24452=CARTESIAN_POINT ( 'NONE',  ( 115.3442858795247759, -8.402594152722688392, -9.854619843455216355 ) ) ;
#24453=VERTEX_POINT ( 'NONE', #20897 ) ;
#24457=CARTESIAN_POINT ( 'NONE',  ( 113.7468640045248236, -10.62599879583958717, -11.00651665394454604 ) ) ;
#24458=CARTESIAN_POINT ( 'NONE',  ( 108.1906140045248463, 0.1403307496149616695, -15.46607636864997204 ) ) ;
#24463=ADVANCED_FACE ( 'NONE', ( #35218, #31588 ), #3338, .T. ) ;
#24471=EDGE_CURVE ( 'NONE', #40625, #21740, #42093, .T. ) ;
#24472=CARTESIAN_POINT ( 'NONE',  ( 109.1629577545248395, -2.791137627527939813, -18.39754474579286025 ) ) ;
#24476=CARTESIAN_POINT ( 'NONE',  ( 143.3676850761856940, -69.76310523276724496, -16.89321520033831447 ) ) ;
#24479=ORIENTED_EDGE ( 'NONE', *, *, #2876, .T. ) ;
#24480=ADVANCED_FACE ( 'NONE', ( #24537 ), #20049, .T. ) ;
#24483=CARTESIAN_POINT ( 'NONE',  ( 106.7320983795247855, -8.402594152722688392, -16.93181055722141792 ) ) ;
#24490=EDGE_CURVE ( 'NONE', #6307, #12500, #26506, .T. ) ;
#24493=CARTESIAN_POINT ( 'NONE',  ( 116.7341483858831737, -6.008534230275574650, -18.41440645892366490 ) ) ;
#24496=DIRECTION ( 'NONE',  ( 1.000000000000000000, 0.000000000000000000, 0.000000000000000000 ) ) ;
#24500=VERTEX_POINT ( 'NONE', #40415 ) ;
#24503=CARTESIAN_POINT ( 'NONE',  ( 111.0381921295247878, 0.8980012041604618078, -13.39321520033831447 ) ) ;
#24508=CARTESIAN_POINT ( 'NONE',  ( 111.6632702545248605, 0.1403307496149616695, -11.32035403202665336 ) ) ;
#24511=CARTESIAN_POINT ( 'NONE',  ( 109.2294418913466103, -8.121613810544367595, -17.63527159796440813 ) ) ;
#24513=CARTESIAN_POINT ( 'NONE',  ( 107.2877233795247776, -8.938348069036489818, -17.46756447353520159 ) ) ;
#24515=CARTESIAN_POINT ( 'NONE',  ( 107.7738952545248310, 0.8980012041604421569, -11.00651665394454071 ) ) ;
#24521=EDGE_LOOP ( 'NONE', ( #23865, #40365, #31411, #8974 ) ) ;
#24522=AXIS2_PLACEMENT_3D ( 'NONE', #35732, #41705, #24372 ) ;
#24533=CARTESIAN_POINT ( 'NONE',  ( 112.3578015045248861, -2.477300249445798297, -7.631215200338321125 ) ) ;
#24536=CIRCLE ( 'NONE', #31078, 20.00000000000000355 ) ;
#24537=FACE_OUTER_BOUND ( 'NONE', #28121, .T. ) ;
#24544=CARTESIAN_POINT ( 'NONE',  ( 117.0111608795247946, -1.325403438956436419, -16.93181055722141792 ) ) ;
#24556=CARTESIAN_POINT ( 'NONE',  ( 115.0664733795247798, -1.325403438956436419, -9.854619843455211026 ) ) ;
#24559=CARTESIAN_POINT ( 'NONE',  ( 86.21536009029834702, -26.71263513348336360, -8.458135821852174274 ) ) ;
#24560=CARTESIAN_POINT ( 'NONE',  ( 114.5803015045248117, -2.477300249445798297, -7.631215200338321125 ) ) ;
#24564=CARTESIAN_POINT ( 'NONE',  ( 109.2294415350724393, -1.058881497505862690, -9.579285122087750182 ) ) ;
#24567=CARTESIAN_POINT ( 'NONE',  ( 109.9963952545248134, -9.868328341294098749, -15.46607636864997204 ) ) ;
#24568=CARTESIAN_POINT ( 'NONE',  ( 117.1877300385866789, 1.365262974659312123, -21.54737627516459142 ) ) ;
#24571=CARTESIAN_POINT ( 'NONE',  ( 111.7327233795247849, -8.938348069036489818, -17.46756447353520159 ) ) ;
#24581=CARTESIAN_POINT ( 'NONE',  ( 107.9822546295247889, -4.863998795839590272, -18.39754474579285315 ) ) ;
#24583=FACE_BOUND ( 'NONE', #26117, .T. ) ;
#24590=CARTESIAN_POINT ( 'NONE',  ( 106.8015515045248378, -6.936859964151250502, -18.39754474579286025 ) ) ;
#24595=CARTESIAN_POINT ( 'NONE',  ( 83.82415148905927538, -46.76310523276723785, -4.893215200338314474 ) ) ;
#24600=CARTESIAN_POINT ( 'NONE',  ( 116.8928740015602870, 0.2848729546123598966, -14.64321520033831447 ) ) ;
#24608=CARTESIAN_POINT ( 'NONE',  ( 108.3295202545248657, -10.62599879583958717, -15.77991374673208469 ) ) ;
#24610=DIRECTION ( 'NONE',  ( -1.000000000000000000, 0.000000000000000000, 0.000000000000000000 ) ) ;
#24611=CARTESIAN_POINT ( 'NONE',  ( 113.3470697905468825, 0.6938714319018670640, -12.14321520033833579 ) ) ;
#24614=DIRECTION ( 'NONE',  ( 0.000000000000000000, -0.3713878862591641905, 0.9284778069183722282 ) ) ;
#24619=CARTESIAN_POINT ( 'NONE',  ( 112.2188952545247531, -9.868328341294098749, -15.46607636864997204 ) ) ;
#24626=CARTESIAN_POINT ( 'NONE',  ( 109.2294421295247844, 0.8460904216231607267, -19.39321520033831447 ) ) ;
#24627=CARTESIAN_POINT ( 'NONE',  ( 61.43583762032555029, 4.505738898882963639, -14.64321520033831447 ) ) ;
#24634=CARTESIAN_POINT ( 'NONE',  ( 116.5982304348999889, -9.866848165334292986, -13.49403011250934625 ) ) ;
#24640=CARTESIAN_POINT ( 'NONE',  ( 107.2182702545248105, -10.62599879583958717, -15.77991374673208469 ) ) ;
#24642=EDGE_LOOP ( 'NONE', ( #41940, #25623, #19125, #20970 ) ) ;
#24643=ORIENTED_EDGE ( 'NONE', *, *, #25029, .F. ) ;
#24646=CARTESIAN_POINT ( 'NONE',  ( 79.25282380889900935, 4.987561187848681854, -20.71017453681549725 ) ) ;
#24650=DIRECTION ( 'NONE',  ( -1.000000000000000000, 1.156482317317869950E-15, 0.000000000000000000 ) ) ;
#24658=CARTESIAN_POINT ( 'NONE',  ( 114.6497546295247929, -4.863998795839590272, -18.39754474579285315 ) ) ;
#24659=CARTESIAN_POINT ( 'NONE',  ( 107.7044421295247929, -9.868328341294093420, -13.39321520033831447 ) ) ;
#24660=CARTESIAN_POINT ( 'NONE',  ( 113.0523327545247838, -6.936859964151250502, -8.388885654883777576 ) ) ;
#24663=ORIENTED_EDGE ( 'NONE', *, *, #22011, .F. ) ;
#24665=CARTESIAN_POINT ( 'NONE',  ( 112.8439733795247832, -8.938348069036489818, -17.46756447353520159 ) ) ;
#24666=CARTESIAN_POINT ( 'NONE',  ( 66.82415148905926117, -30.76310523276723785, -21.89321520033831447 ) ) ;
#24671=CARTESIAN_POINT ( 'NONE',  ( 112.9134265045247645, -7.250697342233347165, -19.15521520033831138 ) ) ;
#24672=CARTESIAN_POINT ( 'NONE',  ( 106.6626452545248611, 0.8980012041604421569, -11.00651665394454071 ) ) ;
#24677=CARTESIAN_POINT ( 'NONE',  ( 115.6220983795247861, -0.7896495226426338832, -9.318865927141430916 ) ) ;
#24678=CARTESIAN_POINT ( 'NONE',  ( 105.4819421295248247, -9.868328341294093420, -13.39321520033831447 ) ) ;
#24680=UNCERTAINTY_MEASURE_WITH_UNIT (LENGTH_MEASURE( 1.000000000000000082E-05 ), #30518, 'distance_accuracy_value', 'NONE');
#24689=CARTESIAN_POINT ( 'NONE',  ( 106.0375671295248310, -10.62599879583958540, -13.39321520033831447 ) ) ;
#24690=CARTESIAN_POINT ( 'NONE',  ( 112.8439733795247832, -1.325403438956436419, -9.854619843455211026 ) ) ;
#24697=VERTEX_POINT ( 'NONE', #41767 ) ;
#24700=CARTESIAN_POINT ( 'NONE',  ( 116.5249890045247980, 0.8980012041604421569, -15.77991374673208469 ) ) ;
#24707=FACE_OUTER_BOUND ( 'NONE', #3073, .T. ) ;
#24708=CARTESIAN_POINT ( 'NONE',  ( 84.90318689630748850, -29.89078148095193654, -11.34622365899691943 ) ) ;
#24715=CARTESIAN_POINT ( 'NONE',  ( 85.75809888461174069, -18.45227461768569199, -19.39321520033831447 ) ) ;
#24716=CARTESIAN_POINT ( 'NONE',  ( 111.1076452545248259, 0.8980012041604421569, -11.00651665394454071 ) ) ;
#24720=EDGE_CURVE ( 'NONE', #38298, #40576, #14312, .T. ) ;
#24722=CARTESIAN_POINT ( 'NONE',  ( 107.9822546295247889, -4.863998795839590272, -18.39754474579285315 ) ) ;
#24724=CARTESIAN_POINT ( 'NONE',  ( 112.0105358795247810, -0.7896495226426338832, -17.46756447353520159 ) ) ;
#24725=CARTESIAN_POINT ( 'NONE',  ( 109.2296352495891796, -8.786749211135761684, -17.08468090821677166 ) ) ;
#24727=CARTESIAN_POINT ( 'NONE',  ( 107.1488171295247867, -10.62599879583958540, -13.39321520033831447 ) ) ;
#24728=CARTESIAN_POINT ( 'NONE',  ( 116.6638952545248031, -9.868328341294098749, -15.46607636864997204 ) ) ;
#24729=CARTESIAN_POINT ( 'NONE',  ( 109.1629577545248395, -7.250697342233347165, -7.631215200338321125 ) ) ;
#24732=DIRECTION ( 'NONE',  ( -1.000000000000000000, 0.000000000000000000, 0.000000000000000000 ) ) ;
#24735=EDGE_LOOP ( 'NONE', ( #13598, #23689, #44434, #28282 ) ) ;
#24741=EDGE_CURVE ( 'NONE', #23514, #27457, #40820, .T. ) ;
#24744=EDGE_CURVE ( 'NONE', #29882, #38699, #10751, .T. ) ;
#24748=CARTESIAN_POINT ( 'NONE',  ( 108.9545983795247821, -0.7896495226426338832, -9.318865927141430916 ) ) ;
#24751=CARTESIAN_POINT ( 'NONE',  ( 116.8028015045247940, -6.936859964151250502, -18.39754474579286025 ) ) ;
#24756=CARTESIAN_POINT ( 'NONE',  ( 111.5473838361194794, 0.1075849324168598464, -12.14321520033829671 ) ) ;
#24758=CARTESIAN_POINT ( 'NONE',  ( 116.9417077545247992, -2.791137627527939813, -18.39754474579286025 ) ) ;
#24764=PLANE ( 'NONE',  #11830 ) ;
#24769=CARTESIAN_POINT ( 'NONE',  ( 114.3719421295247827, -9.868328341294093420, -13.39321520033831447 ) ) ;
#24775=CARTESIAN_POINT ( 'NONE',  ( 111.7327233795247849, -8.938348069036489818, -17.46756447353520159 ) ) ;
#24780=CARTESIAN_POINT ( 'NONE',  ( 109.2294428007942741, -3.526316717755844987, -8.039392986164429544 ) ) ;
#24782=CARTESIAN_POINT ( 'NONE',  ( 109.8574890045247940, -9.868328341294098749, -11.32035403202665869 ) ) ;
#24784=CYLINDRICAL_SURFACE ( 'NONE', #6575, 4.500000000000003553 ) ;
#24787=CARTESIAN_POINT ( 'NONE',  ( 109.9963952545248134, 0.8980012041604421569, -11.00651665394454071 ) ) ;
#24800=CARTESIAN_POINT ( 'NONE',  ( 115.7610046295247912, -4.863998795839590272, -7.631215200338315796 ) ) ;
#24802=CARTESIAN_POINT ( 'NONE',  ( 116.0286950891469786, 2.331313199634366118, -4.893215200338314474 ) ) ;
#24808=CARTESIAN_POINT ( 'NONE',  ( 115.8304577545247582, -7.250697342233347165, -7.631215200338321125 ) ) ;
#24817=CIRCLE ( 'NONE', #5870, 5.000000000000004441 ) ;
#24820=CIRCLE ( 'NONE', #43746, 5.132259260909280307 ) ;
#24828=CARTESIAN_POINT ( 'NONE',  ( 113.4690515045247992, -6.936859964151250502, -18.39754474579286025 ) ) ;
#24838=EDGE_CURVE ( 'NONE', #38575, #11904, #41104, .T. ) ;
#24840=CARTESIAN_POINT ( 'NONE',  ( 110.8992858795247827, -8.402594152722688392, -9.854619843455216355 ) ) ;
#24852=DIRECTION ( 'NONE',  ( 0.000000000000000000, 0.000000000000000000, -1.000000000000000000 ) ) ;
#24854=EDGE_LOOP ( 'NONE', ( #229, #4554, #12368, #2253 ) ) ;
#24855=DIRECTION ( 'NONE',  ( 0.000000000000000000, 0.000000000000000000, -1.000000000000000000 ) ) ;
#24856=AXIS2_PLACEMENT_3D ( 'NONE', #11513, #1894, #18570 ) ;
#24860=B_SPLINE_SURFACE_WITH_KNOTS ( 'NONE', 3, 3, ( 
 ( #36892, #29164, #5662, #29394, #43305, #16171, #19581, #33462, #12074, #25978 ),
 ( #5999, #5097, #22881, #19012, #39986, #40676, #26767, #15597, #26310, #36775 ),
 ( #19243, #19922, #33808, #16509, #5327, #5546, #1674, #33575, #8983, #32898 ),
 ( #36553, #29500, #2350, #2579, #43414, #19463, #12181, #8752, #9428, #23341 ),
 ( #40218, #33346, #2120, #33126, #30408, #11958, #25856, #1895, #16049, #26082 ),
 ( #29955, #22657, #43870, #39762, #9210, #12642, #15823, #29722, #37225, #43636 ),
 ( #8532, #26538, #12410, #40448, #23119, #36996, #5767, #22434, #19688, #36327 ),
 ( #16282, #30184, #44102, #12867, #3643, #25077, #42409, #37697, #9661, #11173 ) ),
 .UNSPECIFIED., .F., .F., .F.,
 ( 4, 2, 2, 4 ),
 ( 4, 2, 2, 2, 4 ),
 ( 0.000000000000000000, 0.5000000000000000000, 0.7500000000000000000, 1.000000000000000000 ),
 ( 0.000000000000000000, 0.2500000000000000000, 0.5000000000000000000, 0.7500000000000000000, 1.000000000000000000 ),
 .UNSPECIFIED. ) ;
#24862=FACE_OUTER_BOUND ( 'NONE', #26663, .T. ) ;
#24864=CARTESIAN_POINT ( 'NONE',  ( 109.9963952545248134, 0.8980012041604421569, -11.00651665394454071 ) ) ;
#24866=VERTEX_POINT ( 'NONE', #17152 ) ;
#24870=DIRECTION ( 'NONE',  ( -1.000000000000000000, 0.000000000000000000, 0.000000000000000000 ) ) ;
#24882=CARTESIAN_POINT ( 'NONE',  ( 112.2395221536727377, 0.3967854368540359999, -10.50530088663809636 ) ) ;
#24883=CARTESIAN_POINT ( 'NONE',  ( 114.1635827545248389, -2.477300249445798297, -19.15521520033831138 ) ) ;
#24884=CARTESIAN_POINT ( 'NONE',  ( 114.7192077545248594, -2.791137627527939813, -18.39754474579286025 ) ) ;
#24886=CARTESIAN_POINT ( 'NONE',  ( 110.3436608795247764, -1.325403438956436419, -16.93181055722141792 ) ) ;
#24887=CARTESIAN_POINT ( 'NONE',  ( 113.1912390045248031, -9.868328341294098749, -11.32035403202665869 ) ) ;
#24890=ORIENTED_EDGE ( 'NONE', *, *, #14485, .T. ) ;
#24892=CARTESIAN_POINT ( 'NONE',  ( 109.9963952545248134, 0.8980012041604421569, -11.00651665394454071 ) ) ;
#24896=CARTESIAN_POINT ( 'NONE',  ( 79.31152370492512205, 5.005448908239999994, -6.165396227893437775 ) ) ;
#24898=CARTESIAN_POINT ( 'NONE',  ( 114.4413952545248350, 0.8980012041604421569, -11.00651665394454071 ) ) ;
#24899=CARTESIAN_POINT ( 'NONE',  ( 111.5243640045248412, 0.1403307496149616695, -15.46607636864997204 ) ) ;
#24908=ORIENTED_EDGE ( 'NONE', *, *, #18083, .T. ) ;
#24916=CARTESIAN_POINT ( 'NONE',  ( 106.6626452545248611, 0.8980012041604421569, -11.00651665394454071 ) ) ;
#24917=CARTESIAN_POINT ( 'NONE',  ( 112.7050671295247923, 0.1403307496149613920, -13.39321520033831447 ) ) ;
#24920=EDGE_LOOP ( 'NONE', ( #30776, #8602, #6015, #22164 ) ) ;
#24928=CARTESIAN_POINT ( 'NONE',  ( 109.0240515045248202, -2.477300249445798297, -7.631215200338321125 ) ) ;
#24929=CARTESIAN_POINT ( 'NONE',  ( 117.1373561229423217, -11.24370064073201902, -21.77221270345598825 ) ) ;
#24933=ORIENTED_EDGE ( 'NONE', *, *, #17248, .T. ) ;
#24936=CARTESIAN_POINT ( 'NONE',  ( 115.3442858795247759, -0.7896495226426338832, -17.46756447353520159 ) ) ;
#24941=VERTEX_POINT ( 'NONE', #18256 ) ;
#24944=CARTESIAN_POINT ( 'NONE',  ( 111.3854577545248645, -7.250697342233347165, -7.631215200338321125 ) ) ;
#24949=CARTESIAN_POINT ( 'NONE',  ( 111.6379010812576809, -0.01829820670803256055, -12.14321520033831625 ) ) ;
#24950=CARTESIAN_POINT ( 'NONE',  ( 111.9410827545248708, -6.936859964151250502, -8.388885654883777576 ) ) ;
#24951=EDGE_LOOP ( 'NONE', ( #14483, #13622, #43282 ) ) ;
#24954=CARTESIAN_POINT ( 'NONE',  ( 109.2294425607255164, -3.087680864912572432, -18.17836862529099307 ) ) ;
#24958=CARTESIAN_POINT ( 'NONE',  ( 107.4960827545248350, -2.477300249445798297, -19.15521520033831138 ) ) ;
#24959=LINE ( 'NONE', #38618, #14532 ) ;
#24972=AXIS2_PLACEMENT_3D ( 'NONE', #44820, #44595, #20423 ) ;
#24975=CARTESIAN_POINT ( 'NONE',  ( 110.4825671295247815, -10.62599879583958540, -13.39321520033831447 ) ) ;
#24978=CARTESIAN_POINT ( 'NONE',  ( 115.8304577545247582, -2.791137627527939813, -18.39754474579286025 ) ) ;
#24981=CARTESIAN_POINT ( 'NONE',  ( 117.2294421295247986, 1.224656517226988761, -5.142251848794600733 ) ) ;
#24983=CARTESIAN_POINT ( 'NONE',  ( 111.3178276191212888, 0.4261359969230590905, -12.14321520033830026 ) ) ;
#24985=CARTESIAN_POINT ( 'NONE',  ( 114.1635827545248389, -6.936859964151250502, -8.388885654883777576 ) ) ;
#24995=DIRECTION ( 'NONE',  ( -0.6383198453882299450, -0.7697712484781087383, -9.200178928217186715E-17 ) ) ;
#24997=CARTESIAN_POINT ( 'NONE',  ( 116.0388171295248014, 0.1403307496149613920, -13.39321520033831447 ) ) ;
#24999=VECTOR ( 'NONE', #18628, 1000.000000000000000 ) ;
#25002=CARTESIAN_POINT ( 'NONE',  ( 113.8163171295247764, -10.62599879583958540, -13.39321520033831447 ) ) ;
#25006=CARTESIAN_POINT ( 'NONE',  ( 109.2295803840910509, -1.953966997837194963, -8.791361225266440371 ) ) ;
#25008=CARTESIAN_POINT ( 'NONE',  ( 113.4690515045247992, -2.477300249445798297, -7.631215200338321125 ) ) ;
#25010=CARTESIAN_POINT ( 'NONE',  ( 116.4462812948059707, 2.227954574770207863, -20.42202840589934709 ) ) ;
#25013=CARTESIAN_POINT ( 'NONE',  ( 112.5661608795247872, -8.938348069036489818, -9.318865927141430916 ) ) ;
#25024=CARTESIAN_POINT ( 'NONE',  ( 112.4967077545247633, -7.250697342233347165, -7.631215200338321125 ) ) ;
#25027=ORIENTED_EDGE ( 'NONE', *, *, #14710, .F. ) ;
#25029=EDGE_CURVE ( 'NONE', #13571, #27865, #4335, .T. ) ;
#25030=VECTOR ( 'NONE', #7280, 1000.000000000000000 ) ;
#25032=ADVANCED_FACE ( 'NONE', ( #14839 ), #758, .F. ) ;
#25034=ORIENTED_EDGE ( 'NONE', *, *, #5771, .T. ) ;
#25035=CARTESIAN_POINT ( 'NONE',  ( 106.1070202545248407, 0.1403307496149616695, -11.32035403202665336 ) ) ;
#25039=CARTESIAN_POINT ( 'NONE',  ( 65.96249443994719286, -37.38467533475423465, -4.893215200338314474 ) ) ;
#25040=CARTESIAN_POINT ( 'NONE',  ( 64.35098164443778046, -35.92212675331819582, -5.786495942213375265 ) ) ;
#25056=ORIENTED_EDGE ( 'NONE', *, *, #13941, .F. ) ;
#25058=CARTESIAN_POINT ( 'NONE',  ( 115.8304577545247582, -2.791137627527939813, -18.39754474579286025 ) ) ;
#25069=VECTOR ( 'NONE', #34877, 1000.000000000000000 ) ;
#25070=CARTESIAN_POINT ( 'NONE',  ( 113.8857702545248003, 0.1403307496149616695, -11.32035403202665336 ) ) ;
#25077=CARTESIAN_POINT ( 'NONE',  ( 68.68839935636917460, -25.95913848132418522, -5.893215200338315363 ) ) ;
#25081=CARTESIAN_POINT ( 'NONE',  ( 62.78176453955970970, -64.70373736148800958, -45.96606927953587984 ) ) ;
#25102=LINE ( 'NONE', #36019, #5842 ) ;
#25103=DIRECTION ( 'NONE',  ( 0.000000000000000000, 0.000000000000000000, 1.000000000000000000 ) ) ;
#25111=EDGE_CURVE ( 'NONE', #22322, #13343, #25102, .T. ) ;
#25114=CARTESIAN_POINT ( 'NONE',  ( 116.5249890045247980, 0.8980012041604421569, -15.77991374673208469 ) ) ;
#25115=CARTESIAN_POINT ( 'NONE',  ( 106.0375671295248310, -10.62599879583958540, -13.39321520033831447 ) ) ;
#25116=CARTESIAN_POINT ( 'NONE',  ( 112.9134265045247645, -2.791137627527939813, -8.388885654883777576 ) ) ;
#25122=CARTESIAN_POINT ( 'NONE',  ( 107.0793640045248196, -10.62599879583958717, -11.00651665394454604 ) ) ;
#25123=PLANE ( 'NONE',  #16134 ) ;
#25129=CARTESIAN_POINT ( 'NONE',  ( 113.2606921295247702, 0.8980012041604618078, -13.39321520033831447 ) ) ;
#25130=CARTESIAN_POINT ( 'NONE',  ( 110.3436608795247764, -1.325403438956436419, -16.93181055722141792 ) ) ;
#25133=CARTESIAN_POINT ( 'NONE',  ( 116.0286950891469786, 2.331313199634366118, -4.893215200338314474 ) ) ;
#25148=CARTESIAN_POINT ( 'NONE',  ( 105.8986608795248401, -8.938348069036489818, -9.318865927141430916 ) ) ;
#25149=CARTESIAN_POINT ( 'NONE',  ( 115.1359265045248605, -7.250697342233347165, -19.15521520033831138 ) ) ;
#25151=ORIENTED_EDGE ( 'NONE', *, *, #8956, .F. ) ;
#25155=CYLINDRICAL_SURFACE ( 'NONE', #38910, 4.500000000000003553 ) ;
#25161=CARTESIAN_POINT ( 'NONE',  ( 110.8992858795247827, -0.7896495226426338832, -17.46756447353520159 ) ) ;
#25162=CARTESIAN_POINT ( 'NONE',  ( 117.1361595269186040, -11.24668708007285289, -21.77080567551499968 ) ) ;
#25165=DIRECTION ( 'NONE',  ( 0.000000000000000000, 0.000000000000000000, -1.000000000000000000 ) ) ;
#25169=CARTESIAN_POINT ( 'NONE',  ( 84.86020291624612355, -29.99489077589588959, -12.39321520033831447 ) ) ;
#25170=CARTESIAN_POINT ( 'NONE',  ( 116.8057029421682813, 0.1954196160062621201, -12.14321520033831625 ) ) ;
#25171=ADVANCED_FACE ( 'NONE', ( #31702 ), #31925, .T. ) ;
#25176=CARTESIAN_POINT ( 'NONE',  ( 109.7185827545247889, -2.477300249445798297, -19.15521520033831138 ) ) ;
#25180=CARTESIAN_POINT ( 'NONE',  ( 112.1494421295248003, -9.868328341294093420, -13.39321520033836421 ) ) ;
#25184=CARTESIAN_POINT ( 'NONE',  ( 109.2294421286841697, -3.110521482657592873, -18.18806147283417474 ) ) ;
#25188=CARTESIAN_POINT ( 'NONE',  ( 115.4137390045248566, -9.868328341294098749, -11.32035403202665869 ) ) ;
#25189=CARTESIAN_POINT ( 'NONE',  ( 107.1488171295247867, -10.62599879583958540, -13.39321520033831447 ) ) ;
#25192=LINE ( 'NONE', #20873, #14602 ) ;
#25206=CARTESIAN_POINT ( 'NONE',  ( 108.8156921295247912, 0.8980012041604618078, -13.39321520033831447 ) ) ;
#25209=CARTESIAN_POINT ( 'NONE',  ( 111.9410827545248708, -6.936859964151250502, -8.388885654883777576 ) ) ;
#25215=CARTESIAN_POINT ( 'NONE',  ( 112.4272546295247821, -4.863998795839590272, -18.39754474579285315 ) ) ;
#25228=CARTESIAN_POINT ( 'NONE',  ( 116.1777233795247781, -1.325403438956436419, -9.854619843455211026 ) ) ;
#25232=CARTESIAN_POINT ( 'NONE',  ( 85.91347875220176888, -27.44380683465356441, -8.664846435848167161 ) ) ;
#25233=CARTESIAN_POINT ( 'NONE',  ( 113.2606921295247702, 0.8980012041604618078, -13.39321520033831447 ) ) ;
#25236=CARTESIAN_POINT ( 'NONE',  ( 116.3860827545247787, -6.936859964151197211, -8.388885654883754484 ) ) ;
#25237=CARTESIAN_POINT ( 'NONE',  ( 109.2294653279517149, -0.7726726615477512716, -9.908608680919114065 ) ) ;
#25239=CARTESIAN_POINT ( 'NONE',  ( 114.5108483795247878, -0.7896495226426338832, -9.318865927141430916 ) ) ;
#25241=CARTESIAN_POINT ( 'NONE',  ( 76.69189222814998175, -45.49566950204133065, -19.39321520033831447 ) ) ;
#25242=CARTESIAN_POINT ( 'NONE',  ( 83.96621166889828203, -31.47958770101378434, -20.89321520034811641 ) ) ;
#25245=CARTESIAN_POINT ( 'NONE',  ( 109.7880358795247986, -0.7896495226426338832, -17.46756447353520159 ) ) ;
#25247=ORIENTED_EDGE ( 'NONE', *, *, #15010, .T. ) ;
#25256=CARTESIAN_POINT ( 'NONE',  ( 111.8021765045248372, -7.250697342233347165, -19.15521520033831138 ) ) ;
#25260=ORIENTED_EDGE ( 'NONE', *, *, #35036, .F. ) ;
#25264=VERTEX_POINT ( 'NONE', #9344 ) ;
#25265=DIRECTION ( 'NONE',  ( 0.9659258262890690894, 0.2588190451025180749, 0.000000000000000000 ) ) ;
#25269=CARTESIAN_POINT ( 'NONE',  ( 77.24258364551867828, -56.45027166639924587, -1.965605518563571019 ) ) ;
#25280=CARTESIAN_POINT ( 'NONE',  ( 61.69189222814998175, -69.76310523276724496, -16.89321520033831447 ) ) ;
#25282=ORIENTED_EDGE ( 'NONE', *, *, #26130, .F. ) ;
#25284=CARTESIAN_POINT ( 'NONE',  ( 113.8163171295247764, 0.1403307496149613920, -13.39321520033831447 ) ) ;
#25286=CIRCLE ( 'NONE', #11463, 5.132259260909266985 ) ;
#25291=ORIENTED_EDGE ( 'NONE', *, *, #29196, .F. ) ;
#25299=CARTESIAN_POINT ( 'NONE',  ( 106.0375671295248310, 0.1403307496149613920, -13.39321520033831447 ) ) ;
#25300=VERTEX_POINT ( 'NONE', #29413 ) ;
#25316=VERTEX_POINT ( 'NONE', #39680 ) ;
#25320=EDGE_CURVE ( 'NONE', #35019, #9951, #1809, .T. ) ;
#25322=CARTESIAN_POINT ( 'NONE',  ( 111.4549108795247747, -1.325403438956436419, -16.93181055722138595 ) ) ;
#25328=VECTOR ( 'NONE', #37501, 1000.000000000000000 ) ;
#25335=CARTESIAN_POINT ( 'NONE',  ( 116.6298240518509317, -9.627756678427191517, -15.02827327735217544 ) ) ;
#25339=ORIENTED_EDGE ( 'NONE', *, *, #10299, .T. ) ;
#25343=CARTESIAN_POINT ( 'NONE',  ( 115.5526452545247622, -9.868328341294098749, -15.46607636864997204 ) ) ;
#25344=CARTESIAN_POINT ( 'NONE',  ( 114.9970202545248412, 0.1403307496149616695, -11.32035403202665336 ) ) ;
#25352=CARTESIAN_POINT ( 'NONE',  ( 109.2294452378115039, 0.04794956319235682551, -14.87050034823130851 ) ) ;
#25356=CARTESIAN_POINT ( 'NONE',  ( 115.1359265045248605, -7.250697342233347165, -19.15521520033831138 ) ) ;
#25357=CARTESIAN_POINT ( 'NONE',  ( 113.3995983795247895, -8.402594152722688392, -16.93181055722141792 ) ) ;
#25359=CARTESIAN_POINT ( 'NONE',  ( 69.69189222814998175, -41.76310523276723785, -24.39321520033831447 ) ) ;
#25372=CARTESIAN_POINT ( 'NONE',  ( 110.6689883310706790, 0.1843591316377651834, -12.14321520033831625 ) ) ;
#25375=CARTESIAN_POINT ( 'NONE',  ( 107.9822546295247889, -4.863998795839590272, -18.39754474579285315 ) ) ;
#25378=ORIENTED_EDGE ( 'NONE', *, *, #2876, .F. ) ;
#25383=DIRECTION ( 'NONE',  ( 0.000000000000000000, 0.000000000000000000, 1.000000000000000000 ) ) ;
#25385=ORIENTED_EDGE ( 'NONE', *, *, #5771, .F. ) ;
#25386=DIRECTION ( 'NONE',  ( 0.2588190451025260685, -0.9659258262890669799, 0.000000000000000000 ) ) ;
#25388=CARTESIAN_POINT ( 'NONE',  ( 110.6214733795247867, -8.938348069036489818, -17.46756447353520159 ) ) ;
#25392=PLANE ( 'NONE',  #19649 ) ;
#25393=ORIENTED_EDGE ( 'NONE', *, *, #20393, .T. ) ;
#25397=CARTESIAN_POINT ( 'NONE',  ( 115.0664733795247798, -8.938348069036489818, -17.46756447353520159 ) ) ;
#25401=CARTESIAN_POINT ( 'NONE',  ( 62.36806374128264707, -37.05470338471879188, -5.389733333427170869 ) ) ;
#25402=CARTESIAN_POINT ( 'NONE',  ( 113.6774108795247997, -8.938348069036489818, -9.318865927141430916 ) ) ;
#25410=CARTESIAN_POINT ( 'NONE',  ( 109.2294977741537707, -10.19482194012555176, -11.51702172248756284 ) ) ;
#25413=CARTESIAN_POINT ( 'NONE',  ( 114.6497546295247929, -4.863998795839590272, -18.39754474579285315 ) ) ;
#25414=CARTESIAN_POINT ( 'NONE',  ( 113.7468640045248236, 0.1403307496149616695, -15.46607636864997204 ) ) ;
#25417=DIRECTION ( 'NONE',  ( -1.000000000000000000, 0.000000000000000000, 0.000000000000000000 ) ) ;
#25431=EDGE_CURVE ( 'NONE', #20559, #23478, #11713, .T. ) ;
#25432=CARTESIAN_POINT ( 'NONE',  ( 109.4407702545248355, -10.62599879583958717, -15.77991374673208469 ) ) ;
#25433=CARTESIAN_POINT ( 'NONE',  ( 109.2294421295247844, 7.836001204160461420, -14.64321520033831447 ) ) ;
#25434=FACE_OUTER_BOUND ( 'NONE', #24735, .T. ) ;
#25435=CARTESIAN_POINT ( 'NONE',  ( 114.7886608795247696, -1.325403438956436419, -16.93181055722141792 ) ) ;
#25443=CARTESIAN_POINT ( 'NONE',  ( 108.6073327545248048, -6.936859964151250502, -8.388885654883777576 ) ) ;
#25454=CARTESIAN_POINT ( 'NONE',  ( 113.6079577545248043, -2.791137627527939813, -18.39754474579286025 ) ) ;
#25459=CARTESIAN_POINT ( 'NONE',  ( 107.2182702545248105, -10.62599879583958717, -15.77991374673208469 ) ) ;
#25462=CARTESIAN_POINT ( 'NONE',  ( 116.1319545411901970, -0.3595008806742178709, -10.82052240173746682 ) ) ;
#25465=CARTESIAN_POINT ( 'NONE',  ( 115.4137390045248566, 0.8980012041604421569, -15.77991374673208469 ) ) ;
#25466=CARTESIAN_POINT ( 'NONE',  ( 116.8411475980424257, 1.961928045763841499, -20.95697541397089836 ) ) ;
#25467=FACE_OUTER_BOUND ( 'NONE', #781, .T. ) ;
#25470=CARTESIAN_POINT ( 'NONE',  ( 109.3713171295247832, -10.62599879583958540, -13.39321520033831447 ) ) ;
#25472=VERTEX_POINT ( 'NONE', #15962 ) ;
#25479=CARTESIAN_POINT ( 'NONE',  ( 112.5661608795247872, -8.938348069036489818, -9.318865927141430916 ) ) ;
#25480=AXIS2_PLACEMENT_3D ( 'NONE', #1131, #1354, #4323 ) ;
#25492=CARTESIAN_POINT ( 'NONE',  ( 114.9716510812576757, -0.01829820670803256055, -12.14321520033831625 ) ) ;
#25497=CYLINDRICAL_SURFACE ( 'NONE', #1074, 1.299999999999995604 ) ;
#25505=CYLINDRICAL_SURFACE ( 'NONE', #7458, 1.999999999999999112 ) ;
#25509=CARTESIAN_POINT ( 'NONE',  ( 113.1912390045248031, -9.868328341294098749, -11.32035403202665869 ) ) ;
#25510=CARTESIAN_POINT ( 'NONE',  ( 82.48419058924217495, -31.76353122097473047, -22.93120623788412615 ) ) ;
#25514=CARTESIAN_POINT ( 'NONE',  ( 115.9693640045247776, 0.1403307496149616695, -15.46607636864997204 ) ) ;
#25515=ORIENTED_EDGE ( 'NONE', *, *, #36970, .F. ) ;
#25521=CARTESIAN_POINT ( 'NONE',  ( 108.4684265045248424, -2.791137627527939813, -8.388885654883777576 ) ) ;
#25533=CARTESIAN_POINT ( 'NONE',  ( 116.5249890045247980, -9.868328341294098749, -11.32035403202665869 ) ) ;
#25546=CIRCLE ( 'NONE', #2258, 5.000000000000004441 ) ;
#25547=CARTESIAN_POINT ( 'NONE',  ( 79.79010115959992788, 5.106172230548759572, -19.89321520033831447 ) ) ;
#25559=CARTESIAN_POINT ( 'NONE',  ( 114.5108483795247878, -0.7896495226426338832, -9.318865927141430916 ) ) ;
#25560=CARTESIAN_POINT ( 'NONE',  ( 110.4131140045248287, 0.1403307496149616695, -15.46607636864997204 ) ) ;
#25561=CARTESIAN_POINT ( 'NONE',  ( 112.7745202545247878, 0.1403307496149616695, -11.32035403202665336 ) ) ;
#25562=AXIS2_PLACEMENT_3D ( 'NONE', #41062, #20525, #6840 ) ;
#25565=ORIENTED_EDGE ( 'NONE', *, *, #10543, .F. ) ;
#25567=CARTESIAN_POINT ( 'NONE',  ( 108.4684265045247997, -7.250697342233347165, -19.15521520033831138 ) ) ;
#25568=DIRECTION ( 'NONE',  ( 0.000000000000000000, 0.000000000000000000, -1.000000000000000000 ) ) ;
#25575=CARTESIAN_POINT ( 'NONE',  ( 112.0799890045248475, 0.8980012041604421569, -15.77991374673208469 ) ) ;
#25576=CARTESIAN_POINT ( 'NONE',  ( 109.9269421295247753, -9.868328341294093420, -13.39321520033831447 ) ) ;
#25594=CARTESIAN_POINT ( 'NONE',  ( 107.5655358795247736, -8.402594152722688392, -9.854619843455216355 ) ) ;
#25598=ORIENTED_EDGE ( 'NONE', *, *, #36161, .F. ) ;
#25603=ADVANCED_FACE ( 'NONE', ( #37374 ), #31089, .T. ) ;
#25605=VERTEX_POINT ( 'NONE', #11444 ) ;
#25607=CARTESIAN_POINT ( 'NONE',  ( 71.91396631829535124, -25.73035770285813939, -4.893215200338314474 ) ) ;
#25609=CARTESIAN_POINT ( 'NONE',  ( 109.5796765045248122, -7.250697342233347165, -19.15521520033831138 ) ) ;
#25615=ORIENTED_EDGE ( 'NONE', *, *, #27157, .T. ) ;
#25619=CARTESIAN_POINT ( 'NONE',  ( 116.8028015045247940, -6.936859964151250502, -18.39754474579286025 ) ) ;
#25623=ORIENTED_EDGE ( 'NONE', *, *, #35941, .T. ) ;
#25627=CARTESIAN_POINT ( 'NONE',  ( 109.3018640045248304, -10.62599879583958717, -11.00651665394454604 ) ) ;
#25629=ADVANCED_FACE ( 'NONE', ( #13851 ), #29910, .F. ) ;
#25633=CARTESIAN_POINT ( 'NONE',  ( 72.75524511225664526, -25.99489077589583630, -8.393215200338314474 ) ) ;
#25634=CARTESIAN_POINT ( 'NONE',  ( 106.3153796295248412, -4.863998795839590272, -8.388885654883775800 ) ) ;
#25635=ORIENTED_EDGE ( 'NONE', *, *, #28135, .F. ) ;
#25636=CARTESIAN_POINT ( 'NONE',  ( 109.2294321978889542, -10.20217893803289222, -14.76446976949403656 ) ) ;
#25640=CARTESIAN_POINT ( 'NONE',  ( 111.1076452545248259, -9.868328341294098749, -15.46607636864997204 ) ) ;
#25641=CARTESIAN_POINT ( 'NONE',  ( 115.6915515045247531, -6.936859964151250502, -18.39754474579286025 ) ) ;
#25655=LINE ( 'NONE', #15391, #19881 ) ;
#25658=CARTESIAN_POINT ( 'NONE',  ( 113.0523327545247838, -6.936859964151250502, -8.388885654883777576 ) ) ;
#25664=EDGE_CURVE ( 'NONE', #26785, #24453, #20483, .T. ) ;
#25666=CARTESIAN_POINT ( 'NONE',  ( 110.1353015045248469, -6.936859964151250502, -18.39754474579286025 ) ) ;
#25673=ORIENTED_EDGE ( 'NONE', *, *, #25320, .T. ) ;
#25675=CARTESIAN_POINT ( 'NONE',  ( 116.5987716749792895, -9.866677412677834269, -13.52174868289714027 ) ) ;
#25676=CARTESIAN_POINT ( 'NONE',  ( 110.0658483795247804, -8.402594152722688392, -16.93181055722141792 ) ) ;
#25681=CARTESIAN_POINT ( 'NONE',  ( 106.9404577545248145, -7.250697342233347165, -7.631215200338321125 ) ) ;
#25684=CARTESIAN_POINT ( 'NONE',  ( 78.69189222814998175, -69.76310523276724496, -16.89321520033831447 ) ) ;
#25685=PLANE ( 'NONE',  #29183 ) ;
#25687=CARTESIAN_POINT ( 'NONE',  ( 114.9275671295247889, -10.62599879583958540, -13.39321520033831447 ) ) ;
#25689=CARTESIAN_POINT ( 'NONE',  ( 82.42681365487543133, -31.76737129425208295, -22.90237778003977809 ) ) ;
#25692=CARTESIAN_POINT ( 'NONE',  ( 105.5513952545248060, 0.8980012041604421569, -11.00651665394454071 ) ) ;
#25696=VERTEX_POINT ( 'NONE', #6561 ) ;
#25704=CARTESIAN_POINT ( 'NONE',  ( 114.2330358795247776, -0.7896495226426338832, -17.46756447353520159 ) ) ;
#25715=CYLINDRICAL_SURFACE ( 'NONE', #16551, 3.000000000000002665 ) ;
#25718=CARTESIAN_POINT ( 'NONE',  ( 64.79538738837304379, -35.65327282786526553, -5.786495942213274901 ) ) ;
#25733=CARTESIAN_POINT ( 'NONE',  ( 114.0941296295247867, -4.863998795839590272, -19.15521520033831493 ) ) ;
#25734=CARTESIAN_POINT ( 'NONE',  ( 115.6220983795247861, -8.402594152722688392, -16.93181055722141792 ) ) ;
#25736=AXIS2_PLACEMENT_3D ( 'NONE', #28011, #24363, #44675 ) ;
#25741=ORIENTED_EDGE ( 'NONE', *, *, #126, .F. ) ;
#25746=CARTESIAN_POINT ( 'NONE',  ( 106.3848327545248651, -6.936859964151250502, -8.388885654883777576 ) ) ;
#25751=LINE ( 'NONE', #32575, #7367 ) ;
#25753=DIRECTION ( 'NONE',  ( -1.000000000000000000, 0.000000000000000000, 0.000000000000000000 ) ) ;
#25757=CARTESIAN_POINT ( 'NONE',  ( 114.5108483795247878, -8.402594152722688392, -16.93181055722141792 ) ) ;
#25764=CARTESIAN_POINT ( 'NONE',  ( 110.5757045411902908, -0.3595008806742185925, -10.82052240173743130 ) ) ;
#25766=AXIS2_PLACEMENT_3D ( 'NONE', #28410, #34985, #32037 ) ;
#25769=CARTESIAN_POINT ( 'NONE',  ( 69.69189222814998175, -41.76310523276723785, -20.39321520033831447 ) ) ;
#25770=CARTESIAN_POINT ( 'NONE',  ( 117.2294421295247844, 0.2335149919452661482, -4.893215200338314474 ) ) ;
#25772=CYLINDRICAL_SURFACE ( 'NONE', #13460, 5.000000000000000888 ) ;
#25782=CARTESIAN_POINT ( 'NONE',  ( 114.6515776191212836, 0.4261359969231631739, -12.14321520033831625 ) ) ;
#25784=CARTESIAN_POINT ( 'NONE',  ( 108.8851452545248151, -9.868328341294098749, -15.46607636864997204 ) ) ;
#25785=CARTESIAN_POINT ( 'NONE',  ( 108.7462390045248242, -9.868328341294098749, -11.32035403202665869 ) ) ;
#25789=CARTESIAN_POINT ( 'NONE',  ( 107.5655358795247736, -0.7896495226426338832, -17.46756447353520159 ) ) ;
#25792=FACE_OUTER_BOUND ( 'NONE', #15204, .T. ) ;
#25795=CARTESIAN_POINT ( 'NONE',  ( 111.9410827545248708, -2.477300249445798297, -19.15521520033831138 ) ) ;
#25796=CARTESIAN_POINT ( 'NONE',  ( 111.1076452545248259, -9.868328341294098749, -15.46607636864997204 ) ) ;
#25798=DIRECTION ( 'NONE',  ( -0.9970811988817437355, 0.07634843047859309062, 0.000000000000000000 ) ) ;
#25813=CARTESIAN_POINT ( 'NONE',  ( 116.4555358795247884, -0.7896495226426338832, -17.46756447353520159 ) ) ;
#25821=VERTEX_POINT ( 'NONE', #17282 ) ;
#25823=CARTESIAN_POINT ( 'NONE',  ( 71.85867159647438029, -25.32195970414818476, -4.893215200338314474 ) ) ;
#25824=CARTESIAN_POINT ( 'NONE',  ( 111.2465515045248168, -2.477300249445798297, -7.631215200338321125 ) ) ;
#25833=VECTOR ( 'NONE', #7531, 1000.000000000000000 ) ;
#25834=CARTESIAN_POINT ( 'NONE',  ( 114.9970202545248412, -10.62599879583958717, -15.77991374673208469 ) ) ;
#25835=CARTESIAN_POINT ( 'NONE',  ( 116.3166296295247832, -4.863998795839590272, -8.388885654883775800 ) ) ;
#25836=CARTESIAN_POINT ( 'NONE',  ( 113.6079577545248043, -7.250697342233347165, -7.631215200338321125 ) ) ;
#25846=CARTESIAN_POINT ( 'NONE',  ( 116.8784914538011179, -11.65352397162535603, -6.030266697614802496 ) ) ;
#25850=CARTESIAN_POINT ( 'NONE',  ( 109.2295251720720728, -9.839649396385770075, -15.65853133350598014 ) ) ;
#25852=CARTESIAN_POINT ( 'NONE',  ( 113.9552233795247815, -1.325403438956436419, -9.854619843455211026 ) ) ;
#25853=CARTESIAN_POINT ( 'NONE',  ( 105.6903015045248253, -2.477300249445798297, -7.631215200338321125 ) ) ;
#25856=CARTESIAN_POINT ( 'NONE',  ( 69.81876103444739101, -25.95566152907768753, -5.787138065658625763 ) ) ;
#25857=EDGE_CURVE ( 'NONE', #35384, #17767, #24820, .T. ) ;
#25861=EDGE_CURVE ( 'NONE', #30491, #23154, #15354, .T. ) ;
#25879=CARTESIAN_POINT ( 'NONE',  ( 114.8581140045248361, 0.1403307496149616695, -15.46607636864997204 ) ) ;
#25886=CARTESIAN_POINT ( 'NONE',  ( 110.6909265045248247, -2.791137627527939813, -8.388885654883777576 ) ) ;
#25894=ORIENTED_EDGE ( 'NONE', *, *, #30301, .F. ) ;
#25897=CARTESIAN_POINT ( 'NONE',  ( 110.4131140045248287, 0.1403307496149616695, -15.46607636864997204 ) ) ;
#25903=CARTESIAN_POINT ( 'NONE',  ( 108.8156921295247912, 0.8980012041604618078, -13.39321520033831447 ) ) ;
#25909=CARTESIAN_POINT ( 'NONE',  ( 114.7886608795247696, -8.938348069036489818, -9.318865927141430916 ) ) ;
#25911=CARTESIAN_POINT ( 'NONE',  ( 84.02342478082003652, -31.32369313687246049, -21.95975535756046071 ) ) ;
#25914=CARTESIAN_POINT ( 'NONE',  ( 108.8156921295247912, 0.8980012041604618078, -13.39321520033831447 ) ) ;
#25920=EDGE_CURVE ( 'NONE', #15215, #21469, #12231, .T. ) ;
#25926=CARTESIAN_POINT ( 'NONE',  ( 109.2324108795247923, -8.938348069036489818, -9.318865927141430916 ) ) ;
#25928=CARTESIAN_POINT ( 'NONE',  ( 116.7565503026016813, -4.863998795840742240, -18.55532337341522364 ) ) ;
#25941=CARTESIAN_POINT ( 'NONE',  ( 65.06330879403716949, -35.71473443186641816, -5.721420406450495655 ) ) ;
#25952=CARTESIAN_POINT ( 'NONE',  ( 114.4413952545248350, -9.868328341294098749, -15.46607636864997204 ) ) ;
#25954=ORIENTED_EDGE ( 'NONE', *, *, #29962, .F. ) ;
#25956=CARTESIAN_POINT ( 'NONE',  ( 113.8857702545248003, -10.62599879583958717, -15.77991374673208469 ) ) ;
#25957=CARTESIAN_POINT ( 'NONE',  ( 108.8156921295247912, -9.868328341294093420, -13.39321520033831447 ) ) ;
#25960=CARTESIAN_POINT ( 'NONE',  ( 84.39081516114408998, -30.32262605124144272, -9.757176231017245627 ) ) ;
#25962=CARTESIAN_POINT ( 'NONE',  ( 116.7333483795247844, -8.402594152722688392, -16.93181055722141792 ) ) ;
#25969=CARTESIAN_POINT ( 'NONE',  ( 105.9681140045248355, 0.1403307496149616695, -15.46607636864997204 ) ) ;
#25972=CARTESIAN_POINT ( 'NONE',  ( 116.2659068881580708, -12.01880880694303855, -20.89321520033831447 ) ) ;
#25978=CARTESIAN_POINT ( 'NONE',  ( 71.67504600870660170, -26.72445618319088823, -4.893215200338314474 ) ) ;
#25980=EDGE_CURVE ( 'NONE', #27061, #13571, #5376, .T. ) ;
#25982=CARTESIAN_POINT ( 'NONE',  ( 116.8028015045247940, -6.936859964151250502, -18.39754474579286025 ) ) ;
#25994=CARTESIAN_POINT ( 'NONE',  ( 64.69189222814998175, -41.76310523276723785, -23.89321520033831803 ) ) ;
#25995=CARTESIAN_POINT ( 'NONE',  ( 79.79010115959992788, 5.106172230548759572, -12.14321520033831625 ) ) ;
#26004=CARTESIAN_POINT ( 'NONE',  ( 116.6639544560221253, -8.875725282760177137, -16.49651588959498127 ) ) ;
#26011=CARTESIAN_POINT ( 'NONE',  ( 114.0246765045248196, -7.250697342233347165, -19.15521520033831138 ) ) ;
#26012=CARTESIAN_POINT ( 'NONE',  ( 111.6632702545248605, 0.1403307496149616695, -11.32035403202665336 ) ) ;
#26013=CARTESIAN_POINT ( 'NONE',  ( 108.8156921295247912, -9.868328341294093420, -13.39321520033831447 ) ) ;
#26016=VERTEX_POINT ( 'NONE', #33392 ) ;
#26017=CARTESIAN_POINT ( 'NONE',  ( 105.8986608795248401, -8.938348069036489818, -9.318865927141430916 ) ) ;
#26022=CARTESIAN_POINT ( 'NONE',  ( 111.1076452545248259, 0.8980012041604421569, -11.00651665394454071 ) ) ;
#26025=CARTESIAN_POINT ( 'NONE',  ( 110.4384831777918805, -0.01829820670803256055, -14.64321520033831447 ) ) ;
#26041=CARTESIAN_POINT ( 'NONE',  ( 107.4266296295248821, -4.863998795839590272, -8.388885654883775800 ) ) ;
#26046=ADVANCED_FACE ( 'NONE', ( #36600 ), #32074, .T. ) ;
#26051=CARTESIAN_POINT ( 'NONE',  ( 62.16333102610810357, -65.29371840568624918, -44.88093227629854454 ) ) ;
#26052=CARTESIAN_POINT ( 'NONE',  ( 106.8015515045248378, -2.477300249445798297, -7.631215200338321125 ) ) ;
#26059=EDGE_LOOP ( 'NONE', ( #20722, #7797 ) ) ;
#26062=CARTESIAN_POINT ( 'NONE',  ( 110.8992858795247827, -0.7896495226426338832, -17.46756447353520159 ) ) ;
#26064=CARTESIAN_POINT ( 'NONE',  ( 112.8439733795247832, -8.938348069036489818, -17.46756447353520159 ) ) ;
#26069=CARTESIAN_POINT ( 'NONE',  ( 107.4960827545248350, -2.477300249445798297, -19.15521520033831138 ) ) ;
#26073=CARTESIAN_POINT ( 'NONE',  ( 117.1996198715402215, -11.04292984039206793, -5.371871346472351760 ) ) ;
#26074=ORIENTED_EDGE ( 'NONE', *, *, #1650, .F. ) ;
#26076=CARTESIAN_POINT ( 'NONE',  ( 109.2295177676240456, -10.22869049659968610, -11.63402529915072492 ) ) ;
#26078=CARTESIAN_POINT ( 'NONE',  ( 111.5243640045248412, 0.1403307496149616695, -15.46607636864997204 ) ) ;
#26079=CARTESIAN_POINT ( 'NONE',  ( 106.2459265045248173, -7.250697342233347165, -19.15521520033831138 ) ) ;
#26082=CARTESIAN_POINT ( 'NONE',  ( 69.74921804855158314, -26.23096954073753651, -5.785566283887345840 ) ) ;
#26091=ORIENTED_EDGE ( 'NONE', *, *, #31166, .T. ) ;
#26096=CARTESIAN_POINT ( 'NONE',  ( 109.0240515045248202, -2.477300249445798297, -7.631215200338321125 ) ) ;
#26098=CARTESIAN_POINT ( 'NONE',  ( 117.2294421295247844, 1.035107641088057973, -4.893215200338314474 ) ) ;
#26099=CARTESIAN_POINT ( 'NONE',  ( 110.2047546295247855, -4.863998795839590272, -18.39754474579285315 ) ) ;
#26107=CARTESIAN_POINT ( 'NONE',  ( 109.3713171295247832, 0.1403307496149613920, -13.39321520033831447 ) ) ;
#26113=CARTESIAN_POINT ( 'NONE',  ( 71.48339778575683567, -26.67534733500407640, -5.037593897558821254 ) ) ;
#26115=VECTOR ( 'NONE', #2462, 1000.000000000000000 ) ;
#26117=EDGE_LOOP ( 'NONE', ( #15308, #25741 ) ) ;
#26119=DIRECTION ( 'NONE',  ( 1.000000000000000000, 0.000000000000000000, 0.000000000000000000 ) ) ;
#26120=CARTESIAN_POINT ( 'NONE',  ( 110.7603796295247918, -4.863998795839590272, -8.388885654883775800 ) ) ;
#26125=CARTESIAN_POINT ( 'NONE',  ( 106.6626452545248611, 0.8980012041604421569, -11.00651665394454071 ) ) ;
#26129=CARTESIAN_POINT ( 'NONE',  ( 108.6767858795247861, -0.7896495226426338832, -17.46756447353520159 ) ) ;
#26130=EDGE_CURVE ( 'NONE', #3693, #408, #1948, .T. ) ;
#26132=CARTESIAN_POINT ( 'NONE',  ( 84.10271796608054728, -31.10763468207608895, -20.89321520033831447 ) ) ;
#26135=CARTESIAN_POINT ( 'NONE',  ( 106.2459265045248173, -7.250697342233347165, -19.15521520033831138 ) ) ;
#26140=ORIENTED_EDGE ( 'NONE', *, *, #9691, .T. ) ;
#26141=CARTESIAN_POINT ( 'NONE',  ( 112.1114130180079798, 0.7607806665037644134, -14.64321520033833046 ) ) ;
#26148=CARTESIAN_POINT ( 'NONE',  ( 109.7880358795247986, -0.7896495226426338832, -17.46756447353520159 ) ) ;
#26150=CARTESIAN_POINT ( 'NONE',  ( 110.8298327545248299, -2.477300249445798297, -19.15521520033832203 ) ) ;
#26155=ADVANCED_FACE ( 'NONE', ( #29771 ), #25685, .F. ) ;
#26156=LINE ( 'NONE', #42593, #34922 ) ;
#26165=CARTESIAN_POINT ( 'NONE',  ( 109.8889130180080826, 0.7607806665037644134, -14.64321520033833579 ) ) ;
#26175=CARTESIAN_POINT ( 'NONE',  ( 114.6497546295247929, -4.863998795839590272, -18.39754474579285315 ) ) ;
#26179=CARTESIAN_POINT ( 'NONE',  ( 115.6915515045247531, -2.477300249445798297, -7.631215200338321125 ) ) ;
#26180=CARTESIAN_POINT ( 'NONE',  ( 107.8433483795247838, -8.402594152722688392, -16.93181055722141792 ) ) ;
#26185=CARTESIAN_POINT ( 'NONE',  ( 114.9970202545248412, 0.1403307496149616695, -11.32035403202665336 ) ) ;
#26186=ORIENTED_EDGE ( 'NONE', *, *, #29029, .F. ) ;
#26192=LINE ( 'NONE', #32569, #34089 ) ;
#26193=CARTESIAN_POINT ( 'NONE',  ( 107.7738952545248310, -9.868328341294098749, -15.46607636864997204 ) ) ;
#26201=CARTESIAN_POINT ( 'NONE',  ( 85.75809888461174069, -18.45227461768569199, -4.893215200338314474 ) ) ;
#26203=CARTESIAN_POINT ( 'NONE',  ( 112.2188952545247531, -9.868328341294098749, -15.46607636864997204 ) ) ;
#26205=CARTESIAN_POINT ( 'NONE',  ( 78.69189222814998175, -59.27884951796255564, -42.87418841894956500 ) ) ;
#26209=FACE_OUTER_BOUND ( 'NONE', #36303, .T. ) ;
#26232=CARTESIAN_POINT ( 'NONE',  ( 109.8574890045247940, 0.8980012041604421569, -15.77991374673208469 ) ) ;
#26233=CARTESIAN_POINT ( 'NONE',  ( 111.7327233795247849, -1.325403438956436419, -9.854619843455211026 ) ) ;
#26234=CARTESIAN_POINT ( 'NONE',  ( 107.2877233795247776, -1.325403438956436419, -9.854619843455211026 ) ) ;
#26243=CARTESIAN_POINT ( 'NONE',  ( 108.8851452545248151, 0.8980012041604421569, -11.00651665394454071 ) ) ;
#26253=EDGE_CURVE ( 'NONE', #31317, #15833, #33525, .T. ) ;
#26266=CARTESIAN_POINT ( 'NONE',  ( 113.9552233795247815, -8.938348069036489818, -17.46756447353520159 ) ) ;
#26277=CARTESIAN_POINT ( 'NONE',  ( 105.8986608795248401, -8.938348069036489818, -9.318865927141430916 ) ) ;
#26287=CARTESIAN_POINT ( 'NONE',  ( 112.4967077545247633, -7.250697342233347165, -7.631215200338321125 ) ) ;
#26290=CARTESIAN_POINT ( 'NONE',  ( 113.8857702545248003, -10.62599879583958717, -15.77991374673208469 ) ) ;
#26293=AXIS2_PLACEMENT_3D ( 'NONE', #15735, #22566, #44010 ) ;
#26295=CARTESIAN_POINT ( 'NONE',  ( 63.10563328194941590, -37.74164650239046637, -4.980946376743919046 ) ) ;
#26296=CARTESIAN_POINT ( 'NONE',  ( 107.7044421295247929, 0.8980012041604618078, -13.39321520033831447 ) ) ;
#26299=DIRECTION ( 'NONE',  ( 0.000000000000000000, 1.000000000000000000, 0.000000000000000000 ) ) ;
#26300=CARTESIAN_POINT ( 'NONE',  ( 116.9233217481409355, -11.60109430213782744, -5.955714001824102155 ) ) ;
#26303=CARTESIAN_POINT ( 'NONE',  ( 109.2294327885794161, -10.27098468477303150, -14.50962478522546739 ) ) ;
#26305=EDGE_CURVE ( 'NONE', #34946, #17270, #25546, .T. ) ;
#26306=CARTESIAN_POINT ( 'NONE',  ( 112.2883483795247770, -8.402594152722688392, -16.93181055722141792 ) ) ;
#26307=CARTESIAN_POINT ( 'NONE',  ( 109.3713171295247832, 0.1403307496149613920, -13.39321520033831447 ) ) ;
#26310=CARTESIAN_POINT ( 'NONE',  ( 71.33058836615619214, -26.45114454543378812, -5.217245182119505387 ) ) ;
#26323=EDGE_CURVE ( 'NONE', #37706, #42269, #22101, .T. ) ;
#26326=CARTESIAN_POINT ( 'NONE',  ( 105.8292077545248446, -7.250697342233347165, -7.631215200338321125 ) ) ;
#26328=CARTESIAN_POINT ( 'NONE',  ( 69.69189222814998175, -41.76310523276723785, -47.71602681600972318 ) ) ;
#26329=CARTESIAN_POINT ( 'NONE',  ( 111.3854577545248645, -2.791137627527939813, -18.39754474579286025 ) ) ;
#26336=CARTESIAN_POINT ( 'NONE',  ( 116.5249890045247980, -9.868328341294098749, -11.32035403202665869 ) ) ;
#26337=CARTESIAN_POINT ( 'NONE',  ( 107.7738952545248310, -9.868328341294098749, -15.46607636864997204 ) ) ;
#26350=CARTESIAN_POINT ( 'NONE',  ( 109.3018640045248304, 0.1403307496149616695, -15.46607636864997204 ) ) ;
#26354=CARTESIAN_POINT ( 'NONE',  ( 105.9681140045248355, -10.62599879583958717, -11.00651665394454604 ) ) ;
#26355=CONICAL_SURFACE ( 'NONE', #14705, 5.000000000000000888, 0.7853981633974419507 ) ;
#26358=DIRECTION ( 'NONE',  ( 4.295035233247849253E-16, 0.3713878862591650232, -0.9284778069183718952 ) ) ;
#26359=CARTESIAN_POINT ( 'NONE',  ( 113.0523327545247838, -2.477300249445798297, -19.15521520033831138 ) ) ;
#26361=CARTESIAN_POINT ( 'NONE',  ( 115.7610046295247912, -4.863998795839590272, -7.631215200338315796 ) ) ;
#26366=CYLINDRICAL_SURFACE ( 'NONE', #29396, 5.000000000000004441 ) ;
#26375=CARTESIAN_POINT ( 'NONE',  ( 108.5378796295247810, -4.863998795839590272, -19.15521520033831493 ) ) ;
#26376=AXIS2_PLACEMENT_3D ( 'NONE', #28087, #3462, #261 ) ;
#26378=CARTESIAN_POINT ( 'NONE',  ( 109.9649712410415816, 0.7607806665038616689, -12.14321520033831625 ) ) ;
#26383=CARTESIAN_POINT ( 'NONE',  ( 69.01908044833263034, -25.32952000468398879, -5.893215200338315363 ) ) ;
#26386=DIRECTION ( 'NONE',  ( 0.000000000000000000, 0.000000000000000000, 1.000000000000000000 ) ) ;
#26400=CARTESIAN_POINT ( 'NONE',  ( 115.9693640045247776, 0.1403307496149616695, -15.46607636864997204 ) ) ;
#26404=CARTESIAN_POINT ( 'NONE',  ( 106.5237390045248418, -9.868328341294098749, -11.32035403202665869 ) ) ;
#26405=CARTESIAN_POINT ( 'NONE',  ( 110.6909265045248247, -2.791137627527939813, -8.388885654883777576 ) ) ;
#26411=CARTESIAN_POINT ( 'NONE',  ( 111.6632702545248605, 0.1403307496149616695, -11.32035403202665336 ) ) ;
#26419=CARTESIAN_POINT ( 'NONE',  ( 105.2735827545248810, -6.936859964151250502, -8.388885654883777576 ) ) ;
#26421=VERTEX_POINT ( 'NONE', #11394 ) ;
#26422=AXIS2_PLACEMENT_3D ( 'NONE', #17688, #11748, #15162 ) ;
#26427=CARTESIAN_POINT ( 'NONE',  ( 72.75524511225664526, -25.99489077589588604, -12.39321520033831447 ) ) ;
#26431=CARTESIAN_POINT ( 'NONE',  ( 112.9134265045247645, -2.791137627527939813, -8.388885654883777576 ) ) ;
#26441=ORIENTED_EDGE ( 'NONE', *, *, #29340, .F. ) ;
#26462=VERTEX_POINT ( 'NONE', #26627 ) ;
#26464=CARTESIAN_POINT ( 'NONE',  ( 110.9687390045248350, 0.8980012041604421569, -15.77991374673208469 ) ) ;
#26465=CARTESIAN_POINT ( 'NONE',  ( 108.1211608795247798, -1.325403438956436419, -16.93181055722141792 ) ) ;
#26466=CARTESIAN_POINT ( 'NONE',  ( 107.5655358795247736, -8.402594152722688392, -9.854619843455216355 ) ) ;
#26471=CARTESIAN_POINT ( 'NONE',  ( 66.82415148905926117, -40.21211973637273474, -23.89321520033831803 ) ) ;
#26472=CARTESIAN_POINT ( 'NONE',  ( 117.2294421295247844, -10.76310523276723785, -21.89255013987451548 ) ) ;
#26475=CARTESIAN_POINT ( 'NONE',  ( 106.0375671295248310, 0.1403307496149613920, -13.39321520033831447 ) ) ;
#26477=CARTESIAN_POINT ( 'NONE',  ( 108.5378796295247810, -4.863998795839590272, -19.15521520033831493 ) ) ;
#26486=DIRECTION ( 'NONE',  ( 0.000000000000000000, 0.000000000000000000, -1.000000000000000000 ) ) ;
#26497=CARTESIAN_POINT ( 'NONE',  ( 114.5803015045248117, -2.477300249445798297, -7.631215200338321125 ) ) ;
#26506=LINE ( 'NONE', #40185, #34947 ) ;
#26518=CARTESIAN_POINT ( 'NONE',  ( 114.7192077545248594, -7.250697342233347165, -7.631215200338321125 ) ) ;
#26519=CARTESIAN_POINT ( 'NONE',  ( 112.3578015045248861, -6.936859964151250502, -18.39754474579286025 ) ) ;
#26520=CARTESIAN_POINT ( 'NONE',  ( 110.5520202545248054, -10.62599879583958717, -15.77991374673208469 ) ) ;
#26524=CARTESIAN_POINT ( 'NONE',  ( 61.76986277844709861, -39.32091226840162079, -7.393215200338315363 ) ) ;
#26525=CARTESIAN_POINT ( 'NONE',  ( 106.6626452545248611, 0.8980012041604421569, -11.00651665394454071 ) ) ;
#26529=FACE_OUTER_BOUND ( 'NONE', #3065, .T. ) ;
#26534=CARTESIAN_POINT ( 'NONE',  ( 111.8716296295247901, -4.863998795839590272, -8.388885654883775800 ) ) ;
#26535=CARTESIAN_POINT ( 'NONE',  ( 109.0935046295247872, -4.863998795839590272, -18.39754474579285315 ) ) ;
#26537=CARTESIAN_POINT ( 'NONE',  ( 67.69189222814998175, -55.76310523276723785, -40.89321520033831092 ) ) ;
#26538=CARTESIAN_POINT ( 'NONE',  ( 68.93854012757255134, -25.83497651491618896, -5.893215200338315363 ) ) ;
#26548=ADVANCED_FACE ( 'NONE', ( #32778 ), #37194, .T. ) ;
#26552=CARTESIAN_POINT ( 'NONE',  ( 106.3153796295248412, -4.863998795839590272, -19.15521520033831493 ) ) ;
#26556=CARTESIAN_POINT ( 'NONE',  ( 110.4825671295247815, 0.1403307496149613920, -13.39321520033831447 ) ) ;
#26557=EDGE_CURVE ( 'NONE', #8479, #20261, #1539, .T. ) ;
#26558=LINE ( 'NONE', #43438, #7390 ) ;
#26562=ORIENTED_EDGE ( 'NONE', *, *, #43752, .F. ) ;
#26563=CARTESIAN_POINT ( 'NONE',  ( 109.2294421295247844, -11.83367149576868727, -19.39321520033831447 ) ) ;
#26568=DIRECTION ( 'NONE',  ( 0.7071067811865520136, 8.659560562354881089E-17, 0.7071067811865431318 ) ) ;
#26569=CARTESIAN_POINT ( 'NONE',  ( 113.9077908578216807, 0.04929351793716424401, -12.14321520033834467 ) ) ;
#26575=CARTESIAN_POINT ( 'NONE',  ( 111.1770983795247787, -8.402594152722688392, -16.93181055722141792 ) ) ;
#26579=CARTESIAN_POINT ( 'NONE',  ( 113.3301452545248083, -9.868328341294098749, -15.46607636864997204 ) ) ;
#26584=CARTESIAN_POINT ( 'NONE',  ( 112.2883483795247770, -0.7896495226426338832, -9.318865927141430916 ) ) ;
#26586=CARTESIAN_POINT ( 'NONE',  ( 113.3995983795247895, -0.7896495226426338832, -9.318865927141430916 ) ) ;
#26594=AXIS2_PLACEMENT_3D ( 'NONE', #39900, #4784, #18704 ) ;
#26602=CARTESIAN_POINT ( 'NONE',  ( 108.1211608795247798, -8.938348069036489818, -9.318865927141430916 ) ) ;
#26609=CARTESIAN_POINT ( 'NONE',  ( 112.9828796295247884, -4.863998795839638234, -8.388885654883775800 ) ) ;
#26612=CARTESIAN_POINT ( 'NONE',  ( 116.9333032873346383, 1.865211299501440712, -5.695039816857145887 ) ) ;
#26614=CARTESIAN_POINT ( 'NONE',  ( 106.8015515045248378, -6.936859964151250502, -18.39754474579286025 ) ) ;
#26626=CARTESIAN_POINT ( 'NONE',  ( 116.6638952545248031, -9.868328341294098749, -15.46607636864997204 ) ) ;
#26627=CARTESIAN_POINT ( 'NONE',  ( 65.19189222814998175, -41.76310523276723785, -6.393215200338315363 ) ) ;
#26631=CARTESIAN_POINT ( 'NONE',  ( 106.3848327545248651, -6.936859964151250502, -8.388885654883777576 ) ) ;
#26632=CARTESIAN_POINT ( 'NONE',  ( 109.7880358795247986, -8.402594152722688392, -9.854619843455216355 ) ) ;
#26633=CARTESIAN_POINT ( 'NONE',  ( 82.80200173989635459, -31.79535628182557971, -23.14532950183733462 ) ) ;
#26636=LINE ( 'NONE', #40549, #21164 ) ;
#26637=CARTESIAN_POINT ( 'NONE',  ( 114.3719421295247827, -9.868328341294093420, -13.39321520033831447 ) ) ;
#26638=ORIENTED_EDGE ( 'NONE', *, *, #42590, .T. ) ;
#26639=CARTESIAN_POINT ( 'NONE',  ( 109.2296068920433783, -0.1296147630240877813, -15.30322596940846758 ) ) ;
#26645=CARTESIAN_POINT ( 'NONE',  ( 117.0091510799717014, -11.49078741053932085, -21.62708738602523084 ) ) ;
#26653=AXIS2_PLACEMENT_3D ( 'NONE', #3889, #24650, #25103 ) ;
#26654=CARTESIAN_POINT ( 'NONE',  ( 110.7603796295247918, -4.863998795839590272, -8.388885654883775800 ) ) ;
#26657=ORIENTED_EDGE ( 'NONE', *, *, #17831, .F. ) ;
#26663=EDGE_LOOP ( 'NONE', ( #9612, #15578, #33909, #37534, #6421, #43086, #28033, #13646, #37100, #41153, #7590, #43065, #14601, #10107, #9011, #4139, #18744, #36831, #36642, #38439, #28892, #12436, #17983 ) ) ;
#26667=CARTESIAN_POINT ( 'NONE',  ( 110.2742077545248236, -2.791137627527887410, -18.39754474579284249 ) ) ;
#26668=CARTESIAN_POINT ( 'NONE',  ( 79.05243529145373316, 4.793396140045460108, -14.64321520033831447 ) ) ;
#26672=EDGE_CURVE ( 'NONE', #27457, #12848, #38184, .T. ) ;
#26686=CARTESIAN_POINT ( 'NONE',  ( 110.2742077545248094, -7.250697342233347165, -7.631215200338321125 ) ) ;
#26688=CARTESIAN_POINT ( 'NONE',  ( 105.4124890045248293, -9.868328341294098749, -11.32035403202665869 ) ) ;
#26689=CARTESIAN_POINT ( 'NONE',  ( 107.0793640045248196, 0.1403307496149616695, -15.46607636864997204 ) ) ;
#26695=CARTESIAN_POINT ( 'NONE',  ( 105.1346765045248475, -2.791137627527939813, -8.388885654883777576 ) ) ;
#26698=CARTESIAN_POINT ( 'NONE',  ( 114.9970202545248412, 0.1403307496149616695, -11.32035403202665336 ) ) ;
#26700=ORIENTED_EDGE ( 'NONE', *, *, #11402, .F. ) ;
#26701=CARTESIAN_POINT ( 'NONE',  ( 110.7102801496069873, 0.3591747506842615789, -14.64321520033831447 ) ) ;
#26719=CARTESIAN_POINT ( 'NONE',  ( 112.7050671295247923, -10.62599879583958540, -13.39321520033831447 ) ) ;
#26723=ORIENTED_EDGE ( 'NONE', *, *, #26557, .F. ) ;
#26728=CARTESIAN_POINT ( 'NONE',  ( 143.3676850761856940, -49.76310523276723785, -13.39321520033831447 ) ) ;
#26731=CARTESIAN_POINT ( 'NONE',  ( 108.2600671295247992, -10.62599879583958540, -13.39321520033831447 ) ) ;
#26744=CARTESIAN_POINT ( 'NONE',  ( 111.8021765045248372, -7.250697342233347165, -19.15521520033831138 ) ) ;
#26745=CARTESIAN_POINT ( 'NONE',  ( 111.6632702545248605, 0.1403307496149616695, -11.32035403202665336 ) ) ;
#26746=CARTESIAN_POINT ( 'NONE',  ( 111.1770983795247787, -0.7896495226426338832, -9.318865927141430916 ) ) ;
#26763=CARTESIAN_POINT ( 'NONE',  ( 107.9822546295247889, -4.863998795839590272, -18.39754474579285315 ) ) ;
#26764=CARTESIAN_POINT ( 'NONE',  ( 112.9134265045247645, -2.791137627527939813, -8.388885654883777576 ) ) ;
#26767=CARTESIAN_POINT ( 'NONE',  ( 71.45370786120086848, -25.93374482621613808, -5.221195830126694304 ) ) ;
#26770=ORIENTED_EDGE ( 'NONE', *, *, #27842, .F. ) ;
#26776=ORIENTED_EDGE ( 'NONE', *, *, #27007, .F. ) ;
#26783=CARTESIAN_POINT ( 'NONE',  ( 108.8851452545248151, 0.8980012041604421569, -11.00651665394454071 ) ) ;
#26785=VERTEX_POINT ( 'NONE', #24200 ) ;
#26786=CARTESIAN_POINT ( 'NONE',  ( 110.2742077545248094, -2.791137627527939813, -18.39754474579286025 ) ) ;
#26799=EDGE_LOOP ( 'NONE', ( #37306, #5841, #26638, #8211 ) ) ;
#26802=CARTESIAN_POINT ( 'NONE',  ( 107.1488171295247867, 0.1403307496149613920, -13.39321520033831447 ) ) ;
#26807=CARTESIAN_POINT ( 'NONE',  ( 112.4967077545247633, -2.791137627527939813, -18.39754474579286025 ) ) ;
#26811=CARTESIAN_POINT ( 'NONE',  ( 111.3854577545248645, -7.250697342233347165, -7.631215200338321125 ) ) ;
#26813=CARTESIAN_POINT ( 'NONE',  ( 112.0799890045248475, 0.8980012041604421569, -15.77991374673208469 ) ) ;
#26816=DIRECTION ( 'NONE',  ( 0.000000000000000000, 0.000000000000000000, -1.000000000000000000 ) ) ;
#26830=CARTESIAN_POINT ( 'NONE',  ( 107.4266296295248821, -4.863998795839590272, -19.15521520033831493 ) ) ;
#26840=CARTESIAN_POINT ( 'NONE',  ( 116.4318426488974580, 2.234111456617531744, -6.383118217132903283 ) ) ;
#26842=CARTESIAN_POINT ( 'NONE',  ( 106.7320983795247855, -8.402594152722688392, -16.93181055722141792 ) ) ;
#26852=CARTESIAN_POINT ( 'NONE',  ( 114.1635827545248389, -6.936859964151250502, -8.388885654883777576 ) ) ;
#26856=CARTESIAN_POINT ( 'NONE',  ( 111.9410827545248708, -2.477300249445798297, -19.15521520033831138 ) ) ;
#26857=CARTESIAN_POINT ( 'NONE',  ( 107.5655358795247736, -8.402594152722688392, -9.854619843455216355 ) ) ;
#26858=CARTESIAN_POINT ( 'NONE',  ( 82.85202896377741411, -31.80474036673594540, -23.17876345974346819 ) ) ;
#26862=CARTESIAN_POINT ( 'NONE',  ( 112.3578015045248861, -6.936859964151250502, -18.39754474579286025 ) ) ;
#26863=EDGE_LOOP ( 'NONE', ( #25056, #3371, #25954, #45064 ) ) ;
#26870=CARTESIAN_POINT ( 'NONE',  ( 105.1346765045248475, -2.791137627527939813, -8.388885654883777576 ) ) ;
#26874=ADVANCED_FACE ( 'NONE', ( #24862 ), #4549, .F. ) ;
#26879=CARTESIAN_POINT ( 'NONE',  ( 111.0381921295247878, -9.868328341294093420, -13.39321520033831447 ) ) ;
#26881=CARTESIAN_POINT ( 'NONE',  ( 83.82415148905927538, -46.76310523276723785, -4.893215200338314474 ) ) ;
#26882=ORIENTED_EDGE ( 'NONE', *, *, #11970, .T. ) ;
#26896=CARTESIAN_POINT ( 'NONE',  ( 114.5108483795247878, -8.402594152722688392, -16.93181055722141792 ) ) ;
#26909=CARTESIAN_POINT ( 'NONE',  ( 111.6632702545248605, -10.62599879583958717, -15.77991374673208469 ) ) ;
#26914=ORIENTED_EDGE ( 'NONE', *, *, #24189, .T. ) ;
#26920=CARTESIAN_POINT ( 'NONE',  ( 106.1764733795248219, -8.938348069036489818, -17.46756447353520159 ) ) ;
#26939=CARTESIAN_POINT ( 'NONE',  ( 111.5938171295247940, -10.62599879583958540, -13.39321520033831447 ) ) ;
#26951=CARTESIAN_POINT ( 'NONE',  ( 107.0099108795247815, -8.938348069036489818, -9.318865927141430916 ) ) ;
#26960=DIRECTION ( 'NONE',  ( -1.237391069487127839E-47, -1.069961080215129965E-32, 1.000000000000000000 ) ) ;
#26962=CARTESIAN_POINT ( 'NONE',  ( 107.2877233795247776, -8.938348069036489818, -17.46756447353520159 ) ) ;
#26963=CARTESIAN_POINT ( 'NONE',  ( 113.5385046295247804, -4.863998795839590272, -18.39754474579285315 ) ) ;
#26964=CARTESIAN_POINT ( 'NONE',  ( 107.0793640045248196, -10.62599879583958717, -11.00651665394454604 ) ) ;
#26973=( BOUNDED_CURVE ( )  B_SPLINE_CURVE ( 3, ( #27141, #20747, #37149, #10051 ),
 .UNSPECIFIED., .F., .F. ) 
 B_SPLINE_CURVE_WITH_KNOTS ( ( 4, 4 ),
 ( 3.141592653589795336, 4.712388980384689674 ),
 .UNSPECIFIED. ) 
 CURVE ( )  GEOMETRIC_REPRESENTATION_ITEM ( )  RATIONAL_B_SPLINE_CURVE ( ( 1.000000000000000000, 0.8047378541243659367, 0.8047378541243659367, 1.000000000000000000 ) ) 
 REPRESENTATION_ITEM ( '' )  );
#26979=ORIENTED_EDGE ( 'NONE', *, *, #43722, .F. ) ;
#26984=CARTESIAN_POINT ( 'NONE',  ( 106.4542858795248179, -8.402594152722688392, -9.854619843455216355 ) ) ;
#26985=CARTESIAN_POINT ( 'NONE',  ( 113.1912390045248031, -9.868328341294098749, -11.32035403202665869 ) ) ;
#26996=ORIENTED_EDGE ( 'NONE', *, *, #25431, .T. ) ;
#27006=VERTEX_POINT ( 'NONE', #4775 ) ;
#27007=EDGE_CURVE ( 'NONE', #30187, #22775, #23299, .T. ) ;
#27009=CARTESIAN_POINT ( 'NONE',  ( 111.1076452545248259, -9.868328341294098749, -15.46607636864997204 ) ) ;
#27025=CARTESIAN_POINT ( 'NONE',  ( 70.91713523389951490, -26.53035501928088635, -5.366017652747787636 ) ) ;
#27031=CARTESIAN_POINT ( 'NONE',  ( 114.3024890045248156, 0.8980012041604421569, -15.77991374673208469 ) ) ;
#27035=CARTESIAN_POINT ( 'NONE',  ( 113.0523327545247838, -6.936859964151250502, -8.388885654883777576 ) ) ;
#27037=CARTESIAN_POINT ( 'NONE',  ( 115.9947331777918862, -0.01829820670803256055, -14.64321520033831447 ) ) ;
#27039=CARTESIAN_POINT ( 'NONE',  ( 112.8439733795247832, -8.938348069036489818, -17.46756447353520159 ) ) ;
#27041=CARTESIAN_POINT ( 'NONE',  ( 115.0664733795247798, -8.938348069036489818, -17.46756447353520159 ) ) ;
#27044=CARTESIAN_POINT ( 'NONE',  ( 114.9970202545248554, -10.62599879583958540, -15.77991374673209179 ) ) ;
#27057=CARTESIAN_POINT ( 'NONE',  ( 110.8992858795247827, -8.402594152722688392, -9.854619843455216355 ) ) ;
#27060=CARTESIAN_POINT ( 'NONE',  ( 112.0105358795247810, -0.7896495226426338832, -17.46756447353520159 ) ) ;
#27061=VERTEX_POINT ( 'NONE', #41100 ) ;
#27063=CARTESIAN_POINT ( 'NONE',  ( 113.1259820646196914, 0.6269505268395592079, -14.64321520033833579 ) ) ;
#27065=CARTESIAN_POINT ( 'NONE',  ( 113.3301452545248083, -9.868328341294102302, -15.46607636865002355 ) ) ;
#27066=CIRCLE ( 'NONE', #35767, 5.999999999999998224 ) ;
#27068=CARTESIAN_POINT ( 'NONE',  ( 116.3808264296373807, 2.254317590850374309, -6.449063452130288532 ) ) ;
#27070=CARTESIAN_POINT ( 'NONE',  ( 108.7462390045248242, -9.868328341294098749, -11.32035403202665869 ) ) ;
#27074=AXIS2_PLACEMENT_3D ( 'NONE', #41789, #6896, #4356 ) ;
#27075=CARTESIAN_POINT ( 'NONE',  ( 116.0829010812576882, -0.01829820670803256055, -12.14321520033834290 ) ) ;
#27079=ORIENTED_EDGE ( 'NONE', *, *, #12343, .F. ) ;
#27081=ADVANCED_FACE ( 'NONE', ( #3449 ), #26, .T. ) ;
#27086=CARTESIAN_POINT ( 'NONE',  ( 110.3436608795247764, -8.938348069036489818, -9.318865927141430916 ) ) ;
#27087=CARTESIAN_POINT ( 'NONE',  ( 106.0375671295248310, 0.1403307496149613920, -13.39321520033831447 ) ) ;
#27088=CARTESIAN_POINT ( 'NONE',  ( 83.37840489759373952, -32.03678395546867819, -23.58446301471671802 ) ) ;
#27091=DIRECTION ( 'NONE',  ( -1.000000000000000000, 0.000000000000000000, 0.000000000000000000 ) ) ;
#27092=CARTESIAN_POINT ( 'NONE',  ( 114.4413952545248350, -9.868328341294098749, -15.46607636864997204 ) ) ;
#27094=CARTESIAN_POINT ( 'NONE',  ( 61.27778620743471549, -25.99489077589588604, -15.39321520033831625 ) ) ;
#27100=CARTESIAN_POINT ( 'NONE',  ( 114.0941296295247867, -4.863998795839590272, -19.15521520033831493 ) ) ;
#27110=CARTESIAN_POINT ( 'NONE',  ( 109.3018640045248304, 0.1403307496149616695, -15.46607636864997204 ) ) ;
#27134=COLOUR_RGB ( '',0.7921568627450980005, 0.8196078431372548767, 0.9333333333333333481 ) ;
#27136=VERTEX_POINT ( 'NONE', #28745 ) ;
#27138=CARTESIAN_POINT ( 'NONE',  ( 107.9822546295247889, -4.863998795839590272, -7.631215200338315796 ) ) ;
#27139=CARTESIAN_POINT ( 'NONE',  ( 106.9404577545248145, -2.791137627527939813, -18.39754474579286025 ) ) ;
#27140=CIRCLE ( 'NONE', #3113, 15.89999999999999680 ) ;
#27141=CARTESIAN_POINT ( 'NONE',  ( 87.44708369096657918, -21.99489077589588604, -7.893215200338315363 ) ) ;
#27142=B_SPLINE_CURVE_WITH_KNOTS ( 'NONE', 3,
 ( #39546, #8307, #31455, #17561, #5766, #17128, #13704, #27611, #10068, #23969, #20764, #14137 ),
 .UNSPECIFIED., .F., .F.,
 ( 4, 2, 2, 2, 2, 4 ),
 ( 0.000000000000000000, 0.1126714536578860004, 0.2901371629263108098, 0.4676028721947325661, 0.6450685814631537118, 1.000000000000000000 ),
 .UNSPECIFIED. ) ;
#27143=CARTESIAN_POINT ( 'NONE',  ( 109.6491296295247793, -4.863998795839590272, -19.15521520033831493 ) ) ;
#27147=CARTESIAN_POINT ( 'NONE',  ( 79.00611218289952831, -44.99489077589586827, -6.893215200338315363 ) ) ;
#27151=CARTESIAN_POINT ( 'NONE',  ( 105.6903015045248253, -2.477300249445798297, -7.631215200338321125 ) ) ;
#27157=EDGE_CURVE ( 'NONE', #29699, #44941, #15385, .T. ) ;
#27161=CARTESIAN_POINT ( 'NONE',  ( 114.4099712410415748, 0.7607806665037644134, -12.14321520033829316 ) ) ;
#27173=CARTESIAN_POINT ( 'NONE',  ( 112.2883483795247770, -0.7896495226426338832, -9.318865927141430916 ) ) ;
#27180=LINE ( 'NONE', #3450, #44078 ) ;
#27195=DIRECTION ( 'NONE',  ( -1.000000000000000000, 0.000000000000000000, 0.000000000000000000 ) ) ;
#27196=CARTESIAN_POINT ( 'NONE',  ( 107.8433483795247838, -0.7896495226426338832, -9.318865927141430916 ) ) ;
#27198=CARTESIAN_POINT ( 'NONE',  ( 114.1635827545248389, -6.936859964151250502, -8.388885654883777576 ) ) ;
#27199=CARTESIAN_POINT ( 'NONE',  ( 105.5513952545248060, 0.8980012041604421569, -11.00651665394454071 ) ) ;
#27211=CARTESIAN_POINT ( 'NONE',  ( 115.6220983795247861, -8.402594152722688392, -16.93181055722141792 ) ) ;
#27212=VERTEX_POINT ( 'NONE', #7530 ) ;
#27217=CARTESIAN_POINT ( 'NONE',  ( 106.8015515045248378, -6.936859964151250502, -18.39754474579286025 ) ) ;
#27218=CARTESIAN_POINT ( 'NONE',  ( 110.9687390045248350, -9.868328341294098749, -11.32035403202665869 ) ) ;
#27228=ORIENTED_EDGE ( 'NONE', *, *, #35941, .F. ) ;
#27239=DIRECTION ( 'NONE',  ( 0.000000000000000000, 1.000000000000000000, 0.000000000000000000 ) ) ;
#27241=CARTESIAN_POINT ( 'NONE',  ( 107.0099108795247815, -1.325403438956436419, -16.93181055722141792 ) ) ;
#27242=CIRCLE ( 'NONE', #11938, 5.635000000000000675 ) ;
#27243=CARTESIAN_POINT ( 'NONE',  ( 115.0664733795247798, -1.325403438956533675, -9.854619843455179051 ) ) ;
#27250=EDGE_CURVE ( 'NONE', #14709, #14403, #18022, .T. ) ;
#27251=CARTESIAN_POINT ( 'NONE',  ( 112.1874712410415924, 0.7607806665037644134, -12.14321520033829493 ) ) ;
#27253=LINE ( 'NONE', #13349, #2527 ) ;
#27259=CARTESIAN_POINT ( 'NONE',  ( 114.3719421295247827, 0.8980012041604618078, -13.39321520033831447 ) ) ;
#27260=EDGE_CURVE ( 'NONE', #34483, #21278, #17804, .T. ) ;
#27265=CARTESIAN_POINT ( 'NONE',  ( 114.4413952545248350, -9.868328341294098749, -15.46607636864997204 ) ) ;
#27269=CARTESIAN_POINT ( 'NONE',  ( 106.9404577545248145, -7.250697342233347165, -7.631215200338321125 ) ) ;
#27270=CARTESIAN_POINT ( 'NONE',  ( 117.2294421295248270, -10.07080413108645267, -4.893215200338313586 ) ) ;
#27271=CARTESIAN_POINT ( 'NONE',  ( 114.6497546295247929, -4.863998795839590272, -7.631215200338315796 ) ) ;
#27274=CARTESIAN_POINT ( 'NONE',  ( 114.7192077545248452, -7.250697342233347165, -7.631215200338321125 ) ) ;
#27284=EDGE_CURVE ( 'NONE', #28048, #970, #15390, .T. ) ;
#27286=ADVANCED_FACE ( 'NONE', ( #42649 ), #11417, .F. ) ;
#27288=CARTESIAN_POINT ( 'NONE',  ( 106.2459265045248173, -7.250697342233347165, -19.15521520033831138 ) ) ;
#27289=AXIS2_PLACEMENT_3D ( 'NONE', #8784, #9242, #22689 ) ;
#27291=CARTESIAN_POINT ( 'NONE',  ( 116.8392602215938751, -1.056629477399154915, -17.00092880501178527 ) ) ;
#27292=CARTESIAN_POINT ( 'NONE',  ( 111.6632702545248605, -10.62599879583958717, -15.77991374673208469 ) ) ;
#27298=CARTESIAN_POINT ( 'NONE',  ( 117.0059805889377316, 1.765016726092817789, -5.580912673505509680 ) ) ;
#27300=CARTESIAN_POINT ( 'NONE',  ( 105.4819421295248247, -9.868328341294093420, -13.39321520033831447 ) ) ;
#27301=DIRECTION ( 'NONE',  ( 0.000000000000000000, 0.000000000000000000, 1.000000000000000000 ) ) ;
#27313=CARTESIAN_POINT ( 'NONE',  ( 112.6356140045247827, -10.62599879583958717, -11.00651665394454604 ) ) ;
#27315=CARTESIAN_POINT ( 'NONE',  ( 106.2459265045248173, -2.791137627527939813, -8.388885654883777576 ) ) ;
#27316=CARTESIAN_POINT ( 'NONE',  ( 83.54882120758564668, -32.57787328110440939, -23.89321520033832513 ) ) ;
#27320=DIRECTION ( 'NONE',  ( 0.000000000000000000, 0.000000000000000000, -1.000000000000000000 ) ) ;
#27322=CARTESIAN_POINT ( 'NONE',  ( 108.6073327545248048, -6.936859964151250502, -8.388885654883777576 ) ) ;
#27323=EDGE_LOOP ( 'NONE', ( #32370, #44278, #41520, #35780 ) ) ;
#27324=CARTESIAN_POINT ( 'NONE',  ( 109.2294421526880086, -0.4654583522832261289, -15.91752710485221733 ) ) ;
#27327=CARTESIAN_POINT ( 'NONE',  ( 79.79010115959992788, 5.106172230548961188, -19.89321520033831447 ) ) ;
#27330=CARTESIAN_POINT ( 'NONE',  ( 114.2818621053768737, 0.3967854368539331933, -16.28112951403851838 ) ) ;
#27331=VECTOR ( 'NONE', #38213, 1000.000000000000114 ) ;
#27339=CARTESIAN_POINT ( 'NONE',  ( 116.3860827545247787, -2.477300249445798297, -19.15521520033831138 ) ) ;
#27342=CARTESIAN_POINT ( 'NONE',  ( 61.69189222814998175, -69.76310523276724496, -16.89321520033831447 ) ) ;
#27343=VERTEX_POINT ( 'NONE', #33030 ) ;
#27351=DIRECTION ( 'NONE',  ( 0.000000000000000000, -1.000000000000000000, 0.000000000000000000 ) ) ;
#27357=CARTESIAN_POINT ( 'NONE',  ( 67.69189222814998175, -49.76310523276723785, -34.89321520033831092 ) ) ;
#27366=CARTESIAN_POINT ( 'NONE',  ( 107.0099108795247815, -8.938348069036489818, -9.318865927141430916 ) ) ;
#27367=CARTESIAN_POINT ( 'NONE',  ( 105.2041296295248287, -4.863998795839590272, -8.388885654883775800 ) ) ;
#27369=CARTESIAN_POINT ( 'NONE',  ( 109.2324108795247923, -8.938348069036489818, -9.318865927141436245 ) ) ;
#27371=ORIENTED_EDGE ( 'NONE', *, *, #14186, .F. ) ;
#27375=EDGE_CURVE ( 'NONE', #27136, #34675, #39883, .T. ) ;
#27377=CARTESIAN_POINT ( 'NONE',  ( 106.3153796295248412, -4.863998795839590272, -19.15521520033831493 ) ) ;
#27396=ORIENTED_EDGE ( 'NONE', *, *, #14986, .F. ) ;
#27400=CARTESIAN_POINT ( 'NONE',  ( 108.0517077545248696, -7.250697342233347165, -7.631215200338321125 ) ) ;
#27403=ORIENTED_EDGE ( 'NONE', *, *, #12343, .T. ) ;
#27409=CARTESIAN_POINT ( 'NONE',  ( 114.8834831777918879, -0.01829820670803256055, -14.64321520033831447 ) ) ;
#27421=AXIS2_PLACEMENT_3D ( 'NONE', #25769, #39898, #11863 ) ;
#27424=CARTESIAN_POINT ( 'NONE',  ( 108.0517077545248696, -7.250697342233347165, -7.631215200338321125 ) ) ;
#27425=CARTESIAN_POINT ( 'NONE',  ( 115.2748327545248657, -6.936859964151250502, -8.388885654883777576 ) ) ;
#27426=CARTESIAN_POINT ( 'NONE',  ( 106.9404577545248145, -7.250697342233347165, -7.631215200338321125 ) ) ;
#27431=CARTESIAN_POINT ( 'NONE',  ( 112.4967077545247633, -7.250697342233347165, -7.631215200338321125 ) ) ;
#27438=CARTESIAN_POINT ( 'NONE',  ( 114.0941296295247867, -4.863998795839590272, -8.388885654883775800 ) ) ;
#27444=CARTESIAN_POINT ( 'NONE',  ( 116.5944421295247793, 0.8980012041604618078, -13.39321520033831447 ) ) ;
#27445=CARTESIAN_POINT ( 'NONE',  ( 107.2182702545248105, 0.1403307496149616695, -11.32035403202665336 ) ) ;
#27452=EDGE_CURVE ( 'NONE', #30525, #34165, #13827, .T. ) ;
#27453=LINE ( 'NONE', #41812, #28788 ) ;
#27457=VERTEX_POINT ( 'NONE', #25995 ) ;
#27463=ORIENTED_EDGE ( 'NONE', *, *, #8044, .F. ) ;
#27466=CARTESIAN_POINT ( 'NONE',  ( 113.8857702545248003, -10.62599879583958717, -15.77991374673208469 ) ) ;
#27468=CARTESIAN_POINT ( 'NONE',  ( 64.19189222814998175, -49.76310523276725206, -36.33917278160905084 ) ) ;
#27472=ORIENTED_EDGE ( 'NONE', *, *, #12948, .T. ) ;
#27484=CARTESIAN_POINT ( 'NONE',  ( 114.0246765045248196, -7.250697342233347165, -19.15521520033831138 ) ) ;
#27486=CIRCLE ( 'NONE', #12908, 15.89999999999999680 ) ;
#27488=CARTESIAN_POINT ( 'NONE',  ( 112.6119297178594536, -0.3595008806742178709, -15.96590799893915502 ) ) ;
#27489=CARTESIAN_POINT ( 'NONE',  ( 108.3295202545248657, 0.1403307496149616695, -11.32035403202665336 ) ) ;
#27490=DIRECTION ( 'NONE',  ( 0.000000000000000000, 0.000000000000000000, 1.000000000000000000 ) ) ;
#27491=CARTESIAN_POINT ( 'NONE',  ( 84.10271796608054728, -31.10763468207608895, -20.89321520033831447 ) ) ;
#27495=CARTESIAN_POINT ( 'NONE',  ( 111.6632702545248605, -10.62599879583958717, -15.77991374673208469 ) ) ;
#27498=CARTESIAN_POINT ( 'NONE',  ( 112.1114130180079798, 0.7607806665037644134, -14.64321520033833046 ) ) ;
#27513=CARTESIAN_POINT ( 'NONE',  ( 114.9970202545248412, -10.62599879583958717, -15.77991374673208469 ) ) ;
#27514=ORIENTED_EDGE ( 'NONE', *, *, #41547, .T. ) ;
#27516=LINE ( 'NONE', #41870, #4562 ) ;
#27521=CARTESIAN_POINT ( 'NONE',  ( 116.1231069823931961, 2.324083898875324738, -6.775768760798180246 ) ) ;
#27523=CARTESIAN_POINT ( 'NONE',  ( 106.9404577545248145, -2.791137627527939813, -18.39754474579286025 ) ) ;
#27524=CARTESIAN_POINT ( 'NONE',  ( 111.0001630180080809, 0.7607806665038616689, -14.64321520033831447 ) ) ;
#27527=CARTESIAN_POINT ( 'NONE',  ( 115.9923838361194868, 0.1075849324169569909, -12.14321520033831625 ) ) ;
#27537=EDGE_CURVE ( 'NONE', #5046, #18690, #8660, .T. ) ;
#27540=CARTESIAN_POINT ( 'NONE',  ( 109.1629577545248395, -7.250697342233347165, -7.631215200338321125 ) ) ;
#27541=CARTESIAN_POINT ( 'NONE',  ( 106.8015515045248378, -6.936859964151250502, -18.39754474579286025 ) ) ;
#27542=CARTESIAN_POINT ( 'NONE',  ( 115.0664733795247798, -8.938348069036489818, -17.46756447353520159 ) ) ;
#27545=DIRECTION ( 'NONE',  ( 0.000000000000000000, 0.000000000000000000, -1.000000000000000000 ) ) ;
#27547=CARTESIAN_POINT ( 'NONE',  ( 110.6214733795247867, -1.325403438956436419, -9.854619843455211026 ) ) ;
#27563=CARTESIAN_POINT ( 'NONE',  ( 116.2471765045247594, -7.250697342233347165, -19.15521520033831138 ) ) ;
#27566=FACE_OUTER_BOUND ( 'NONE', #28721, .T. ) ;
#27569=EDGE_CURVE ( 'NONE', #18860, #3693, #33479, .T. ) ;
#27574=CARTESIAN_POINT ( 'NONE',  ( 114.7192077545248594, -7.250697342233347165, -7.631215200338321125 ) ) ;
#27578=CARTESIAN_POINT ( 'NONE',  ( 78.01081489496232280, -57.59294529755612757, -1.022260109403890782 ) ) ;
#27582=FACE_OUTER_BOUND ( 'NONE', #23088, .T. ) ;
#27589=ADVANCED_FACE ( 'NONE', ( #17315 ), #13883, .F. ) ;
#27594=CARTESIAN_POINT ( 'NONE',  ( 106.2459265045248173, -7.250697342233347165, -19.15521520033831138 ) ) ;
#27595=CARTESIAN_POINT ( 'NONE',  ( 106.8015515045248378, -6.936859964151250502, -18.39754474579286025 ) ) ;
#27596=CARTESIAN_POINT ( 'NONE',  ( 105.8292077545248446, -2.791137627527939813, -18.39754474579286025 ) ) ;
#27597=CARTESIAN_POINT ( 'NONE',  ( 113.4920311052981816, 0.4930828106259610433, -12.14321520033829849 ) ) ;
#27604=CARTESIAN_POINT ( 'NONE',  ( 105.5513952545248060, 0.8980012041604421569, -11.00651665394454071 ) ) ;
#27611=CARTESIAN_POINT ( 'NONE',  ( 82.66491059565053945, -31.44298744622023989, -22.15403020929251454 ) ) ;
#27624=CARTESIAN_POINT ( 'NONE',  ( 109.4407702545248355, -10.62599879583958717, -15.77991374673208469 ) ) ;
#27627=ORIENTED_EDGE ( 'NONE', *, *, #5222, .T. ) ;
#27641=( BOUNDED_CURVE ( )  B_SPLINE_CURVE ( 2, ( #21462, #42443, #34512, #41395, #10148, #9925, #44808, #37494, #31712, #37725, #20411, #6496, #34295, #3068, #35344, #24882, #13565 ),
 .UNSPECIFIED., .F., .T. ) 
 B_SPLINE_CURVE_WITH_KNOTS ( ( 3, 2, 2, 2, 2, 2, 2, 2, 3 ),
 ( 0.3035091206787220441, 0.3125000000000000000, 0.3250000000000000111, 0.3375000000000000222, 0.3499999999999999778, 0.3624999999999999889, 0.3750000000000000000, 0.3875000000000000111, 0.3964908793212780225 ),
 .UNSPECIFIED. ) 
 CURVE ( )  GEOMETRIC_REPRESENTATION_ITEM ( )  RATIONAL_B_SPLINE_CURVE ( ( 0.9692594319298230010, 0.9452488050343769155, 1.000000000000000000, 0.9238795325112869605, 1.000000000000000000, 0.9238795325112869605, 1.000000000000000000, 0.9238795325112869605, 1.000000000000000000, 0.9238795325112869605, 1.000000000000000000, 0.9238795325112869605, 1.000000000000000000, 0.9238795325112869605, 1.000000000000000000, 0.9452488050343769155, 0.9692594319298220018 ) ) 
 REPRESENTATION_ITEM ( '' )  );
#27647=CARTESIAN_POINT ( 'NONE',  ( 109.0240515045248202, -2.477300249445798297, -7.631215200338321125 ) ) ;
#27648=CARTESIAN_POINT ( 'NONE',  ( 109.5796765045248122, -2.791137627527939813, -8.388885654883777576 ) ) ;
#27649=CARTESIAN_POINT ( 'NONE',  ( 106.7320983795247855, -0.7896495226426338832, -9.318865927141430916 ) ) ;
#27652=VERTEX_POINT ( 'NONE', #3607 ) ;
#27654=CARTESIAN_POINT ( 'NONE',  ( 109.7880358795247986, -0.7896495226426338832, -17.46756447353520159 ) ) ;
#27662=CARTESIAN_POINT ( 'NONE',  ( 106.1070202545248407, -10.62599879583958717, -15.77991374673208469 ) ) ;
#27664=CYLINDRICAL_SURFACE ( 'NONE', #465, 4.500000000000003553 ) ;
#27667=AXIS2_PLACEMENT_3D ( 'NONE', #17902, #42969, #3757 ) ;
#27668=CARTESIAN_POINT ( 'NONE',  ( 115.8999108795247821, -8.938348069036489818, -9.318865927141430916 ) ) ;
#27669=CARTESIAN_POINT ( 'NONE',  ( 108.1211608795247798, -1.325403438956436419, -16.93181055722141792 ) ) ;
#27682=EDGE_LOOP ( 'NONE', ( #16729, #24933, #16453, #12991 ) ) ;
#27690=CARTESIAN_POINT ( 'NONE',  ( 113.5385046295247804, -4.863998795839590272, -7.631215200338315796 ) ) ;
#27692=CARTESIAN_POINT ( 'NONE',  ( 115.9456797178594343, -0.3595008806742178709, -15.96590799893915857 ) ) ;
#27699=VECTOR ( 'NONE', #13446, 1000.000000000000000 ) ;
#27702=ADVANCED_FACE ( 'NONE', ( #10550, #38339 ), #34468, .T. ) ;
#27708=CARTESIAN_POINT ( 'NONE',  ( 106.8015515045248378, -6.936859964151250502, -18.39754474579286025 ) ) ;
#27713=CARTESIAN_POINT ( 'NONE',  ( 110.9687390045248350, -9.868328341294098749, -11.32035403202665869 ) ) ;
#27717=CARTESIAN_POINT ( 'NONE',  ( 107.6349890045248401, 0.8980012041604421569, -15.77991374673208469 ) ) ;
#27719=CARTESIAN_POINT ( 'NONE',  ( 111.1770983795247787, -0.7896495226426338832, -9.318865927141430916 ) ) ;
#27737=CARTESIAN_POINT ( 'NONE',  ( 114.1635827545248389, -2.477300249445798297, -19.15521520033831138 ) ) ;
#27740=DIRECTION ( 'NONE',  ( -0.9970811988817437355, 0.07634843047859309062, 0.000000000000000000 ) ) ;
#27748=CARTESIAN_POINT ( 'NONE',  ( 114.3024890045248156, -9.868328341294098749, -11.32035403202665869 ) ) ;
#27761=CARTESIAN_POINT ( 'NONE',  ( 105.5513952545248060, -9.868328341294098749, -15.46607636864997204 ) ) ;
#27762=CARTESIAN_POINT ( 'NONE',  ( 111.5938171295247940, -10.62599879583958540, -13.39321520033831447 ) ) ;
#27765=CARTESIAN_POINT ( 'NONE',  ( 116.5944421295247793, -4.863998795839590272, -13.39321520033831447 ) ) ;
#27767=CARTESIAN_POINT ( 'NONE',  ( 107.5655358795247736, -8.402594152722688392, -9.854619843455216355 ) ) ;
#27774=CARTESIAN_POINT ( 'NONE',  ( 113.5385046295247804, -4.863998795839590272, -7.631215200338315796 ) ) ;
#27781=CARTESIAN_POINT ( 'NONE',  ( 106.5237390045248418, -9.868328341294098749, -11.32035403202665869 ) ) ;
#27783=DIRECTION ( 'NONE',  ( 0.000000000000000000, 0.000000000000000000, -1.000000000000000000 ) ) ;
#27786=ADVANCED_FACE ( 'NONE', ( #25792 ), #18729, .T. ) ;
#27790=CARTESIAN_POINT ( 'NONE',  ( 113.9552233795247815, -8.938348069036489818, -17.46756447353520159 ) ) ;
#27791=AXIS2_PLACEMENT_3D ( 'NONE', #44710, #5930, #34411 ) ;
#27804=ORIENTED_EDGE ( 'NONE', *, *, #23359, .F. ) ;
#27806=CARTESIAN_POINT ( 'NONE',  ( 106.7320983795247855, -0.7896495226426338832, -9.318865927141430916 ) ) ;
#27809=CARTESIAN_POINT ( 'NONE',  ( 105.6208483795248299, -8.402594152722688392, -16.93181055722141792 ) ) ;
#27810=CIRCLE ( 'NONE', #8151, 2.000000000000001776 ) ;
#27818=DIRECTION ( 'NONE',  ( -1.156482317317869950E-15, -1.000000000000000000, 0.000000000000000000 ) ) ;
#27821=CARTESIAN_POINT ( 'NONE',  ( 111.2465515045248168, -6.936859964151250502, -18.39754474579286025 ) ) ;
#27822=CARTESIAN_POINT ( 'NONE',  ( 117.2294421295247844, -10.76310523276723785, -21.89255013987451548 ) ) ;
#27831=CARTESIAN_POINT ( 'NONE',  ( 112.7491510812576934, -0.01829820670803256055, -12.14321520033831625 ) ) ;
#27833=ORIENTED_EDGE ( 'NONE', *, *, #23542, .F. ) ;
#27835=CARTESIAN_POINT ( 'NONE',  ( 116.5946626450759851, -9.863530430156441042, -13.31021735937817851 ) ) ;
#27842=EDGE_CURVE ( 'NONE', #40576, #7297, #7672, .T. ) ;
#27846=CARTESIAN_POINT ( 'NONE',  ( 108.9545983795247821, -0.7896495226426338832, -9.318865927141430916 ) ) ;
#27849=ORIENTED_EDGE ( 'NONE', *, *, #9440, .T. ) ;
#27853=CARTESIAN_POINT ( 'NONE',  ( 79.79010115959992788, 5.106172230548961188, -4.893215200338314474 ) ) ;
#27857=CIRCLE ( 'NONE', #29307, 0.9999999999999952260 ) ;
#27863=CARTESIAN_POINT ( 'NONE',  ( 70.55229225240181279, -24.89194276641628889, -5.467054258871676176 ) ) ;
#27865=VERTEX_POINT ( 'NONE', #13639 ) ;
#27867=CARTESIAN_POINT ( 'NONE',  ( 106.3848327545248651, -2.477300249445798297, -19.15521520033831138 ) ) ;
#27868=CARTESIAN_POINT ( 'NONE',  ( 107.4266296295248821, -4.863998795839590272, -8.388885654883775800 ) ) ;
#27869=CARTESIAN_POINT ( 'NONE',  ( 106.4542858795248179, -0.7896495226426338832, -17.46756447353520159 ) ) ;
#27874=CARTESIAN_POINT ( 'NONE',  ( 111.1770983795247787, -0.7896495226426338832, -9.318865927141430916 ) ) ;
#27881=CARTESIAN_POINT ( 'NONE',  ( 114.9275671295247889, -10.62599879583958540, -13.39321520033831447 ) ) ;
#27882=CARTESIAN_POINT ( 'NONE',  ( 106.1764733795248219, -8.938348069036489818, -17.46756447353520159 ) ) ;
#27884=DIRECTION ( 'NONE',  ( -1.387778780781445478E-15, -1.000000000000000000, 0.000000000000000000 ) ) ;
#27888=CARTESIAN_POINT ( 'NONE',  ( 114.5803015045248117, -2.477300249445798297, -7.631215200338321125 ) ) ;
#27889=CARTESIAN_POINT ( 'NONE',  ( 106.8015515045248378, -6.936859964151250502, -18.39754474579286025 ) ) ;
#27902=CARTESIAN_POINT ( 'NONE',  ( 111.9410827545248708, -6.936859964151250502, -8.388885654883777576 ) ) ;
#27907=( BOUNDED_CURVE ( )  B_SPLINE_CURVE ( 3, ( #6220, #12851, #13072, #30169 ),
 .UNSPECIFIED., .F., .T. ) 
 B_SPLINE_CURVE_WITH_KNOTS ( ( 4, 4 ),
 ( 4.712388980384689674, 5.355890089177970381 ),
 .UNSPECIFIED. ) 
 CURVE ( )  GEOMETRIC_REPRESENTATION_ITEM ( )  RATIONAL_B_SPLINE_CURVE ( ( 1.000000000000000000, 0.9657888653670090306, 0.9657888653670090306, 1.000000000000000000 ) ) 
 REPRESENTATION_ITEM ( '' )  );
#27914=CARTESIAN_POINT ( 'NONE',  ( 113.3995983795247895, -0.7896495226426338832, -9.318865927141430916 ) ) ;
#27924=VECTOR ( 'NONE', #11348, 1000.000000000000000 ) ;
#27925=CARTESIAN_POINT ( 'NONE',  ( 66.38809756183205479, -36.79083284667497367, -4.893215200338314474 ) ) ;
#27931=CARTESIAN_POINT ( 'NONE',  ( 110.0658483795247804, -0.7896495226426338832, -9.318865927141430916 ) ) ;
#27936=CARTESIAN_POINT ( 'NONE',  ( 108.1906140045248463, 0.1403307496149616695, -15.46607636864997204 ) ) ;
#27937=CARTESIAN_POINT ( 'NONE',  ( 111.3160046295247838, -4.863998795839590272, -7.631215200338315796 ) ) ;
#27938=CARTESIAN_POINT ( 'NONE',  ( 109.2294420763164453, -8.136444762514427609, -17.62486350101510624 ) ) ;
#27940=DIRECTION ( 'NONE',  ( 0.9970811988817434024, -0.07634843047859724008, 9.125038414728753042E-18 ) ) ;
#27941=CARTESIAN_POINT ( 'NONE',  ( 117.0806140045248185, 0.1403307496149616695, -15.46607636864997204 ) ) ;
#27942=CARTESIAN_POINT ( 'NONE',  ( 108.3295202545248657, -10.62599879583958717, -15.77991374673208469 ) ) ;
#27960=EDGE_CURVE ( 'NONE', #424, #11479, #15319, .T. ) ;
#27962=CARTESIAN_POINT ( 'NONE',  ( 113.1217858795247935, -0.7896495226426338832, -17.46756447353520159 ) ) ;
#27965=CARTESIAN_POINT ( 'NONE',  ( 143.3676850761856940, -64.41823023953081417, -19.25521411788945514 ) ) ;
#27972=CARTESIAN_POINT ( 'NONE',  ( 115.9693640045247776, 0.1403307496149616695, -15.46607636864997204 ) ) ;
#27974=AXIS2_PLACEMENT_3D ( 'NONE', #31038, #38101, #41548 ) ;
#27977=ADVANCED_FACE ( 'NONE', ( #41241 ), #41016, .T. ) ;
#27988=CARTESIAN_POINT ( 'NONE',  ( 111.4549108795247747, -8.938348069036489818, -9.318865927141430916 ) ) ;
#27992=CARTESIAN_POINT ( 'NONE',  ( 109.2294421297036280, -3.476265968579914212, -8.054548070311122743 ) ) ;
#27994=CARTESIAN_POINT ( 'NONE',  ( 107.0099108795247815, -1.325403438956436419, -16.93181055722141792 ) ) ;
#27995=CARTESIAN_POINT ( 'NONE',  ( 117.2294421295247844, 1.035107641088057973, -21.72657133228191739 ) ) ;
#27998=CARTESIAN_POINT ( 'NONE',  ( 110.6909265045248247, -7.250697342233347165, -19.15521520033831138 ) ) ;
#28001=CARTESIAN_POINT ( 'NONE',  ( 70.36267391504962632, -5.685877709920933221, -19.39321520033831447 ) ) ;
#28008=CARTESIAN_POINT ( 'NONE',  ( 108.0517077545248696, -2.791137627527939813, -18.39754474579286025 ) ) ;
#28011=CARTESIAN_POINT ( 'NONE',  ( 69.69189222814998175, -41.76310523276723785, -19.39321520033831447 ) ) ;
#28016=VERTEX_POINT ( 'NONE', #20484 ) ;
#28017=CARTESIAN_POINT ( 'NONE',  ( 114.5108483795247878, -0.7896495226426338832, -9.318865927141430916 ) ) ;
#28033=ORIENTED_EDGE ( 'NONE', *, *, #5958, .F. ) ;
#28035=CARTESIAN_POINT ( 'NONE',  ( 109.2324108795247923, -8.938348069036489818, -9.318865927141430916 ) ) ;
#28037=CARTESIAN_POINT ( 'NONE',  ( 114.8344297178593507, -0.3595008806742178709, -15.96590799893915857 ) ) ;
#28043=FACE_OUTER_BOUND ( 'NONE', #13269, .T. ) ;
#28046=CARTESIAN_POINT ( 'NONE',  ( 111.7327233795247849, -1.325403438956436419, -9.854619843455211026 ) ) ;
#28048=VERTEX_POINT ( 'NONE', #24128 ) ;
#28059=AXIS2_PLACEMENT_3D ( 'NONE', #36465, #15959, #36906 ) ;
#28067=CARTESIAN_POINT ( 'NONE',  ( 108.6073327545248048, -2.477300249445798297, -19.15521520033831138 ) ) ;
#28071=ORIENTED_EDGE ( 'NONE', *, *, #37975, .F. ) ;
#28074=CARTESIAN_POINT ( 'NONE',  ( 79.40190946915554093, 5.047224606967246174, -20.48130549182737425 ) ) ;
#28087=CARTESIAN_POINT ( 'NONE',  ( 85.75809888461174069, -18.45227461768569199, -7.393215200338315363 ) ) ;
#28089=CARTESIAN_POINT ( 'NONE',  ( 113.0523327545247838, -6.936859964151250502, -8.388885654883777576 ) ) ;
#28090=CARTESIAN_POINT ( 'NONE',  ( 109.9269421295247753, -9.868328341294093420, -13.39321520033831447 ) ) ;
#28091=CARTESIAN_POINT ( 'NONE',  ( 113.4690515045247992, -6.936859964151250502, -18.39754474579286025 ) ) ;
#28097=CARTESIAN_POINT ( 'NONE',  ( 110.0658483795247804, -0.7896495226426338832, -9.318865927141430916 ) ) ;
#28098=DIRECTION ( 'NONE',  ( -1.156482317317869950E-15, -1.000000000000000000, 0.000000000000000000 ) ) ;
#28100=EDGE_CURVE ( 'NONE', #11967, #8479, #37337, .T. ) ;
#28106=CARTESIAN_POINT ( 'NONE',  ( 114.1635827545248389, -2.477300249445798297, -19.15521520033831138 ) ) ;
#28107=CARTESIAN_POINT ( 'NONE',  ( 105.7597546295248350, -4.863998795839590272, -7.631215200338315796 ) ) ;
#28112=CARTESIAN_POINT ( 'NONE',  ( 114.8581140045248361, -10.62599879583958717, -11.00651665394454604 ) ) ;
#28113=CARTESIAN_POINT ( 'NONE',  ( 107.0099108795247815, -1.325403438956436419, -16.93181055722141792 ) ) ;
#28117=ORIENTED_EDGE ( 'NONE', *, *, #37268, .T. ) ;
#28121=EDGE_LOOP ( 'NONE', ( #29558, #44552, #28572, #38982 ) ) ;
#28123=CARTESIAN_POINT ( 'NONE',  ( 106.8015515045248378, -2.477300249445798297, -7.631215200338321125 ) ) ;
#28124=CARTESIAN_POINT ( 'NONE',  ( 110.5520202545248054, 0.1403307496149616695, -11.32035403202665336 ) ) ;
#28125=EDGE_CURVE ( 'NONE', #35850, #23757, #38903, .T. ) ;
#28135=EDGE_CURVE ( 'NONE', #3445, #11630, #28436, .T. ) ;
#28136=CARTESIAN_POINT ( 'NONE',  ( 116.1777233795247781, -8.938348069036489818, -17.46756447353520159 ) ) ;
#28141=ORIENTED_EDGE ( 'NONE', *, *, #36889, .F. ) ;
#28143=DIRECTION ( 'NONE',  ( 0.000000000000000000, 0.5905882410490339574, 0.8069730661766899571 ) ) ;
#28144=CARTESIAN_POINT ( 'NONE',  ( 65.66749702063913219, -36.20550398600038022, -5.467054258871666406 ) ) ;
#28148=VERTEX_POINT ( 'NONE', #42798 ) ;
#28150=CARTESIAN_POINT ( 'NONE',  ( 115.8759982281897862, 0.3371508018708627152, -21.89321520033831447 ) ) ;
#28151=CARTESIAN_POINT ( 'NONE',  ( 109.9269421295247753, 0.8980012041604618078, -13.39321520033831447 ) ) ;
#28157=CARTESIAN_POINT ( 'NONE',  ( 108.3989733795248753, -1.325403438956436419, -9.854619843455211026 ) ) ;
#28160=CARTESIAN_POINT ( 'NONE',  ( 109.2295290894191311, -5.098491836473954208, -18.58823644444565204 ) ) ;
#28162=CARTESIAN_POINT ( 'NONE',  ( 105.6208483795248299, -0.7896495226426338832, -9.318865927141430916 ) ) ;
#28164=CARTESIAN_POINT ( 'NONE',  ( 111.3160046295247838, -4.863998795839590272, -7.631215200338315796 ) ) ;
#28179=( BOUNDED_CURVE ( )  B_SPLINE_CURVE ( 2, ( #14567, #28037, #20967, #18212, #17544, #11379, #42390, #11155, #39182, #21634, #38493, #7946, #7721, #21857, #31437, #7268, #4293 ),
 .UNSPECIFIED., .F., .T. ) 
 B_SPLINE_CURVE_WITH_KNOTS ( ( 3, 2, 2, 2, 2, 2, 2, 2, 3 ),
 ( 0.1040431156034945931, 0.1125000000000000028, 0.1250000000000000000, 0.1375000000000000111, 0.1499999999999999944, 0.1625000000000000056, 0.1749999999999999889, 0.1875000000000000000, 0.1959568843965054930 ),
 .UNSPECIFIED. ) 
 CURVE ( )  GEOMETRIC_REPRESENTATION_ITEM ( )  RATIONAL_B_SPLINE_CURVE ( ( 0.9666851417651740608, 0.9485006404992000206, 1.000000000000000000, 0.9238795325112869605, 1.000000000000000000, 0.9238795325112869605, 1.000000000000000000, 0.9238795325112869605, 1.000000000000000000, 0.9238795325112869605, 1.000000000000000000, 0.9238795325112869605, 1.000000000000000000, 0.9238795325112869605, 1.000000000000000000, 0.9485006404991980222, 0.9666851417651760592 ) ) 
 REPRESENTATION_ITEM ( '' )  );
#28183=CARTESIAN_POINT ( 'NONE',  ( 107.7738952545248310, 0.8980012041604421569, -11.00651665394454071 ) ) ;
#28192=ADVANCED_FACE ( 'NONE', ( #38676 ), #24784, .T. ) ;
#28194=CARTESIAN_POINT ( 'NONE',  ( 116.3860827545247787, -6.936859964151250502, -8.388885654883777576 ) ) ;
#28199=B_SPLINE_CURVE_WITH_KNOTS ( 'NONE', 3,
 ( #31268, #30832, #41, #13954, #16937, #35116, #17379, #21239, #17597, #34677 ),
 .UNSPECIFIED., .F., .F.,
 ( 4, 3, 3, 4 ),
 ( 0.000000000000000000, 1.415135068341309975E-06, 2.830270136676894854E-06, 5.507324299894169413E-06 ),
 .UNSPECIFIED. ) ;
#28206=CARTESIAN_POINT ( 'NONE',  ( 114.4413952545248350, -9.868328341294098749, -15.46607636864997204 ) ) ;
#28210=CARTESIAN_POINT ( 'NONE',  ( 114.5108483795247878, -0.7896495226426338832, -9.318865927141430916 ) ) ;
#28217=CARTESIAN_POINT ( 'NONE',  ( 111.3160046295247838, -4.863998795839590272, -18.39754474579285315 ) ) ;
#28218=DIRECTION ( 'NONE',  ( 0.000000000000000000, 0.000000000000000000, 1.000000000000000000 ) ) ;
#28221=CARTESIAN_POINT ( 'NONE',  ( 111.4549108795247747, -8.938348069036489818, -9.318865927141430916 ) ) ;
#28223=VERTEX_POINT ( 'NONE', #18401 ) ;
#28232=CARTESIAN_POINT ( 'NONE',  ( 113.6774108795247997, -8.938348069036489818, -9.318865927141430916 ) ) ;
#28239=CARTESIAN_POINT ( 'NONE',  ( 114.7886608795247696, -8.938348069036489818, -9.318865927141430916 ) ) ;
#28244=CYLINDRICAL_SURFACE ( 'NONE', #6970, 5.132259260909266985 ) ;
#28248=CARTESIAN_POINT ( 'NONE',  ( 117.0049627575976814, 0.4002175711165650851, -14.64321520033831447 ) ) ;
#28254=ORIENTED_EDGE ( 'NONE', *, *, #8425, .T. ) ;
#28256=CARTESIAN_POINT ( 'NONE',  ( 114.3024890045248156, -9.868328341294098749, -11.32035403202665869 ) ) ;
#28257=DIRECTION ( 'NONE',  ( 0.000000000000000000, 0.000000000000000000, 1.000000000000000000 ) ) ;
#28268=CARTESIAN_POINT ( 'NONE',  ( 112.0105358795248804, -8.402594152722688392, -9.854619843455216355 ) ) ;
#28282=ORIENTED_EDGE ( 'NONE', *, *, #27007, .T. ) ;
#28283=CARTESIAN_POINT ( 'NONE',  ( 116.5976908158778826, -9.866790291921139655, -13.46630915925490690 ) ) ;
#28289=CARTESIAN_POINT ( 'NONE',  ( 109.5796765045248122, -7.250697342233347165, -19.15521520033831138 ) ) ;
#28291=ORIENTED_EDGE ( 'NONE', *, *, #35301, .F. ) ;
#28293=DIRECTION ( 'NONE',  ( -1.000000000000000000, 0.000000000000000000, 0.000000000000000000 ) ) ;
#28305=ORIENTED_EDGE ( 'NONE', *, *, #14186, .T. ) ;
#28308=CARTESIAN_POINT ( 'NONE',  ( 112.7050671295247923, 0.1403307496149613920, -13.39321520033831447 ) ) ;
#28309=CARTESIAN_POINT ( 'NONE',  ( 106.8015515045248378, -6.936859964151250502, -18.39754474579286025 ) ) ;
#28310=CARTESIAN_POINT ( 'NONE',  ( 113.5385046295247804, -4.863998795839590272, -18.39754474579285315 ) ) ;
#28315=CARTESIAN_POINT ( 'NONE',  ( 111.5938171295247940, -10.62599879583958540, -13.39321520033831447 ) ) ;
#28316=FACE_BOUND ( 'NONE', #30306, .T. ) ;
#28319=CARTESIAN_POINT ( 'NONE',  ( 79.14411413026581954, 4.892312988188566081, -5.897268129732760045 ) ) ;
#28321=FACE_OUTER_BOUND ( 'NONE', #1572, .T. ) ;
#28322=CARTESIAN_POINT ( 'NONE',  ( 111.8021765045248372, -2.791137627527939813, -8.388885654883777576 ) ) ;
#28327=CARTESIAN_POINT ( 'NONE',  ( 113.9552233795247815, -8.938348069036489818, -17.46756447353520159 ) ) ;
#28334=CIRCLE ( 'NONE', #14493, 2.000000000000001776 ) ;
#28340=CARTESIAN_POINT ( 'NONE',  ( 111.3160046295247838, -4.863998795839590272, -18.39754474579285315 ) ) ;
#28346=EDGE_CURVE ( 'NONE', #25605, #20709, #35705, .T. ) ;
#28351=CARTESIAN_POINT ( 'NONE',  ( 109.3018640045248304, -10.62599879583958717, -11.00651665394454604 ) ) ;
#28359=CARTESIAN_POINT ( 'NONE',  ( 71.36400868967236022, -24.42718413923373788, -4.893215200338314474 ) ) ;
#28360=CARTESIAN_POINT ( 'NONE',  ( 115.8999108795247821, -8.938348069036489818, -9.318865927141430916 ) ) ;
#28366=CARTESIAN_POINT ( 'NONE',  ( 87.44708369096657918, -21.99489077589588604, -7.893215200338315363 ) ) ;
#28367=CARTESIAN_POINT ( 'NONE',  ( 112.1494421295248003, 0.8980012041604618078, -13.39321520033831447 ) ) ;
#28372=CARTESIAN_POINT ( 'NONE',  ( 109.3713171295247832, 0.1403307496149613920, -13.39321520033831447 ) ) ;
#28373=ADVANCED_FACE ( 'NONE', ( #28886 ), #21589, .T. ) ;
#28375=CARTESIAN_POINT ( 'NONE',  ( 116.2471765045247594, -7.250697342233347165, -19.15521520033830427 ) ) ;
#28376=CARTESIAN_POINT ( 'NONE',  ( 109.2294861558825119, -6.900259341933140611, -18.27081374760126664 ) ) ;
#28379=CARTESIAN_POINT ( 'NONE',  ( 115.4831921295247952, -9.868328341294093420, -13.39321520033831447 ) ) ;
#28380=CARTESIAN_POINT ( 'NONE',  ( 110.7603796295247918, -4.863998795839590272, -19.15521520033831493 ) ) ;
#28384=EDGE_CURVE ( 'NONE', #20709, #39064, #3227, .T. ) ;
#28399=CARTESIAN_POINT ( 'NONE',  ( 109.1629577545248395, -7.250697342233347165, -7.631215200338321125 ) ) ;
#28401=EDGE_CURVE ( 'NONE', #16340, #14378, #32776, .T. ) ;
#28410=CARTESIAN_POINT ( 'NONE',  ( 69.69189222814998175, -41.76310523276723785, -4.893215200338314474 ) ) ;
#28411=CARTESIAN_POINT ( 'NONE',  ( 112.2841521944299785, 0.6269505268395592079, -12.14321520033829849 ) ) ;
#28412=CARTESIAN_POINT ( 'NONE',  ( 115.8304577545247582, -2.791137627527939813, -18.39754474579286025 ) ) ;
#28424=CARTESIAN_POINT ( 'NONE',  ( 113.5385046295247804, -4.863998795839590272, -18.39754474579285315 ) ) ;
#28427=CARTESIAN_POINT ( 'NONE',  ( 85.92326454629504440, -27.42010911645014204, -8.655686125604109549 ) ) ;
#28428=CARTESIAN_POINT ( 'NONE',  ( 114.7886608795247696, -8.938348069036489818, -9.318865927141430916 ) ) ;
#28433=CARTESIAN_POINT ( 'NONE',  ( 109.2294400832953301, -1.120989073033315409, -9.512730530502590653 ) ) ;
#28435=CARTESIAN_POINT ( 'NONE',  ( 113.6774108795247997, -8.938348069036489818, -9.318865927141430916 ) ) ;
#28436=LINE ( 'NONE', #11108, #22567 ) ;
#28439=CARTESIAN_POINT ( 'NONE',  ( 113.2606921295247702, 0.8980012041604618078, -13.39321520033831447 ) ) ;
#28453=CARTESIAN_POINT ( 'NONE',  ( 112.9828796295247884, -4.863998795839590272, -19.15521520033831493 ) ) ;
#28456=CARTESIAN_POINT ( 'NONE',  ( 143.3676850761856940, -49.76310523276723785, -40.89321520033831092 ) ) ;
#28463=CARTESIAN_POINT ( 'NONE',  ( 107.6349890045248401, -9.868328341294098749, -11.32035403202665869 ) ) ;
#28468=CARTESIAN_POINT ( 'NONE',  ( 64.61935771200890599, -37.86087448816891765, -4.893215200338314474 ) ) ;
#28471=DIRECTION ( 'NONE',  ( -1.000000000000000000, 0.000000000000000000, 0.000000000000000000 ) ) ;
#28484=CARTESIAN_POINT ( 'NONE',  ( 114.6497546295247929, -4.863998795839590272, -18.39754474579285315 ) ) ;
#28495=CARTESIAN_POINT ( 'NONE',  ( 114.0941296295247867, -4.863998795839590272, -8.388885654883775800 ) ) ;
#28500=AXIS2_PLACEMENT_3D ( 'NONE', #16302, #9451, #22676 ) ;
#28510=EDGE_CURVE ( 'NONE', #6998, #30513, #40419, .T. ) ;
#28511=CARTESIAN_POINT ( 'NONE',  ( 115.7610046295247912, -4.863998795839590272, -18.39754474579285315 ) ) ;
#28533=CARTESIAN_POINT ( 'NONE',  ( 69.16666358353634791, -25.68530218154914024, -5.871463680831265464 ) ) ;
#28536=ORIENTED_EDGE ( 'NONE', *, *, #1621, .T. ) ;
#28538=CARTESIAN_POINT ( 'NONE',  ( 115.2748327545248657, -2.477300249445798297, -19.15521520033831138 ) ) ;
#28539=CARTESIAN_POINT ( 'NONE',  ( 113.1912390045248031, -9.868328341294098749, -11.32035403202665869 ) ) ;
#28541=CARTESIAN_POINT ( 'NONE',  ( 113.6774108795247997, -1.325403438956436419, -16.93181055722141792 ) ) ;
#28547=CARTESIAN_POINT ( 'NONE',  ( 109.3713171295247832, -10.62599879583958540, -13.39321520033831447 ) ) ;
#28551=CARTESIAN_POINT ( 'NONE',  ( 79.26207964172509435, 4.977544347528738200, -6.087841491724327980 ) ) ;
#28553=CARTESIAN_POINT ( 'NONE',  ( 115.4137390045248566, 0.8980012041604421569, -15.77991374673208469 ) ) ;
#28554=CARTESIAN_POINT ( 'NONE',  ( 112.9828796295247884, -4.863998795839590272, -8.388885654883775800 ) ) ;
#28559=CARTESIAN_POINT ( 'NONE',  ( 61.69189222814998175, -60.26310523276723785, -29.64311716074571379 ) ) ;
#28567=ORIENTED_EDGE ( 'NONE', *, *, #24189, .F. ) ;
#28570=CARTESIAN_POINT ( 'NONE',  ( 110.1353015045248469, -6.936859964151250502, -18.39754474579286025 ) ) ;
#28572=ORIENTED_EDGE ( 'NONE', *, *, #34004, .T. ) ;
#28576=EDGE_CURVE ( 'NONE', #15833, #24095, #41184, .T. ) ;
#28581=DIRECTION ( 'NONE',  ( 0.000000000000000000, 0.000000000000000000, 1.000000000000000000 ) ) ;
#28583=CARTESIAN_POINT ( 'NONE',  ( 111.1770983795247787, -0.7896495226426338832, -9.318865927141430916 ) ) ;
#28590=CARTESIAN_POINT ( 'NONE',  ( 115.5526452545247622, 0.8980012041604421569, -11.00651665394454071 ) ) ;
#28591=FACE_OUTER_BOUND ( 'NONE', #707, .T. ) ;
#28597=CARTESIAN_POINT ( 'NONE',  ( 110.4825671295247815, -10.62599879583958540, -13.39321520033831447 ) ) ;
#28605=VECTOR ( 'NONE', #14338, 1000.000000000000000 ) ;
#28607=CARTESIAN_POINT ( 'NONE',  ( 109.2294398423855739, -8.045347437686777070, -17.68788261941902107 ) ) ;
#28610=CARTESIAN_POINT ( 'NONE',  ( 116.4555358795247884, -8.402594152722688392, -9.854619843455216355 ) ) ;
#28611=CARTESIAN_POINT ( 'NONE',  ( 114.7192077545248594, -2.791137627527939813, -18.39754474579286025 ) ) ;
#28627=CARTESIAN_POINT ( 'NONE',  ( 109.5102233795247884, -8.938348069036489818, -17.46756447353520159 ) ) ;
#28629=CARTESIAN_POINT ( 'NONE',  ( 116.8209981608379877, 0.3867979994853637526, -14.64321520033831447 ) ) ;
#28630=EDGE_CURVE ( 'NONE', #37481, #12500, #6744, .T. ) ;
#28631=CARTESIAN_POINT ( 'NONE',  ( 112.8439733795247832, -1.325403438956436419, -9.854619843455211026 ) ) ;
#28638=CARTESIAN_POINT ( 'NONE',  ( 112.1494421295248003, -9.868328341294093420, -13.39321520033831447 ) ) ;
#28650=CARTESIAN_POINT ( 'NONE',  ( 116.3166296295247832, -4.863998795839590272, -8.388885654883775800 ) ) ;
#28654=CARTESIAN_POINT ( 'NONE',  ( 85.94313020268559455, -27.37200725933698564, -8.637542561674017350 ) ) ;
#28655=CARTESIAN_POINT ( 'NONE',  ( 113.1217858795247935, -0.7896495226426338832, -17.46756447353520159 ) ) ;
#28657=VECTOR ( 'NONE', #165, 1000.000000000000227 ) ;
#28659=CARTESIAN_POINT ( 'NONE',  ( 115.7573452706806876, 0.3193521225029610777, -14.64321520033831447 ) ) ;
#28660=CARTESIAN_POINT ( 'NONE',  ( 109.2294408980514930, -1.069172662007336960, -9.568136978171825291 ) ) ;
#28662=CARTESIAN_POINT ( 'NONE',  ( 115.1359265045248605, -7.250697342233347165, -19.15521520033831138 ) ) ;
#28664=CARTESIAN_POINT ( 'NONE',  ( 117.2294421295247986, 1.129870453897466431, -21.68537999533008076 ) ) ;
#28667=CARTESIAN_POINT ( 'NONE',  ( 109.8574890045247940, 0.8980012041604421569, -15.77991374673208469 ) ) ;
#28671=ORIENTED_EDGE ( 'NONE', *, *, #15081, .T. ) ;
#28679=CARTESIAN_POINT ( 'NONE',  ( 114.5108483795247878, -0.7896495226426338832, -9.318865927141430916 ) ) ;
#28683=CARTESIAN_POINT ( 'NONE',  ( 61.76986277844709861, -39.32091226840162079, -19.39321520033831447 ) ) ;
#28685=CLOSED_SHELL ( 'NONE', ( #9157, #29468, #30926, #40077, #5849, #30615, #5283, #44746, #44936, #17153, #18869, #38709, #12811, #44004, #14687, #37594, #11085, #44520, #33422, #37985, #13870, #8589, #42033, #27786, #20118, #28373, #44569, #7918, #26046, #32050, #1057, #19871, #740, #35961, #27589, #45130, #34117, #21958, #17099, #18360, #27977, #6108, #28192, #36121, #27286, #25171, #1906, #39580, #26874, #43120, #20833, #22691, #28918, #16676, #5583, #26155, #30711, #7350, #38479, #27702, #21390, #42839, #14742, #17277, #29763, #31176, #15584, #33416, #3587, #21776, #38738, #4961, #34374, #44952, #14327, #36513, #5507, #29782, #1424, #28972, #2417, #31209, #37396, #38405, #24463, #32607, #23660, #236, #22884, #11913, #42610, #17353, #42023, #18483, #14393, #21992, #12483, #14713, #13694, #16155, #8312, #12870, #26548, #40343, #25603, #15333, #30423, #24480, #32268, #2242, #42582, #37930, #2813, #33464, #33108, #3824, #43747, #30860, #16160, #29733, #42904, #40401, #6374, #19929, #12882, #11531, #31728, #25629, #5031, #42361, #42284, #27081, #19247, #25032, #20464 ) ) ;
#28708=CARTESIAN_POINT ( 'NONE',  ( 114.0941296295247867, -4.863998795839590272, -8.388885654883775800 ) ) ;
#28709=CARTESIAN_POINT ( 'NONE',  ( 78.69189222814998175, -46.76310523276723785, -6.893215200338315363 ) ) ;
#28718=EDGE_CURVE ( 'NONE', #408, #21278, #40957, .T. ) ;
#28720=CARTESIAN_POINT ( 'NONE',  ( 113.5385046295247804, -4.863998795839590272, -18.39754474579285315 ) ) ;
#28721=EDGE_LOOP ( 'NONE', ( #13971, #15852, #656, #8641, #598, #35817, #43148, #16074, #23540 ) ) ;
#28724=CARTESIAN_POINT ( 'NONE',  ( 69.69189222814998175, -41.76310523276723785, -7.393215200338315363 ) ) ;
#28734=CARTESIAN_POINT ( 'NONE',  ( 116.1082702545247827, 0.1403307496149616695, -11.32035403202665336 ) ) ;
#28742=VECTOR ( 'NONE', #10867, 1000.000000000000114 ) ;
#28745=CARTESIAN_POINT ( 'NONE',  ( 110.4384831777918805, -0.01829820670803256055, -14.64321520033831447 ) ) ;
#28749=DIRECTION ( 'NONE',  ( 0.000000000000000000, 0.000000000000000000, -1.000000000000000000 ) ) ;
#28758=ORIENTED_EDGE ( 'NONE', *, *, #13075, .F. ) ;
#28761=CARTESIAN_POINT ( 'NONE',  ( 115.4831921295247952, 0.8980012041604618078, -13.39321520033831447 ) ) ;
#28762=CARTESIAN_POINT ( 'NONE',  ( 113.6079577545248043, -2.791137627527939813, -18.39754474579286025 ) ) ;
#28763=CARTESIAN_POINT ( 'NONE',  ( 115.7610046295247912, -4.863998795839590272, -18.39754474579285315 ) ) ;
#28768=CARTESIAN_POINT ( 'NONE',  ( 105.5513952545248060, 0.8980012041604421569, -11.00651665394454071 ) ) ;
#28774=CARTESIAN_POINT ( 'NONE',  ( 115.8999108795247821, -8.938348069036489818, -9.318865927141430916 ) ) ;
#28775=CARTESIAN_POINT ( 'NONE',  ( 110.7603796295247918, -4.863998795839590272, -8.388885654883775800 ) ) ;
#28788=VECTOR ( 'NONE', #10788, 1000.000000000000000 ) ;
#28792=VERTEX_POINT ( 'NONE', #17669 ) ;
#28793=CARTESIAN_POINT ( 'NONE',  ( 110.9878884760652795, 0.6362173239733635022, -12.14321520033831625 ) ) ;
#28795=CARTESIAN_POINT ( 'NONE',  ( 116.3166296295247832, -4.863998795839590272, -19.15521520033831493 ) ) ;
#28807=CARTESIAN_POINT ( 'NONE',  ( 111.5938171295247940, -10.62599879583958540, -13.39321520033831447 ) ) ;
#28808=CARTESIAN_POINT ( 'NONE',  ( 117.2294421295247844, -10.76310523276723785, -21.89255013987451548 ) ) ;
#28811=FACE_OUTER_BOUND ( 'NONE', #42402, .T. ) ;
#28812=EDGE_LOOP ( 'NONE', ( #9823, #42592, #4116, #1525, #18552 ) ) ;
#28816=CARTESIAN_POINT ( 'NONE',  ( 117.0806140045248185, 0.1403307496149616695, -15.46607636864997204 ) ) ;
#28817=CARTESIAN_POINT ( 'NONE',  ( 116.1777233795247781, -8.938348069036489818, -17.46756447353520159 ) ) ;
#28822=CARTESIAN_POINT ( 'NONE',  ( 112.3578015045248861, -2.477300249445798297, -7.631215200338321125 ) ) ;
#28829=CARTESIAN_POINT ( 'NONE',  ( 115.8304577545247582, -7.250697342233347165, -7.631215200338321125 ) ) ;
#28830=CARTESIAN_POINT ( 'NONE',  ( 109.2294432855482000, -5.177919973337370863, -18.58740422179702989 ) ) ;
#28834=CARTESIAN_POINT ( 'NONE',  ( 114.8581140045248361, 0.1403307496149616695, -15.46607636864997204 ) ) ;
#28835=CARTESIAN_POINT ( 'NONE',  ( 114.8581140045248361, 0.1403307496149616695, -15.46607636864997204 ) ) ;
#28841=ORIENTED_EDGE ( 'NONE', *, *, #13370, .F. ) ;
#28846=EDGE_LOOP ( 'NONE', ( #10575, #8911, #4075, #1825 ) ) ;
#28851=CARTESIAN_POINT ( 'NONE',  ( 109.7185827545247889, -2.477300249445798297, -19.15521520033831138 ) ) ;
#28854=CARTESIAN_POINT ( 'NONE',  ( 114.5108483795247878, -8.402594152722688392, -16.93181055722141792 ) ) ;
#28861=CARTESIAN_POINT ( 'NONE',  ( 112.7745202545247878, 0.1403307496149616695, -11.32035403202665336 ) ) ;
#28865=CARTESIAN_POINT ( 'NONE',  ( 78.69189222814998175, -71.37806158163368764, -41.02281774838951378 ) ) ;
#28870=EDGE_LOOP ( 'NONE', ( #44813, #10243, #35417, #36080 ) ) ;
#28873=CARTESIAN_POINT ( 'NONE',  ( 113.0523327545247838, -6.936859964151250502, -8.388885654883777576 ) ) ;
#28877=CARTESIAN_POINT ( 'NONE',  ( 84.98581999809579202, -29.69064069796288052, -10.86172087519381435 ) ) ;
#28878=CARTESIAN_POINT ( 'NONE',  ( 107.8433483795247838, -0.7896495226426338832, -9.318865927141430916 ) ) ;
#28882=CARTESIAN_POINT ( 'NONE',  ( 109.2294668361295749, -3.968295118983554026, -7.926221972760173706 ) ) ;
#28884=CARTESIAN_POINT ( 'NONE',  ( 116.5944421295247793, 0.8980012041604618078, -13.39321520033831447 ) ) ;
#28886=FACE_OUTER_BOUND ( 'NONE', #959, .T. ) ;
#28887=FACE_OUTER_BOUND ( 'NONE', #18695, .T. ) ;
#28890=CARTESIAN_POINT ( 'NONE',  ( 110.7603796295247918, -4.863998795839590272, -19.15521520033831493 ) ) ;
#28892=ORIENTED_EDGE ( 'NONE', *, *, #37975, .T. ) ;
#28900=VECTOR ( 'NONE', #20083, 1000.000000000000000 ) ;
#28901=CARTESIAN_POINT ( 'NONE',  ( 114.5803015045248117, -2.477300249445798297, -7.631215200338321125 ) ) ;
#28906=AXIS2_PLACEMENT_3D ( 'NONE', #39674, #5231, #19145 ) ;
#28912=CARTESIAN_POINT ( 'NONE',  ( 115.5212212410415873, 0.7607806665037644134, -12.14321520033829493 ) ) ;
#28915=CARTESIAN_POINT ( 'NONE',  ( 64.12920981708656143, -35.11750645889024014, -5.893215200338315363 ) ) ;
#28918=ADVANCED_FACE ( 'NONE', ( #3970 ), #45085, .T. ) ;
#28931=CARTESIAN_POINT ( 'NONE',  ( 113.3301452545248083, -9.868328341294098749, -15.46607636864997204 ) ) ;
#28932=CARTESIAN_POINT ( 'NONE',  ( 82.42994493343583429, -31.76310523276723430, -22.89321520033831803 ) ) ;
#28933=CYLINDRICAL_SURFACE ( 'NONE', #31903, 2.000000000000001776 ) ;
#28935=CARTESIAN_POINT ( 'NONE',  ( 116.9417077545247992, -2.791137627527939813, -18.39754474579286025 ) ) ;
#28939=CARTESIAN_POINT ( 'NONE',  ( 109.2324108795247923, -1.325403438956436419, -16.93181055722137174 ) ) ;
#28940=AXIS2_PLACEMENT_3D ( 'NONE', #2204, #8835, #36191 ) ;
#28942=CARTESIAN_POINT ( 'NONE',  ( 108.6073327545248048, -6.936859964151250502, -8.388885654883777576 ) ) ;
#28951=CARTESIAN_POINT ( 'NONE',  ( 110.4361338361194811, 0.1075849324168598464, -12.14321520033833046 ) ) ;
#28952=EDGE_CURVE ( 'NONE', #36034, #5046, #24817, .T. ) ;
#28964=CARTESIAN_POINT ( 'NONE',  ( 110.5266510812576826, -0.01829820670803256055, -12.14321520033831625 ) ) ;
#28966=EDGE_LOOP ( 'NONE', ( #12401, #11243, #39081, #30132, #21686 ) ) ;
#28970=CARTESIAN_POINT ( 'NONE',  ( 79.41838382432698040, 5.053604680061214438, -20.45601830029449530 ) ) ;
#28972=ADVANCED_FACE ( 'NONE', ( #13369 ), #13140, .F. ) ;
#28975=DIRECTION ( 'NONE',  ( 1.156482317317869950E-15, 1.000000000000000000, 0.000000000000000000 ) ) ;
#28979=CARTESIAN_POINT ( 'NONE',  ( 116.6714741698188504, -8.633658976779720717, -16.79467234361142047 ) ) ;
#28982=ORIENTED_EDGE ( 'NONE', *, *, #13331, .F. ) ;
#28984=CARTESIAN_POINT ( 'NONE',  ( 115.3442858795247759, -0.7896495226426338832, -17.46756447353520159 ) ) ;
#28985=CARTESIAN_POINT ( 'NONE',  ( 113.8163171295247764, 0.1403307496149613920, -13.39321520033831447 ) ) ;
#28986=CARTESIAN_POINT ( 'NONE',  ( 114.7192077545248594, -2.791137627527939813, -18.39754474579286025 ) ) ;
#28994=CARTESIAN_POINT ( 'NONE',  ( 109.2295025952882526, -0.04762797407389267323, -15.11742090230669611 ) ) ;
#28997=CARTESIAN_POINT ( 'NONE',  ( 110.8992858795247827, -0.7896495226426338832, -17.46756447353520159 ) ) ;
#28998=CARTESIAN_POINT ( 'NONE',  ( 113.6774108795247997, -1.325403438956436419, -16.93181055722141792 ) ) ;
#28999=VERTEX_POINT ( 'NONE', #24079 ) ;
#29011=ORIENTED_EDGE ( 'NONE', *, *, #32345, .T. ) ;
#29015=CARTESIAN_POINT ( 'NONE',  ( 114.6497546295247929, -4.863998795839590272, -7.631215200338315796 ) ) ;
#29018=EDGE_LOOP ( 'NONE', ( #21869, #18153, #39538, #44138 ) ) ;
#29026=CARTESIAN_POINT ( 'NONE',  ( 110.6909265045248247, -7.250697342233347165, -19.15521520033831138 ) ) ;
#29029=EDGE_CURVE ( 'NONE', #42684, #17900, #4582, .T. ) ;
#29031=CARTESIAN_POINT ( 'NONE',  ( 109.2294421295247844, -49.76310523276723785, -19.39321520033831447 ) ) ;
#29034=CARTESIAN_POINT ( 'NONE',  ( 116.0388171295248014, -10.62599879583958540, -13.39321520033831447 ) ) ;
#29036=CARTESIAN_POINT ( 'NONE',  ( 114.4413952545248350, 0.8980012041604421569, -11.00651665394454071 ) ) ;
#29038=ORIENTED_EDGE ( 'NONE', *, *, #7431, .F. ) ;
#29041=CARTESIAN_POINT ( 'NONE',  ( 105.6208483795248299, -0.7896495226426338832, -9.318865927141430916 ) ) ;
#29049=CARTESIAN_POINT ( 'NONE',  ( 109.2294421416092689, -10.38236770277540622, -13.95981693459670048 ) ) ;
#29052=CARTESIAN_POINT ( 'NONE',  ( 111.8021765045248372, -2.791137627527939813, -8.388885654883777576 ) ) ;
#29053=CARTESIAN_POINT ( 'NONE',  ( 106.5931921295248372, 0.8980012041604618078, -13.39321520033831447 ) ) ;
#29055=CARTESIAN_POINT ( 'NONE',  ( 70.19189222814998175, -62.44811955051406471, -34.95094429002801206 ) ) ;
#29058=ORIENTED_EDGE ( 'NONE', *, *, #8324, .T. ) ;
#29063=ORIENTED_EDGE ( 'NONE', *, *, #212, .F. ) ;
#29069=CARTESIAN_POINT ( 'NONE',  ( 114.2330358795247776, -8.402594152722688392, -9.854619843455216355 ) ) ;
#29077=CARTESIAN_POINT ( 'NONE',  ( 109.7880358795247986, -8.402594152722688392, -9.854619843455216355 ) ) ;
#29084=ORIENTED_EDGE ( 'NONE', *, *, #35301, .T. ) ;
#29087=CARTESIAN_POINT ( 'NONE',  ( 112.9134265045247645, -2.791137627527939813, -8.388885654883777576 ) ) ;
#29092=CARTESIAN_POINT ( 'NONE',  ( 86.15278414645355554, -26.86419576995684722, -8.486169908812993157 ) ) ;
#29093=CARTESIAN_POINT ( 'NONE',  ( 110.0658483795247804, -0.7896495226426338832, -9.318865927141430916 ) ) ;
#29100=CARTESIAN_POINT ( 'NONE',  ( 114.0246765045248196, -7.250697342233347165, -19.15521520033831138 ) ) ;
#29102=CARTESIAN_POINT ( 'NONE',  ( 71.67504600870660170, -26.72445618319088823, -4.893215200338314474 ) ) ;
#29105=CARTESIAN_POINT ( 'NONE',  ( 107.2877233795247776, -8.938348069036489818, -17.46756447353520159 ) ) ;
#29107=CARTESIAN_POINT ( 'NONE',  ( 87.44708369096657918, -21.99489077589588604, -20.89321520033831447 ) ) ;
#29109=DIRECTION ( 'NONE',  ( -0.3445294493088589816, -0.9387755102040820088, 0.000000000000000000 ) ) ;
#29116=CARTESIAN_POINT ( 'NONE',  ( 112.2188952545247531, 0.8980012041604421569, -11.00651665394454071 ) ) ;
#29119=CARTESIAN_POINT ( 'NONE',  ( 116.7606190177645402, -4.646879210594899945, -18.55939208857811451 ) ) ;
#29127=CARTESIAN_POINT ( 'NONE',  ( 63.10250807381770244, -31.76310523276723430, -23.89321520033831803 ) ) ;
#29131=CARTESIAN_POINT ( 'NONE',  ( 64.01282776924010420, -34.86145050234441811, -5.893215200338315363 ) ) ;
#29133=DIRECTION ( 'NONE',  ( -1.000000000000000000, 0.000000000000000000, 0.000000000000000000 ) ) ;
#29146=CARTESIAN_POINT ( 'NONE',  ( 109.0935046295247872, -4.863998795839590272, -18.39754474579285315 ) ) ;
#29147=CARTESIAN_POINT ( 'NONE',  ( 112.4967077545247633, -2.791137627527939813, -18.39754474579286025 ) ) ;
#29148=CARTESIAN_POINT ( 'NONE',  ( 83.47559691244318003, -32.81415873735240041, -23.89321520033831803 ) ) ;
#29149=CARTESIAN_POINT ( 'NONE',  ( 66.69189222814998175, -41.76310523276723785, -24.39321520033831447 ) ) ;
#29151=CARTESIAN_POINT ( 'NONE',  ( 116.2471765045247594, -2.791137627527939813, -8.388885654883777576 ) ) ;
#29153=AXIS2_PLACEMENT_3D ( 'NONE', #38318, #14160, #41333 ) ;
#29157=CARTESIAN_POINT ( 'NONE',  ( 106.6626452545248611, -9.868328341294098749, -15.46607636864997204 ) ) ;
#29164=CARTESIAN_POINT ( 'NONE',  ( 71.50489436060276205, -24.57757939319463958, -4.893215200338314474 ) ) ;
#29168=CARTESIAN_POINT ( 'NONE',  ( 116.7333483795247844, -8.402594152722688392, -16.93181055722141792 ) ) ;
#29171=B_SPLINE_CURVE_WITH_KNOTS ( 'NONE', 3,
 ( #36480, #1819, #1154, #8229, #5021, #25782, #18937, #11651, #1595, #12106 ),
 .UNSPECIFIED., .F., .F.,
 ( 4, 3, 3, 4 ),
 ( 0.000000000000000000, 0.0002476486447138990187, 0.0004952972925464390165, 0.0009604418836934789901 ),
 .UNSPECIFIED. ) ;
#29183=AXIS2_PLACEMENT_3D ( 'NONE', #43681, #22929, #36822 ) ;
#29187=EDGE_CURVE ( 'NONE', #16480, #18690, #2947, .T. ) ;
#29196=EDGE_CURVE ( 'NONE', #36673, #25696, #15177, .T. ) ;
#29200=CARTESIAN_POINT ( 'NONE',  ( 114.7192077545248594, -7.250697342233347165, -7.631215200338321125 ) ) ;
#29201=CARTESIAN_POINT ( 'NONE',  ( 111.8021765045248372, -2.791137627527939813, -8.388885654883777576 ) ) ;
#29202=CARTESIAN_POINT ( 'NONE',  ( 111.1076452545248259, -9.868328341294098749, -15.46607636864997204 ) ) ;
#29208=CARTESIAN_POINT ( 'NONE',  ( 108.1906140045248463, -10.62599879583958717, -11.00651665394454604 ) ) ;
#29214=CARTESIAN_POINT ( 'NONE',  ( 111.4549108795247747, -8.938348069036489818, -9.318865927141430916 ) ) ;
#29215=CARTESIAN_POINT ( 'NONE',  ( 112.6356140045247827, 0.1403307496149616695, -15.46607636864997204 ) ) ;
#29222=AXIS2_PLACEMENT_3D ( 'NONE', #21439, #32585, #35322 ) ;
#29236=CARTESIAN_POINT ( 'NONE',  ( 106.0375671295248310, 0.1403307496149613920, -13.39321520033831447 ) ) ;
#29248=CARTESIAN_POINT ( 'NONE',  ( 111.7327233795247849, -8.938348069036489818, -17.46756447353520159 ) ) ;
#29258=CARTESIAN_POINT ( 'NONE',  ( 112.7050671295247923, -10.62599879583958540, -13.39321520033831447 ) ) ;
#29259=CARTESIAN_POINT ( 'NONE',  ( 116.1777233795247781, -1.325403438956436419, -9.854619843455211026 ) ) ;
#29260=CARTESIAN_POINT ( 'NONE',  ( 113.5385046295247804, -4.863998795839590272, -7.631215200338315796 ) ) ;
#29262=ORIENTED_EDGE ( 'NONE', *, *, #11406, .F. ) ;
#29265=CARTESIAN_POINT ( 'NONE',  ( 105.8986608795248401, -8.938348069036489818, -9.318865927141430916 ) ) ;
#29269=CARTESIAN_POINT ( 'NONE',  ( 117.0080256338066960, -11.48975918537441210, -5.808803638225159993 ) ) ;
#29270=ORIENTED_EDGE ( 'NONE', *, *, #31744, .T. ) ;
#29272=CARTESIAN_POINT ( 'NONE',  ( 109.2292177412187755, -9.286740210711322163, -9.723229054767012158 ) ) ;
#29274=CARTESIAN_POINT ( 'NONE',  ( 111.4549108795247747, -1.325403438956436419, -16.93181055722141792 ) ) ;
#29275=CARTESIAN_POINT ( 'NONE',  ( 107.2182702545248105, -10.62599879583958717, -15.77991374673208469 ) ) ;
#29277=CARTESIAN_POINT ( 'NONE',  ( 70.19189222814998175, -65.04786711941002864, -39.22192925581980916 ) ) ;
#29283=CIRCLE ( 'NONE', #11806, 4.999999999999999112 ) ;
#29293=CARTESIAN_POINT ( 'NONE',  ( 69.87572422742091760, -11.86958442233774313, -21.89321520033831447 ) ) ;
#29294=AXIS2_PLACEMENT_3D ( 'NONE', #12127, #32848, #26486 ) ;
#29296=CARTESIAN_POINT ( 'NONE',  ( 114.3024890045248156, -9.868328341294098749, -11.32035403202665869 ) ) ;
#29303=LINE ( 'NONE', #12894, #30210 ) ;
#29304=CARTESIAN_POINT ( 'NONE',  ( 111.0381921295247878, -9.868328341294093420, -13.39321520033831447 ) ) ;
#29307=AXIS2_PLACEMENT_3D ( 'NONE', #35035, #17308, #34163 ) ;
#29314=CARTESIAN_POINT ( 'NONE',  ( 66.82415148905926117, -40.21211973637273474, -19.39321520033831447 ) ) ;
#29315=CARTESIAN_POINT ( 'NONE',  ( 110.8298327545248299, -6.936859964151250502, -8.388885654883777576 ) ) ;
#29321=CARTESIAN_POINT ( 'NONE',  ( 110.5520202545248054, -10.62599879583958717, -15.77991374673208469 ) ) ;
#29327=CARTESIAN_POINT ( 'NONE',  ( 115.8304577545247582, -7.250697342233347165, -7.631215200338321125 ) ) ;
#29328=DIRECTION ( 'NONE',  ( 0.000000000000000000, 0.9284778069183720062, 0.3713878862591650232 ) ) ;
#29329=CARTESIAN_POINT ( 'NONE',  ( 117.2294421295247844, 0.2335149919452661482, -21.89321520033831447 ) ) ;
#29332=CARTESIAN_POINT ( 'NONE',  ( 106.3848327545248651, -2.477300249445798297, -19.15521520033831138 ) ) ;
#29336=CARTESIAN_POINT ( 'NONE',  ( 112.1997457829843938, 0.6362173239733635022, -14.64321520033831447 ) ) ;
#29340=EDGE_CURVE ( 'NONE', #24500, #30574, #25192, .T. ) ;
#29345=CARTESIAN_POINT ( 'NONE',  ( 108.1906140045248463, -10.62599879583958717, -11.00651665394454604 ) ) ;
#29347=CARTESIAN_POINT ( 'NONE',  ( 110.4131140045248145, -10.62599879583958540, -11.00651665394454071 ) ) ;
#29354=DIRECTION ( 'NONE',  ( 1.000000000000000000, 0.000000000000000000, 0.000000000000000000 ) ) ;
#29369=CARTESIAN_POINT ( 'NONE',  ( 113.1912390045248031, -9.868328341294098749, -11.32035403202665869 ) ) ;
#29373=CARTESIAN_POINT ( 'NONE',  ( 114.5803015045248117, -2.477300249445798297, -7.631215200338321125 ) ) ;
#29374=CARTESIAN_POINT ( 'NONE',  ( 108.9545983795247821, -8.402594152722688392, -16.93181055722141792 ) ) ;
#29376=AXIS2_PLACEMENT_3D ( 'NONE', #34381, #10460, #7029 ) ;
#29379=CARTESIAN_POINT ( 'NONE',  ( 117.0806140045248185, 0.1403307496149616695, -15.46607636864997204 ) ) ;
#29385=CARTESIAN_POINT ( 'NONE',  ( 107.2877233795247776, -1.325403438956436419, -9.854619843455211026 ) ) ;
#29394=CARTESIAN_POINT ( 'NONE',  ( 71.79922130029189020, -25.12209812792223929, -4.893215200338314474 ) ) ;
#29396=AXIS2_PLACEMENT_3D ( 'NONE', #23864, #23176, #40273 ) ;
#29397=CARTESIAN_POINT ( 'NONE',  ( 116.8722546295247895, -4.863998795839590272, -18.39754474579285315 ) ) ;
#29403=CARTESIAN_POINT ( 'NONE',  ( 110.7603796295247918, -4.863998795839638234, -8.388885654883775800 ) ) ;
#29413=CARTESIAN_POINT ( 'NONE',  ( 114.3339130180080758, 0.7607806665038616689, -14.64321520033833579 ) ) ;
#29417=CARTESIAN_POINT ( 'NONE',  ( 116.6331291116711526, -9.576227594267002985, -15.17824202297639857 ) ) ;
#29424=CARTESIAN_POINT ( 'NONE',  ( 114.2330358795247776, -0.7896495226426338832, -17.46756447353520159 ) ) ;
#29425=CARTESIAN_POINT ( 'NONE',  ( 108.6767858795247861, -8.402594152722688392, -9.854619843455216355 ) ) ;
#29426=CARTESIAN_POINT ( 'NONE',  ( 108.2600671295247992, 0.1403307496149613920, -13.39321520033831447 ) ) ;
#29430=CARTESIAN_POINT ( 'NONE',  ( 106.3848327545248651, -2.477300249445798297, -19.15521520033831138 ) ) ;
#29435=CARTESIAN_POINT ( 'NONE',  ( 112.2188952545247531, 0.8980012041604421569, -11.00651665394454071 ) ) ;
#29441=( BOUNDED_SURFACE ( )  B_SPLINE_SURFACE ( 1, 2, ( 
 ( #9301, #9522, #12503, #33220, #36200, #40310, #40540, #26626, #40081, #23209, #12723, #37088, #40765, #44194, #5862, #19784, #5418, #26400, #4965, #22522, #19334, #1995, #9074, #8624, #36419, #32991, #8844, #30044, #33666, #2444, #18877, #22976, #16366, #5187, #30268, #15920, #26175, #12956, #29818, #25952, #36866, #19557, #32768, #26852, #43734, #5636, #33434, #1542, #15463, #1765, #12279, #43280, #2213, #16143, #43960, #22743, #36645, #29369, #12050, #39859, #15691, #29594, #24690, #44390, #24917, #74, #7582, #35154, #2875, #38813, #3710, #19988, #17853, #13987, #16576, #27902, #6068, #34107, #4160, #33875, #520, #21496, #35381, #20221, #28340, #21047, #41817, #18075, #31971, #297, #27057, #2644, #16806, #21272, #14655, #28124, #31302, #30470, #40977, #7136, #733, #28570, #10573, #38579, #3934, #11016, #9500, #17630, #23414, #31752, #34924, #7356, #23643, #37302, #42034, #24472, #13155, #9733, #31527, #37530, #6302, #38362, #14432, #42253, #14210, #10793, #4830, #19201, #18970, #22167, #11914, #11471, #25375, #42925, #21942, #29456, #8262, #32859, #25594, #5055, #26041, #12138, #35610, #18752, #36061, #42479, #39722, #4385, #15779, #11688, #18299, #32641, #1409, #15327, #43369, #35833, #32194, #1629, #8487, #39273, #29236 ),
 ( #39500, #43143, #25813, #14884, #28795, #8036, #15106, #36287, #39946, #8708, #11241, #22392, #22613, #4607, #36511, #15549, #32420, #5285, #33079, #967, #1851, #25149, #39044, #7816, #21723, #42701, #18528, #1193, #29015, #26497, #36953, #36733, #9385, #19878, #13040, #33529, #30140, #2767, #26266, #16237, #40173, #44055, #19642, #6426, #8938, #20110, #22841, #19419, #2535, #30365, #44287, #37180, #12821, #5498, #5724, #33306, #26719, #16005, #40628, #2081, #29682, #23761, #27173, #2307, #41094, #29913, #43593, #23295, #2992, #43827, #9853, #9616, #26939, #12594, #40405, #9165, #33766, #6191, #23069, #13267, #44504, #5953, #16461, #40863, #23536, #37421, #33996, #16691, #37651, #30583, #20336, #34219, #12366, #242, #14376, #24864, #10081, #34437, #24418, #23984, #20556, #28289, #44960, #27624, #7085, #14151, #13717, #13934, #17577, #38308, #27846, #461, #3216, #7525, #35095, #28067, #35327, #3442, #30812, #44736, #17143, #13495, #10301, #27400, #42198, #31469, #6648, #31693, #6869, #10959, #41976, #24202, #38755, #10516, #41322, #24640, #20778, #37872, #34657, #31029, #41538, #21441, #38093, #7300, #16918, #17361, #31249, #3877, #41756, #21, #20994, #34868, #3656, #10741, #38522, #21219, #17799, #8655, #22116, #11413, #14599 ) ),
 .UNSPECIFIED., .F., .F., .T. ) 
 B_SPLINE_SURFACE_WITH_KNOTS ( ( 2, 2 ),
 ( 3, 2, 2, 2, 2, 2, 2, 2, 2, 2, 2, 2, 2, 2, 2, 2, 2, 2, 2, 2, 2, 2, 2, 2, 2, 2, 2, 2, 2, 2, 2, 2, 2, 2, 2, 2, 2, 2, 2, 2, 2, 2, 2, 2, 2, 2, 2, 2, 2, 2, 2, 2, 2, 2, 2, 2, 2, 2, 2, 2, 2, 2, 2, 2, 2, 2, 2, 2, 2, 2, 2, 2, 2, 2, 2, 2, 2, 2, 2, 2, 3 ),
 ( 0.000000000000000000, 1.000000000000000000 ),
 ( 0.000000000000000000, 0.01250000000000000069, 0.02500000000000000139, 0.03749999999999999861, 0.05000000000000000278, 0.06250000000000000000, 0.07499999999999999722, 0.08749999999999999445, 0.1000000000000000056, 0.1125000000000000028, 0.1250000000000000000, 0.1375000000000000111, 0.1499999999999999944, 0.1625000000000000056, 0.1749999999999999889, 0.1875000000000000000, 0.2000000000000000111, 0.2124999999999999944, 0.2250000000000000056, 0.2374999999999999889, 0.2500000000000000000, 0.2625000000000000111, 0.2750000000000000222, 0.2874999999999999778, 0.2999999999999999889, 0.3125000000000000000, 0.3250000000000000111, 0.3375000000000000222, 0.3499999999999999778, 0.3624999999999999889, 0.3750000000000000000, 0.3875000000000000111, 0.4000000000000000222, 0.4124999999999999778, 0.4249999999999999889, 0.4375000000000000000, 0.4500000000000000111, 0.4625000000000000222, 0.4749999999999999778, 0.4874999999999999889, 0.5000000000000000000, 0.5124999999999999556, 0.5250000000000000222, 0.5374999999999999778, 0.5500000000000000444, 0.5625000000000000000, 0.5749999999999999556, 0.5875000000000000222, 0.5999999999999999778, 0.6125000000000000444, 0.6250000000000000000, 0.6374999999999999556, 0.6500000000000000222, 0.6624999999999999778, 0.6750000000000000444, 0.6875000000000000000, 0.6999999999999999556, 0.7125000000000000222, 0.7249999999999999778, 0.7375000000000000444, 0.7500000000000000000, 0.7624999999999999556, 0.7750000000000000222, 0.7874999999999999778, 0.8000000000000000444, 0.8125000000000000000, 0.8249999999999999556, 0.8375000000000000222, 0.8499999999999999778, 0.8625000000000000444, 0.8750000000000000000, 0.8874999999999999556, 0.9000000000000000222, 0.9124999999999999778, 0.9250000000000000444, 0.9375000000000000000, 0.9499999999999999556, 0.9625000000000000222, 0.9749999999999999778, 0.9875000000000000444, 1.000000000000000000 ),
 .UNSPECIFIED. ) 
 GEOMETRIC_REPRESENTATION_ITEM ( )  RATIONAL_B_SPLINE_SURFACE ( (
 ( 1.000000000000000000, 0.9238795325112869605, 1.000000000000000000, 0.9238795325112869605, 1.000000000000000000, 0.9238795325112869605, 1.000000000000000000, 0.9238795325112869605, 1.000000000000000000, 0.9238795325112869605, 1.000000000000000000, 0.9238795325112869605, 1.000000000000000000, 0.9238795325112869605, 1.000000000000000000, 0.9238795325112869605, 1.000000000000000000, 0.9238795325112869605, 1.000000000000000000, 0.9238795325112869605, 1.000000000000000000, 0.9238795325112869605, 1.000000000000000000, 0.9238795325112869605, 1.000000000000000000, 0.9238795325112869605, 1.000000000000000000, 0.9238795325112869605, 1.000000000000000000, 0.9238795325112869605, 1.000000000000000000, 0.9238795325112869605, 1.000000000000000000, 0.9238795325112869605, 1.000000000000000000, 0.9238795325112869605, 1.000000000000000000, 0.9238795325112869605, 1.000000000000000000, 0.9238795325112869605, 1.000000000000000000, 0.9238795325112869605, 1.000000000000000000, 0.9238795325112869605, 1.000000000000000000, 0.9238795325112869605, 1.000000000000000000, 0.9238795325112869605, 1.000000000000000000, 0.9238795325112869605, 1.000000000000000000, 0.9238795325112869605, 1.000000000000000000, 0.9238795325112869605, 1.000000000000000000, 0.9238795325112869605, 1.000000000000000000, 0.9238795325112869605, 1.000000000000000000, 0.9238795325112869605, 1.000000000000000000, 0.9238795325112869605, 1.000000000000000000, 0.9238795325112869605, 1.000000000000000000, 0.9238795325112869605, 1.000000000000000000, 0.9238795325112869605, 1.000000000000000000, 0.9238795325112869605, 1.000000000000000000, 0.9238795325112869605, 1.000000000000000000, 0.9238795325112869605, 1.000000000000000000, 0.9238795325112869605, 1.000000000000000000, 0.9238795325112869605, 1.000000000000000000, 0.9238795325112869605, 1.000000000000000000, 0.9238795325112869605, 1.000000000000000000, 0.9238795325112869605, 1.000000000000000000, 0.9238795325112869605, 1.000000000000000000, 0.9238795325112869605, 1.000000000000000000, 0.9238795325112869605, 1.000000000000000000, 0.9238795325112869605, 1.000000000000000000, 0.9238795325112869605, 1.000000000000000000, 0.9238795325112869605, 1.000000000000000000, 0.9238795325112869605, 1.000000000000000000, 0.9238795325112869605, 1.000000000000000000, 0.9238795325112869605, 1.000000000000000000, 0.9238795325112869605, 1.000000000000000000, 0.9238795325112869605, 1.000000000000000000, 0.9238795325112869605, 1.000000000000000000, 0.9238795325112869605, 1.000000000000000000, 0.9238795325112869605, 1.000000000000000000, 0.9238795325112869605, 1.000000000000000000, 0.9238795325112869605, 1.000000000000000000, 0.9238795325112869605, 1.000000000000000000, 0.9238795325112869605, 1.000000000000000000, 0.9238795325112869605, 1.000000000000000000, 0.9238795325112869605, 1.000000000000000000, 0.9238795325112869605, 1.000000000000000000, 0.9238795325112869605, 1.000000000000000000, 0.9238795325112869605, 1.000000000000000000, 0.9238795325112869605, 1.000000000000000000, 0.9238795325112869605, 1.000000000000000000, 0.9238795325112869605, 1.000000000000000000, 0.9238795325112869605, 1.000000000000000000, 0.9238795325112869605, 1.000000000000000000, 0.9238795325112869605, 1.000000000000000000, 0.9238795325112869605, 1.000000000000000000, 0.9238795325112869605, 1.000000000000000000, 0.9238795325112869605, 1.000000000000000000, 0.9238795325112869605, 1.000000000000000000, 0.9238795325112869605, 1.000000000000000000, 0.9238795325112869605, 1.000000000000000000, 0.9238795325112869605, 1.000000000000000000, 0.9238795325112869605, 1.000000000000000000, 0.9238795325112869605, 1.000000000000000000),
 ( 1.000000000000000000, 0.9238795325112869605, 1.000000000000000000, 0.9238795325112869605, 1.000000000000000000, 0.9238795325112869605, 1.000000000000000000, 0.9238795325112869605, 1.000000000000000000, 0.9238795325112869605, 1.000000000000000000, 0.9238795325112869605, 1.000000000000000000, 0.9238795325112869605, 1.000000000000000000, 0.9238795325112869605, 1.000000000000000000, 0.9238795325112869605, 1.000000000000000000, 0.9238795325112869605, 1.000000000000000000, 0.9238795325112869605, 1.000000000000000000, 0.9238795325112869605, 1.000000000000000000, 0.9238795325112869605, 1.000000000000000000, 0.9238795325112869605, 1.000000000000000000, 0.9238795325112869605, 1.000000000000000000, 0.9238795325112869605, 1.000000000000000000, 0.9238795325112869605, 1.000000000000000000, 0.9238795325112869605, 1.000000000000000000, 0.9238795325112869605, 1.000000000000000000, 0.9238795325112869605, 1.000000000000000000, 0.9238795325112869605, 1.000000000000000000, 0.9238795325112869605, 1.000000000000000000, 0.9238795325112869605, 1.000000000000000000, 0.9238795325112869605, 1.000000000000000000, 0.9238795325112869605, 1.000000000000000000, 0.9238795325112869605, 1.000000000000000000, 0.9238795325112869605, 1.000000000000000000, 0.9238795325112869605, 1.000000000000000000, 0.9238795325112869605, 1.000000000000000000, 0.9238795325112869605, 1.000000000000000000, 0.9238795325112869605, 1.000000000000000000, 0.9238795325112869605, 1.000000000000000000, 0.9238795325112869605, 1.000000000000000000, 0.9238795325112869605, 1.000000000000000000, 0.9238795325112869605, 1.000000000000000000, 0.9238795325112869605, 1.000000000000000000, 0.9238795325112869605, 1.000000000000000000, 0.9238795325112869605, 1.000000000000000000, 0.9238795325112869605, 1.000000000000000000, 0.9238795325112869605, 1.000000000000000000, 0.9238795325112869605, 1.000000000000000000, 0.9238795325112869605, 1.000000000000000000, 0.9238795325112869605, 1.000000000000000000, 0.9238795325112869605, 1.000000000000000000, 0.9238795325112869605, 1.000000000000000000, 0.9238795325112869605, 1.000000000000000000, 0.9238795325112869605, 1.000000000000000000, 0.9238795325112869605, 1.000000000000000000, 0.9238795325112869605, 1.000000000000000000, 0.9238795325112869605, 1.000000000000000000, 0.9238795325112869605, 1.000000000000000000, 0.9238795325112869605, 1.000000000000000000, 0.9238795325112869605, 1.000000000000000000, 0.9238795325112869605, 1.000000000000000000, 0.9238795325112869605, 1.000000000000000000, 0.9238795325112869605, 1.000000000000000000, 0.9238795325112869605, 1.000000000000000000, 0.9238795325112869605, 1.000000000000000000, 0.9238795325112869605, 1.000000000000000000, 0.9238795325112869605, 1.000000000000000000, 0.9238795325112869605, 1.000000000000000000, 0.9238795325112869605, 1.000000000000000000, 0.9238795325112869605, 1.000000000000000000, 0.9238795325112869605, 1.000000000000000000, 0.9238795325112869605, 1.000000000000000000, 0.9238795325112869605, 1.000000000000000000, 0.9238795325112869605, 1.000000000000000000, 0.9238795325112869605, 1.000000000000000000, 0.9238795325112869605, 1.000000000000000000, 0.9238795325112869605, 1.000000000000000000, 0.9238795325112869605, 1.000000000000000000, 0.9238795325112869605, 1.000000000000000000, 0.9238795325112869605, 1.000000000000000000, 0.9238795325112869605, 1.000000000000000000, 0.9238795325112869605, 1.000000000000000000, 0.9238795325112869605, 1.000000000000000000, 0.9238795325112869605, 1.000000000000000000, 0.9238795325112869605, 1.000000000000000000, 0.9238795325112869605, 1.000000000000000000, 0.9238795325112869605, 1.000000000000000000) ) ) 
 REPRESENTATION_ITEM ( '' )  SURFACE ( )  );
#29449=CARTESIAN_POINT ( 'NONE',  ( 63.69189222814998175, -50.16718729050181480, 3.106784799661685526 ) ) ;
#29452=CARTESIAN_POINT ( 'NONE',  ( 110.6214888068194853, 0.1168444861213632779, -12.14321520033831625 ) ) ;
#29456=CARTESIAN_POINT ( 'NONE',  ( 107.7738952545248310, -9.868328341294098749, -15.46607636864997204 ) ) ;
#29463=EDGE_LOOP ( 'NONE', ( #29058, #16892, #26914, #36778 ) ) ;
#29464=CARTESIAN_POINT ( 'NONE',  ( 61.69189222814998175, -49.76310523276723785, -34.89321520033831092 ) ) ;
#29465=CARTESIAN_POINT ( 'NONE',  ( 62.15747001998436616, -65.30058926756809967, -44.86669339845351345 ) ) ;
#29466=CARTESIAN_POINT ( 'NONE',  ( 107.1488171295247867, -10.62599879583958540, -13.39321520033831447 ) ) ;
#29468=ADVANCED_FACE ( 'NONE', ( #7176 ), #35713, .F. ) ;
#29472=CARTESIAN_POINT ( 'NONE',  ( 65.19189222814998175, -41.76310523276723785, -24.39321520033831447 ) ) ;
#29479=CARTESIAN_POINT ( 'NONE',  ( 110.9687390045248350, 0.8980012041604421569, -15.77991374673208469 ) ) ;
#29480=CARTESIAN_POINT ( 'NONE',  ( 116.3860827545247787, -6.936859964151250502, -8.388885654883777576 ) ) ;
#29481=CARTESIAN_POINT ( 'NONE',  ( 110.3436608795247764, -8.938348069036489818, -9.318865927141430916 ) ) ;
#29485=CARTESIAN_POINT ( 'NONE',  ( 62.22678445075433018, -36.72958069525633817, -5.531797115907686191 ) ) ;
#29491=CARTESIAN_POINT ( 'NONE',  ( 116.6168215951329472, -11.86651415378938879, -6.422085954748080638 ) ) ;
#29492=ORIENTED_EDGE ( 'NONE', *, *, #7632, .T. ) ;
#29493=FACE_OUTER_BOUND ( 'NONE', #268, .T. ) ;
#29494=CARTESIAN_POINT ( 'NONE',  ( 109.2294501619033156, -10.07790831936271658, -11.17625042590223927 ) ) ;
#29496=CARTESIAN_POINT ( 'NONE',  ( 110.6909265045248247, -2.791137627527939813, -8.388885654883777576 ) ) ;
#29497=CARTESIAN_POINT ( 'NONE',  ( 106.8015515045248378, -2.477300249445798297, -7.631215200338321125 ) ) ;
#29500=CARTESIAN_POINT ( 'NONE',  ( 69.92918015000313403, -25.34836422082628715, -5.722398249991065278 ) ) ;
#29504=EDGE_CURVE ( 'NONE', #44074, #9856, #24090, .T. ) ;
#29517=CARTESIAN_POINT ( 'NONE',  ( 107.5655358795247736, -0.7896495226426338832, -17.46756447353520159 ) ) ;
#29521=CARTESIAN_POINT ( 'NONE',  ( 113.8857702545248003, 0.1403307496149616695, -11.32035403202665336 ) ) ;
#29522=CARTESIAN_POINT ( 'NONE',  ( 79.72353890764954087, 4.236894767232761261, -14.64321520033831447 ) ) ;
#29523=DIRECTION ( 'NONE',  ( 0.000000000000000000, 0.000000000000000000, -1.000000000000000000 ) ) ;
#29529=CARTESIAN_POINT ( 'NONE',  ( 116.9448827545247696, -2.792930983974093007, -18.39321520033830737 ) ) ;
#29530=CARTESIAN_POINT ( 'NONE',  ( 112.8439733795247832, -1.325403438956436419, -9.854619843455211026 ) ) ;
#29541=CARTESIAN_POINT ( 'NONE',  ( 108.3295202545248657, 0.1403307496149616695, -11.32035403202665336 ) ) ;
#29546=CARTESIAN_POINT ( 'NONE',  ( 107.6349890045248401, 0.8980012041604421569, -15.77991374673208469 ) ) ;
#29549=DIRECTION ( 'NONE',  ( -1.000000000000000000, 1.214306433183763980E-15, 0.000000000000000000 ) ) ;
#29551=CARTESIAN_POINT ( 'NONE',  ( 112.9828796295247884, -4.863998795839590272, -19.15521520033831493 ) ) ;
#29552=CARTESIAN_POINT ( 'NONE',  ( 82.89134431723762475, -31.13449359622123680, -21.94632144483577818 ) ) ;
#29555=CARTESIAN_POINT ( 'NONE',  ( 107.5655358795247736, -0.7896495226426338832, -17.46756447353520159 ) ) ;
#29558=ORIENTED_EDGE ( 'NONE', *, *, #18171, .T. ) ;
#29559=CARTESIAN_POINT ( 'NONE',  ( 112.2879504682428831, 0.5115630086001619059, -14.64321520033830026 ) ) ;
#29567=CARTESIAN_POINT ( 'NONE',  ( 110.8992858795247827, -0.7896495226426338832, -17.46756447353520159 ) ) ;
#29569=CARTESIAN_POINT ( 'NONE',  ( 116.7862463306490355, -3.361876234510294381, -18.36316846464617214 ) ) ;
#29577=CARTESIAN_POINT ( 'NONE',  ( 70.19189222814998175, -75.31442247550839397, -37.94335727672635983 ) ) ;
#29582=CARTESIAN_POINT ( 'NONE',  ( 64.01282776924008999, -34.86145050234441811, -5.893215200338315363 ) ) ;
#29584=CARTESIAN_POINT ( 'NONE',  ( 109.6473066399283880, 0.4261359969231631739, -14.64321520033828605 ) ) ;
#29594=CARTESIAN_POINT ( 'NONE',  ( 112.9134265045247645, -2.791137627527939813, -8.388885654883777576 ) ) ;
#29597=CARTESIAN_POINT ( 'NONE',  ( 114.3024890045248156, 0.8980012041604421569, -15.77991374673208469 ) ) ;
#29598=CARTESIAN_POINT ( 'NONE',  ( 109.8574890045248509, -9.868328341294098749, -11.32035403202665869 ) ) ;
#29599=DIRECTION ( 'NONE',  ( 0.000000000000000000, -1.000000000000000000, 0.000000000000000000 ) ) ;
#29601=CARTESIAN_POINT ( 'NONE',  ( 63.69189222814998175, -50.16718729050181480, -6.893215200338315363 ) ) ;
#29609=CARTESIAN_POINT ( 'NONE',  ( 108.8156921295247912, -9.868328341294093420, -13.39321520033831447 ) ) ;
#29620=CARTESIAN_POINT ( 'NONE',  ( 110.6214733795247867, -1.325403438956436419, -9.854619843455211026 ) ) ;
#29627=DIRECTION ( 'NONE',  ( 0.000000000000000000, 0.000000000000000000, -1.000000000000000000 ) ) ;
#29631=CIRCLE ( 'NONE', #14370, 5.635000000000000675 ) ;
#29649=CARTESIAN_POINT ( 'NONE',  ( 113.4690515045247992, -2.477300249445798297, -7.631215200338321125 ) ) ;
#29650=CARTESIAN_POINT ( 'NONE',  ( 109.4407702545248355, 0.1403307496149616695, -11.32035403202665336 ) ) ;
#29651=CARTESIAN_POINT ( 'NONE',  ( 107.4266296295248821, -4.863998795839590272, -8.388885654883775800 ) ) ;
#29656=LINE ( 'NONE', #15980, #36885 ) ;
#29662=CARTESIAN_POINT ( 'NONE',  ( 108.6073327545248048, -2.477300249445798297, -19.15521520033831138 ) ) ;
#29663=DIRECTION ( 'NONE',  ( 0.000000000000000000, 0.000000000000000000, -1.000000000000000000 ) ) ;
#29664=ORIENTED_EDGE ( 'NONE', *, *, #6978, .T. ) ;
#29681=CIRCLE ( 'NONE', #15855, 5.000000000000004441 ) ;
#29682=CARTESIAN_POINT ( 'NONE',  ( 112.4272546295247821, -4.863998795839590272, -7.631215200338315796 ) ) ;
#29691=CARTESIAN_POINT ( 'NONE',  ( 71.83824405425508530, -26.34469659010723674, -4.893215200338314474 ) ) ;
#29692=CARTESIAN_POINT ( 'NONE',  ( 106.1764733795248219, -8.938348069036489818, -17.46756447353520159 ) ) ;
#29699=VERTEX_POINT ( 'NONE', #42963 ) ;
#29702=CARTESIAN_POINT ( 'NONE',  ( 113.5385046295247804, -4.863998795839590272, -7.631215200338315796 ) ) ;
#29704=CARTESIAN_POINT ( 'NONE',  ( 109.6491296295247793, -4.863998795839590272, -19.15521520033831493 ) ) ;
#29709=CARTESIAN_POINT ( 'NONE',  ( 108.3295202545248657, -10.62599879583958717, -15.77991374673208469 ) ) ;
#29712=DIRECTION ( 'NONE',  ( 1.000000000000000000, 2.774032902257834535E-17, 0.000000000000000000 ) ) ;
#29713=CARTESIAN_POINT ( 'NONE',  ( 116.9589894550429250, -11.55723876051829180, -5.895360932783320962 ) ) ;
#29714=VERTEX_POINT ( 'NONE', #29055 ) ;
#29716=CARTESIAN_POINT ( 'NONE',  ( 109.2295558771343309, -9.780153738166868393, -15.77098437576014334 ) ) ;
#29718=CARTESIAN_POINT ( 'NONE',  ( 110.8992858795247827, -8.402594152722688392, -9.854619843455216355 ) ) ;
#29719=CARTESIAN_POINT ( 'NONE',  ( 112.2883483795247770, -8.402594152722688392, -16.93181055722141792 ) ) ;
#29722=CARTESIAN_POINT ( 'NONE',  ( 69.24601164033393275, -26.03124926770523473, -5.871647083323535021 ) ) ;
#29733=ADVANCED_FACE ( 'NONE', ( #12409 ), #1673, .T. ) ;
#29738=CARTESIAN_POINT ( 'NONE',  ( 107.4266296295248821, -4.863998795839590272, -19.15521520033831493 ) ) ;
#29741=CARTESIAN_POINT ( 'NONE',  ( 111.4549108795247747, -1.325403438956436419, -16.93181055722141792 ) ) ;
#29750=CARTESIAN_POINT ( 'NONE',  ( 108.2600671295247992, 0.1403307496149613920, -13.39321520033831447 ) ) ;
#29756=CARTESIAN_POINT ( 'NONE',  ( 70.38348191167295909, -26.39350520520921961, -5.594626746640797954 ) ) ;
#29760=CARTESIAN_POINT ( 'NONE',  ( 114.7886454522301989, 0.1168444861213632779, -14.64321520033831447 ) ) ;
#29762=CARTESIAN_POINT ( 'NONE',  ( 109.9963952545248134, -9.868328341294098749, -15.46607636864997204 ) ) ;
#29763=ADVANCED_FACE ( 'NONE', ( #33125 ), #8531, .T. ) ;
#29768=CARTESIAN_POINT ( 'NONE',  ( 106.1764733795248219, -8.938348069036489818, -17.46756447353520159 ) ) ;
#29771=FACE_OUTER_BOUND ( 'NONE', #28846, .T. ) ;
#29772=CARTESIAN_POINT ( 'NONE',  ( 109.7880358795247986, -0.7896495226426338832, -17.46756447353520159 ) ) ;
#29774=CARTESIAN_POINT ( 'NONE',  ( 83.43891948909487155, -32.91635598341913749, -23.82430106395967684 ) ) ;
#29777=CARTESIAN_POINT ( 'NONE',  ( 107.2182702545248105, -10.62599879583958717, -15.77991374673208469 ) ) ;
#29782=ADVANCED_FACE ( 'NONE', ( #36774 ), #5545, .F. ) ;
#29791=EDGE_CURVE ( 'NONE', #11630, #14918, #27142, .T. ) ;
#29793=CARTESIAN_POINT ( 'NONE',  ( 107.0099108795247815, -8.938348069036489818, -9.318865927141430916 ) ) ;
#29796=CARTESIAN_POINT ( 'NONE',  ( 110.0170221536727553, 0.3967854368540359999, -10.50530088663810169 ) ) ;
#29799=VECTOR ( 'NONE', #30889, 1000.000000000000000 ) ;
#29818=CARTESIAN_POINT ( 'NONE',  ( 114.5108483795247878, -8.402594152722688392, -16.93181055722141792 ) ) ;
#29822=CARTESIAN_POINT ( 'NONE',  ( 112.9828796295247884, -4.863998795839590272, -19.15521520033831493 ) ) ;
#29823=CARTESIAN_POINT ( 'NONE',  ( 109.0240515045248202, -6.936859964151250502, -18.39754474579286025 ) ) ;
#29828=CARTESIAN_POINT ( 'NONE',  ( 112.0105358795247810, -8.402594152722688392, -9.854619843455216355 ) ) ;
#29829=ORIENTED_EDGE ( 'NONE', *, *, #29340, .T. ) ;
#29834=ORIENTED_EDGE ( 'NONE', *, *, #6115, .T. ) ;
#29836=CARTESIAN_POINT ( 'NONE',  ( 107.2182702545248105, 0.1403307496149616695, -11.32035403202665336 ) ) ;
#29842=VECTOR ( 'NONE', #43267, 1000.000000000000000 ) ;
#29847=CARTESIAN_POINT ( 'NONE',  ( 110.8992858795247827, -8.402594152722688392, -9.854619843455216355 ) ) ;
#29855=CARTESIAN_POINT ( 'NONE',  ( 61.69189222814998175, -68.13214146720427777, -20.74076566292611545 ) ) ;
#29877=CARTESIAN_POINT ( 'NONE',  ( 112.7745202545247878, -10.62599879583958717, -15.77991374673208469 ) ) ;
#29878=CARTESIAN_POINT ( 'NONE',  ( 111.1076452545248259, -9.868328341294098749, -15.46607636864997204 ) ) ;
#29879=CARTESIAN_POINT ( 'NONE',  ( 106.9404577545248145, -2.791137627527939813, -18.39754474579286025 ) ) ;
#29882=VERTEX_POINT ( 'NONE', #24626 ) ;
#29887=CARTESIAN_POINT ( 'NONE',  ( 105.8986608795248401, -1.325403438956436419, -16.93181055722141792 ) ) ;
#29890=CARTESIAN_POINT ( 'NONE',  ( 112.3578015045248861, -2.477300249445798297, -7.631215200338321125 ) ) ;
#29900=( BOUNDED_CURVE ( )  B_SPLINE_CURVE ( 3, ( #8249, #4369, #8475, #721 ),
 .UNSPECIFIED., .F., .F. ) 
 B_SPLINE_CURVE_WITH_KNOTS ( ( 4, 4 ),
 ( 1.570796326794895004, 4.712388980384689674 ),
 .UNSPECIFIED. ) 
 CURVE ( )  GEOMETRIC_REPRESENTATION_ITEM ( )  RATIONAL_B_SPLINE_CURVE ( ( 1.000000000000000000, 0.3333333333333335369, 0.3333333333333335369, 1.000000000000000000 ) ) 
 REPRESENTATION_ITEM ( '' )  );
#29903=VERTEX_POINT ( 'NONE', #3203 ) ;
#29910=CONICAL_SURFACE ( 'NONE', #15357, 5.000000000000000888, 0.7853981633974419507 ) ;
#29913=CARTESIAN_POINT ( 'NONE',  ( 112.0799890045248475, 0.8980012041604421569, -15.77991374673208469 ) ) ;
#29920=DIRECTION ( 'NONE',  ( -1.000000000000000000, 0.000000000000000000, 0.000000000000000000 ) ) ;
#29922=CARTESIAN_POINT ( 'NONE',  ( 106.6626452545248611, 0.8980012041604421569, -11.00651665394454071 ) ) ;
#29923=CIRCLE ( 'NONE', #10281, 4.500000000000003553 ) ;
#29930=ORIENTED_EDGE ( 'NONE', *, *, #4384, .F. ) ;
#29934=CARTESIAN_POINT ( 'NONE',  ( 114.7886608795247696, -8.938348069036489818, -9.318865927141430916 ) ) ;
#29935=CARTESIAN_POINT ( 'NONE',  ( 114.2330358795247776, -8.402594152722688392, -9.854619843455216355 ) ) ;
#29936=CARTESIAN_POINT ( 'NONE',  ( 112.9134265045247645, -7.250697342233347165, -19.15521520033831138 ) ) ;
#29939=AXIS2_PLACEMENT_3D ( 'NONE', #14835, #32593, #35331 ) ;
#29942=CARTESIAN_POINT ( 'NONE',  ( 107.8433483795247838, -0.7896495226426338832, -9.318865927141430916 ) ) ;
#29946=CARTESIAN_POINT ( 'NONE',  ( 116.6234607133849295, -11.86235199658483985, -6.412683223725688109 ) ) ;
#29947=VERTEX_POINT ( 'NONE', #30183 ) ;
#29951=CARTESIAN_POINT ( 'NONE',  ( 111.9410827545248708, -6.936859964151250502, -8.388885654883777576 ) ) ;
#29952=CARTESIAN_POINT ( 'NONE',  ( 113.3301452545248083, -9.868328341294098749, -15.46607636864997204 ) ) ;
#29955=CARTESIAN_POINT ( 'NONE',  ( 69.16666358353634791, -25.68530218154914024, -5.871463680831265464 ) ) ;
#29962=EDGE_CURVE ( 'NONE', #11942, #40078, #22963, .T. ) ;
#29970=CARTESIAN_POINT ( 'NONE',  ( 106.7320983795247855, -0.7896495226426338832, -9.318865927141430916 ) ) ;
#29973=CARTESIAN_POINT ( 'NONE',  ( 107.6349890045248401, -9.868328341294098749, -11.32035403202665869 ) ) ;
#29985=CARTESIAN_POINT ( 'NONE',  ( 76.69189222814998175, -45.49566950204133065, -19.39321520033831447 ) ) ;
#29989=CARTESIAN_POINT ( 'NONE',  ( 109.9772457829843830, 0.6362173239733635022, -14.64321520033829849 ) ) ;
#29991=CARTESIAN_POINT ( 'NONE',  ( 111.5243640045248412, 0.1403307496149616695, -15.46607636864997204 ) ) ;
#29995=CARTESIAN_POINT ( 'NONE',  ( 113.3995983795247895, -8.402594152722688392, -16.93181055722141792 ) ) ;
#30000=CARTESIAN_POINT ( 'NONE',  ( 111.5938171295247940, -10.62599879583958540, -13.39321520033831447 ) ) ;
#30002=CARTESIAN_POINT ( 'NONE',  ( 115.3442858795247759, -0.7896495226426338832, -17.46756447353520159 ) ) ;
#30005=CARTESIAN_POINT ( 'NONE',  ( 105.7597546295248350, -4.863998795839590272, -7.631215200338315796 ) ) ;
#30009=CARTESIAN_POINT ( 'NONE',  ( 112.5661454522301739, 0.1168444861213632779, -14.64321520033832691 ) ) ;
#30014=ORIENTED_EDGE ( 'NONE', *, *, #23940, .T. ) ;
#30018=CARTESIAN_POINT ( 'NONE',  ( 111.3160046295247838, -4.863998795839590272, -7.631215200338315796 ) ) ;
#30021=CARTESIAN_POINT ( 'NONE',  ( 116.8068830708325692, -2.406742318435596051, -17.99911713909528643 ) ) ;
#30022=CARTESIAN_POINT ( 'NONE',  ( 63.69189222814998175, -64.02637234200076932, -46.77412892735921446 ) ) ;
#30026=EDGE_CURVE ( 'NONE', #15215, #13698, #9263, .T. ) ;
#30033=CARTESIAN_POINT ( 'NONE',  ( 105.4124890045248293, -9.868328341294098749, -11.32035403202665869 ) ) ;
#30034=CARTESIAN_POINT ( 'NONE',  ( 70.19189222814998175, -61.33395589173655793, -37.73637771078311687 ) ) ;
#30044=CARTESIAN_POINT ( 'NONE',  ( 115.2748327545248657, -6.936859964151250502, -8.388885654883777576 ) ) ;
#30046=EDGE_CURVE ( 'NONE', #12113, #41318, #34856, .T. ) ;
#30049=AXIS2_PLACEMENT_3D ( 'NONE', #43304, #5661, #5887 ) ;
#30051=CARTESIAN_POINT ( 'NONE',  ( 113.4690515045247992, -2.477300249445798297, -7.631215200338321125 ) ) ;
#30052=CARTESIAN_POINT ( 'NONE',  ( 107.0793640045248196, 0.1403307496149616695, -15.46607636864997204 ) ) ;
#30053=CARTESIAN_POINT ( 'NONE',  ( 83.24887369766287293, -31.94491598976167168, -23.46817222872420317 ) ) ;
#30057=DIRECTION ( 'NONE',  ( 1.156482317317869950E-15, 1.000000000000000000, 0.000000000000000000 ) ) ;
#30058=CARTESIAN_POINT ( 'NONE',  ( 114.0941296295247867, -4.863998795839590272, -8.388885654883775800 ) ) ;
#30067=CARTESIAN_POINT ( 'NONE',  ( 116.5635957019662357, -11.89801664228175859, -21.17206575103167765 ) ) ;
#30073=( NAMED_UNIT ( * ) PLANE_ANGLE_UNIT ( ) SI_UNIT ( $, .RADIAN. ) );
#30078=CARTESIAN_POINT ( 'NONE',  ( 112.7745202545247878, 0.1403307496149616695, -11.32035403202665336 ) ) ;
#30083=TOROIDAL_SURFACE ( 'NONE', #41747, 1.500000000000000000, 0.5000000000000000000 ) ;
#30102=EDGE_CURVE ( 'NONE', #11934, #23514, #25751, .T. ) ;
#30104=ORIENTED_EDGE ( 'NONE', *, *, #10025, .T. ) ;
#30106=CARTESIAN_POINT ( 'NONE',  ( 112.8439733795247832, -8.938348069036489818, -17.46756447353520159 ) ) ;
#30107=CARTESIAN_POINT ( 'NONE',  ( 110.6214733795247867, -1.325403438956436419, -9.854619843455211026 ) ) ;
#30108=CARTESIAN_POINT ( 'NONE',  ( 110.8298327545248299, -6.936859964151250502, -8.388885654883777576 ) ) ;
#30112=CARTESIAN_POINT ( 'NONE',  ( 64.69189222814998175, -41.76310523276723785, -7.393215200338315363 ) ) ;
#30113=CARTESIAN_POINT ( 'NONE',  ( 109.2294468747734300, -7.889554749245212939, -8.547382946171255824 ) ) ;
#30117=CARTESIAN_POINT ( 'NONE',  ( 105.4124890045248293, -9.868328341294098749, -11.32035403202665869 ) ) ;
#30120=CARTESIAN_POINT ( 'NONE',  ( 115.6220983795247861, -8.402594152722688392, -16.93181055722141792 ) ) ;
#30121=CARTESIAN_POINT ( 'NONE',  ( 61.69189222814998175, -80.85404093559408523, -31.07034979220001603 ) ) ;
#30123=FACE_OUTER_BOUND ( 'NONE', #38384, .T. ) ;
#30132=ORIENTED_EDGE ( 'NONE', *, *, #15250, .F. ) ;
#30140=CARTESIAN_POINT ( 'NONE',  ( 114.0941296295247867, -4.863998795839590272, -19.15521520033831493 ) ) ;
#30150=CARTESIAN_POINT ( 'NONE',  ( 106.5931921295248372, 0.8980012041604618078, -13.39321520033831447 ) ) ;
#30159=CARTESIAN_POINT ( 'NONE',  ( 143.3676850761856940, -41.90950876995113816, -19.14091845747268295 ) ) ;
#30160=CARTESIAN_POINT ( 'NONE',  ( 113.3301452545248083, 0.8980012041604421569, -11.00651665394454071 ) ) ;
#30161=CARTESIAN_POINT ( 'NONE',  ( 114.6497546295247929, -4.863998795839590272, -18.39754474579285315 ) ) ;
#30162=CARTESIAN_POINT ( 'NONE',  ( 112.6356140045247827, -10.62599879583958717, -11.00651665394454604 ) ) ;
#30169=CARTESIAN_POINT ( 'NONE',  ( 65.49983523453742862, -18.16718729050178993, -4.893215200338314474 ) ) ;
#30180=CARTESIAN_POINT ( 'NONE',  ( 109.0240515045248202, -6.936859964151250502, -18.39754474579286025 ) ) ;
#30181=CARTESIAN_POINT ( 'NONE',  ( 112.4967077545247633, -2.791137627527939813, -18.39754474579286025 ) ) ;
#30183=CARTESIAN_POINT ( 'NONE',  ( 67.69189222814998175, -62.82237896425675672, -47.71602681600972318 ) ) ;
#30184=CARTESIAN_POINT ( 'NONE',  ( 68.68839935636917460, -25.95913848132418522, -5.893215200338315363 ) ) ;
#30187=VERTEX_POINT ( 'NONE', #3570 ) ;
#30197=CARTESIAN_POINT ( 'NONE',  ( 107.6349890045248401, 0.8980012041604421569, -15.77991374673208469 ) ) ;
#30200=LINE ( 'NONE', #26098, #17198 ) ;
#30202=CARTESIAN_POINT ( 'NONE',  ( 108.9545983795247821, -8.402594152722688392, -16.93181055722141792 ) ) ;
#30210=VECTOR ( 'NONE', #33601, 1000.000000000000114 ) ;
#30212=DIRECTION ( 'NONE',  ( 0.000000000000000000, 0.000000000000000000, 1.000000000000000000 ) ) ;
#30214=CARTESIAN_POINT ( 'NONE',  ( 71.67504600870660170, -26.72445618319088823, -4.893215200338314474 ) ) ;
#30221=CARTESIAN_POINT ( 'NONE',  ( 106.3153796295248412, -4.863998795839590272, -8.388885654883775800 ) ) ;
#30225=CARTESIAN_POINT ( 'NONE',  ( 113.2606921295247702, -9.868328341294093420, -13.39321520033831447 ) ) ;
#30226=CARTESIAN_POINT ( 'NONE',  ( 87.44708369096657918, -25.99489077589588604, -12.39321520033831447 ) ) ;
#30228=CARTESIAN_POINT ( 'NONE',  ( 109.1629577545248395, -7.250697342233347165, -7.631215200338321125 ) ) ;
#30230=CARTESIAN_POINT ( 'NONE',  ( 116.1777233795247781, -8.938348069036489818, -17.46756447353520159 ) ) ;
#30233=CARTESIAN_POINT ( 'NONE',  ( 69.69189222814998175, -41.76310523276723785, -20.39321520033831447 ) ) ;
#30236=VERTEX_POINT ( 'NONE', #34787 ) ;
#30246=CARTESIAN_POINT ( 'NONE',  ( 107.6349890045248401, 0.8980012041604421569, -15.77991374673208469 ) ) ;
#30248=CARTESIAN_POINT ( 'NONE',  ( 116.8247182375590825, -1.639145683561697542, -17.51101245992349220 ) ) ;
#30257=CARTESIAN_POINT ( 'NONE',  ( 108.3295202545248657, 0.1403307496149616695, -11.32035403202665336 ) ) ;
#30258=CARTESIAN_POINT ( 'NONE',  ( 109.5083551332721896, 0.2334052082820642360, -14.64321520033828605 ) ) ;
#30260=VECTOR ( 'NONE', #6439, 1000.000000000000000 ) ;
#30268=CARTESIAN_POINT ( 'NONE',  ( 114.7886608795247696, -1.325403438956436419, -16.93181055722141792 ) ) ;
#30270=AXIS2_PLACEMENT_3D ( 'NONE', #3766, #4448, #32477 ) ;
#30273=CARTESIAN_POINT ( 'NONE',  ( 116.0388171295248014, -10.62599879583958540, -13.39321520033831447 ) ) ;
#30274=CARTESIAN_POINT ( 'NONE',  ( 109.9963952545248134, -9.868328341294098749, -15.46607636864997204 ) ) ;
#30275=CARTESIAN_POINT ( 'NONE',  ( 116.3860827545247787, -2.477300249445798297, -19.15521520033831138 ) ) ;
#30279=CARTESIAN_POINT ( 'NONE',  ( 113.6079577545248043, -2.791137627527939813, -18.39754474579286025 ) ) ;
#30281=CARTESIAN_POINT ( 'NONE',  ( 109.2295991976226190, -0.1639994721771769748, -15.37948311923997657 ) ) ;
#30286=DIRECTION ( 'NONE',  ( 5.948557404824750648E-16, 0.7876185884367599144, -0.6161630946014909904 ) ) ;
#30287=CARTESIAN_POINT ( 'NONE',  ( 116.5974073229478876, -11.87839771549831624, -21.20499330233542068 ) ) ;
#30296=CARTESIAN_POINT ( 'NONE',  ( 111.8716296295247901, -4.863998795839590272, -8.388885654883775800 ) ) ;
#30299=EDGE_LOOP ( 'NONE', ( #16527, #2368, #9890, #33329 ) ) ;
#30301=EDGE_CURVE ( 'NONE', #41818, #6998, #9757, .T. ) ;
#30306=EDGE_LOOP ( 'NONE', ( #10777, #6479 ) ) ;
#30308=CARTESIAN_POINT ( 'NONE',  ( 72.69189222814998175, -41.76310523276723785, -24.89321520033831447 ) ) ;
#30310=CARTESIAN_POINT ( 'NONE',  ( 79.79010115959992788, 5.106172230548759572, -14.64321520033831447 ) ) ;
#30326=CARTESIAN_POINT ( 'NONE',  ( 111.9410827545248708, -2.477300249445798297, -19.15521520033831138 ) ) ;
#30329=CARTESIAN_POINT ( 'NONE',  ( 105.5513952545248060, -9.868328341294098749, -15.46607636864997204 ) ) ;
#30330=CARTESIAN_POINT ( 'NONE',  ( 105.4819421295248247, -9.868328341294093420, -13.39321520033831447 ) ) ;
#30331=CARTESIAN_POINT ( 'NONE',  ( 64.33426790211569823, -36.45104289022312827, -5.633705335131980796 ) ) ;
#30342=CARTESIAN_POINT ( 'NONE',  ( 105.8986608795248401, -8.938348069036489818, -9.318865927141430916 ) ) ;
#30353=ORIENTED_EDGE ( 'NONE', *, *, #17211, .T. ) ;
#30365=CARTESIAN_POINT ( 'NONE',  ( 113.1912390045248031, 0.8980012041604421569, -15.77991374673208469 ) ) ;
#30367=ORIENTED_EDGE ( 'NONE', *, *, #43498, .F. ) ;
#30368=ORIENTED_EDGE ( 'NONE', *, *, #36779, .T. ) ;
#30373=CARTESIAN_POINT ( 'NONE',  ( 62.44280897409132791, -35.50444474346354440, -5.893215200338310922 ) ) ;
#30375=CARTESIAN_POINT ( 'NONE',  ( 105.5513952545248060, 0.8980012041604421569, -11.00651665394454071 ) ) ;
#30381=ORIENTED_EDGE ( 'NONE', *, *, #20585, .F. ) ;
#30385=CARTESIAN_POINT ( 'NONE',  ( 110.3436608795247764, -8.938348069036489818, -9.318865927141430916 ) ) ;
#30386=CARTESIAN_POINT ( 'NONE',  ( 112.0799890045248475, -9.868328341294098749, -11.32035403202665869 ) ) ;
#30387=CARTESIAN_POINT ( 'NONE',  ( 107.7044421295247929, 0.8980012041604618078, -13.39321520033831447 ) ) ;
#30394=CARTESIAN_POINT ( 'NONE',  ( 61.27778620743471549, -25.99489077589588604, -13.39321520033831447 ) ) ;
#30405=CARTESIAN_POINT ( 'NONE',  ( 106.6626452545248611, -9.868328341294098749, -15.46607636864997204 ) ) ;
#30406=CARTESIAN_POINT ( 'NONE',  ( 109.9269421295247753, -9.868328341294093420, -13.39321520033831447 ) ) ;
#30408=CARTESIAN_POINT ( 'NONE',  ( 69.79880589660244539, -25.73400820227583807, -5.787280954910595909 ) ) ;
#30411=VERTEX_POINT ( 'NONE', #16829 ) ;
#30418=DIRECTION ( 'NONE',  ( -1.000000000000000000, 0.000000000000000000, 3.317300593186674996E-33 ) ) ;
#30423=ADVANCED_FACE ( 'NONE', ( #30722 ), #34012, .T. ) ;
#30424=CARTESIAN_POINT ( 'NONE',  ( 108.8156921295247912, 0.8980012041604618078, -13.39321520033831447 ) ) ;
#30428=CARTESIAN_POINT ( 'NONE',  ( 107.4266296295248821, -4.863998795839590272, -8.388885654883775800 ) ) ;
#30436=CARTESIAN_POINT ( 'NONE',  ( 116.5080644685026812, 0.6938714319018670640, -14.64321520033829671 ) ) ;
#30442=ORIENTED_EDGE ( 'NONE', *, *, #7480, .T. ) ;
#30445=CARTESIAN_POINT ( 'NONE',  ( 114.9275671295247889, -10.62599879583958540, -13.39321520033831447 ) ) ;
#30449=CARTESIAN_POINT ( 'NONE',  ( 113.1912390045248031, -9.868328341294098749, -11.32035403202665869 ) ) ;
#30453=CARTESIAN_POINT ( 'NONE',  ( 109.6491296295247793, -4.863998795839590272, -19.15521520033831493 ) ) ;
#30455=CARTESIAN_POINT ( 'NONE',  ( 114.9275671295247889, -10.62599879583958540, -13.39321520033831447 ) ) ;
#30469=CARTESIAN_POINT ( 'NONE',  ( 105.8292077545248446, -7.250697342233347165, -7.631215200338321125 ) ) ;
#30470=CARTESIAN_POINT ( 'NONE',  ( 110.4131140045248287, 0.1403307496149616695, -15.46607636864997204 ) ) ;
#30474=CARTESIAN_POINT ( 'NONE',  ( 113.3995983795247895, -0.7896495226426338832, -9.318865927141430916 ) ) ;
#30478=DIRECTION ( 'NONE',  ( 0.4649787261689617424, 0.8853218534579895271, 0.000000000000000000 ) ) ;
#30481=CARTESIAN_POINT ( 'NONE',  ( 113.8627504229301763, 0.1075849324168598464, -14.64321520033831447 ) ) ;
#30482=CARTESIAN_POINT ( 'NONE',  ( 106.0375671295248310, 0.1403307496149613920, -13.39321520033831447 ) ) ;
#30491=VERTEX_POINT ( 'NONE', #16494 ) ;
#30494=DIRECTION ( 'NONE',  ( 0.9659258262890689783, 0.2588190451025185190, 0.000000000000000000 ) ) ;
#30497=CARTESIAN_POINT ( 'NONE',  ( 110.1353015045248469, -2.477300249445798297, -7.631215200338321125 ) ) ;
#30503=CARTESIAN_POINT ( 'NONE',  ( 112.7745202545247878, 0.1403307496149616695, -11.32035403202665336 ) ) ;
#30505=CARTESIAN_POINT ( 'NONE',  ( 109.2294421145928567, -0.5977367109841295045, -16.12358707770981425 ) ) ;
#30513=VERTEX_POINT ( 'NONE', #3245 ) ;
#30518=( LENGTH_UNIT ( ) NAMED_UNIT ( * ) SI_UNIT ( .MILLI., .METRE. ) );
#30519=DIRECTION ( 'NONE',  ( 0.000000000000000000, 0.000000000000000000, 1.000000000000000000 ) ) ;
#30522=CARTESIAN_POINT ( 'NONE',  ( 113.6774108795247997, -1.325403438956436419, -16.93181055722141792 ) ) ;
#30525=VERTEX_POINT ( 'NONE', #37211 ) ;
#30550=CARTESIAN_POINT ( 'NONE',  ( 105.6903015045248253, -2.477300249445798297, -7.631215200338321125 ) ) ;
#30551=CARTESIAN_POINT ( 'NONE',  ( 107.4266296295248821, -4.863998795839590272, -8.388885654883775800 ) ) ;
#30553=CARTESIAN_POINT ( 'NONE',  ( 109.3018640045248304, -10.62599879583958540, -11.00651665394454071 ) ) ;
#30555=ORIENTED_EDGE ( 'NONE', *, *, #40924, .T. ) ;
#30563=CARTESIAN_POINT ( 'NONE',  ( 107.4266296295248821, -4.863998795839590272, -19.15521520033831493 ) ) ;
#30566=CARTESIAN_POINT ( 'NONE',  ( 70.19189222814998175, -65.04786711941002864, -39.22192925581976652 ) ) ;
#30574=VERTEX_POINT ( 'NONE', #37448 ) ;
#30576=CIRCLE ( 'NONE', #31312, 1.999999999999999112 ) ;
#30583=CARTESIAN_POINT ( 'NONE',  ( 110.4131140045248287, -10.62599879583958717, -11.00651665394454604 ) ) ;
#30606=EDGE_CURVE ( 'NONE', #3191, #27343, #27907, .T. ) ;
#30608=CARTESIAN_POINT ( 'NONE',  ( 108.4684265045247997, -7.250697342233347165, -19.15521520033831138 ) ) ;
#30609=CARTESIAN_POINT ( 'NONE',  ( 112.4967077545247633, -2.791137627527939813, -18.39754474579286025 ) ) ;
#30610=CARTESIAN_POINT ( 'NONE',  ( 107.5655358795247736, -0.7896495226426338832, -17.46756447353520159 ) ) ;
#30615=ADVANCED_FACE ( 'NONE', ( #33559 ), #9645, .F. ) ;
#30630=CARTESIAN_POINT ( 'NONE',  ( 108.8156921295247912, -9.868328341294093420, -13.39321520033831447 ) ) ;
#30631=CARTESIAN_POINT ( 'NONE',  ( 112.7745202545247878, 0.1403307496149616695, -11.32035403202665336 ) ) ;
#30641=ORIENTED_EDGE ( 'NONE', *, *, #23359, .T. ) ;
#30646=( BOUNDED_CURVE ( )  B_SPLINE_CURVE ( 3, ( #26472, #40837, #19619, #20084 ),
 .UNSPECIFIED., .F., .F. ) 
 B_SPLINE_CURVE_WITH_KNOTS ( ( 4, 4 ),
 ( 1.534323482254100091, 1.570796326794904996 ),
 .UNSPECIFIED. ) 
 CURVE ( )  GEOMETRIC_REPRESENTATION_ITEM ( )  RATIONAL_B_SPLINE_CURVE ( ( 1.000000000000000000, 0.9998891473731379431, 0.9998891473731379431, 1.000000000000000000 ) ) 
 REPRESENTATION_ITEM ( '' )  );
#30648=DIRECTION ( 'NONE',  ( 0.000000000000000000, 0.000000000000000000, 1.000000000000000000 ) ) ;
#30654=CARTESIAN_POINT ( 'NONE',  ( 116.2471765045247594, -7.250697342233347165, -19.15521520033831138 ) ) ;
#30665=CARTESIAN_POINT ( 'NONE',  ( 113.8604010812576774, -0.01829820670803256055, -12.14321520033831625 ) ) ;
#30671=CARTESIAN_POINT ( 'NONE',  ( 115.9693640045247776, -10.62599879583958717, -11.00651665394454604 ) ) ;
#30676=CARTESIAN_POINT ( 'NONE',  ( 115.4831921295247952, -9.868328341294093420, -13.39321520033831447 ) ) ;
#30684=CARTESIAN_POINT ( 'NONE',  ( 113.4690515045247992, -2.477300249445798297, -7.631215200338321125 ) ) ;
#30687=EDGE_CURVE ( 'NONE', #20884, #42739, #18417, .T. ) ;
#30690=EDGE_LOOP ( 'NONE', ( #42818, #30368, #30014, #39205 ) ) ;
#30697=VERTEX_POINT ( 'NONE', #7114 ) ;
#30699=CARTESIAN_POINT ( 'NONE',  ( 105.9681140045248355, -10.62599879583958717, -11.00651665394454604 ) ) ;
#30702=CARTESIAN_POINT ( 'NONE',  ( 112.2883483795247770, -0.7896495226426338832, -9.318865927141430916 ) ) ;
#30708=CARTESIAN_POINT ( 'NONE',  ( 116.4217710891409610, 2.238304050683879609, -6.396164327732187793 ) ) ;
#30710=CARTESIAN_POINT ( 'NONE',  ( 109.0240515045248202, -6.936859964151250502, -18.39754474579286025 ) ) ;
#30711=ADVANCED_FACE ( 'NONE', ( #28316, #710 ), #38123, .F. ) ;
#30712=DIRECTION ( 'NONE',  ( 0.000000000000000000, 0.000000000000000000, 1.000000000000000000 ) ) ;
#30722=FACE_OUTER_BOUND ( 'NONE', #1602, .T. ) ;
#30725=CARTESIAN_POINT ( 'NONE',  ( 112.5661608795247872, -8.938348069036489818, -9.318865927141430916 ) ) ;
#30726=CARTESIAN_POINT ( 'NONE',  ( 62.22678445075433018, -36.72958069525633817, -5.531797115907686191 ) ) ;
#30727=CARTESIAN_POINT ( 'NONE',  ( 116.0388171295248014, -10.62599879583958540, -13.39321520033831447 ) ) ;
#30730=EDGE_CURVE ( 'NONE', #13043, #4906, #34685, .T. ) ;
#30732=CARTESIAN_POINT ( 'NONE',  ( 113.4690515045247992, -6.936859964151250502, -18.39754474579286025 ) ) ;
#30741=CARTESIAN_POINT ( 'NONE',  ( 116.8309807853375588, -11.70023447154984453, -21.43868405042244163 ) ) ;
#30747=CARTESIAN_POINT ( 'NONE',  ( 92.26512299712632625, -23.76310523276723785, -6.893215200338315363 ) ) ;
#30750=CARTESIAN_POINT ( 'NONE',  ( 116.5944421295247793, 0.8980012041604618078, -13.39321520033831447 ) ) ;
#30760=CYLINDRICAL_SURFACE ( 'NONE', #31085, 1.299999999999995604 ) ;
#30764=CARTESIAN_POINT ( 'NONE',  ( 78.69189222814998175, -48.76310523276723785, -23.89321520033831803 ) ) ;
#30776=ORIENTED_EDGE ( 'NONE', *, *, #17831, .T. ) ;
#30778=CARTESIAN_POINT ( 'NONE',  ( 106.9404577545248145, -7.250697342233347165, -7.631215200338321125 ) ) ;
#30779=CARTESIAN_POINT ( 'NONE',  ( 107.3571765045248299, -2.791137627527939813, -8.388885654883777576 ) ) ;
#30786=CARTESIAN_POINT ( 'NONE',  ( 116.4555358795247884, -8.402594152722633325, -9.854619843455179051 ) ) ;
#30791=CARTESIAN_POINT ( 'NONE',  ( 115.3442858795247759, -8.402594152722688392, -9.854619843455216355 ) ) ;
#30800=DIRECTION ( 'NONE',  ( -1.000000000000000000, 0.000000000000000000, 0.000000000000000000 ) ) ;
#30802=ORIENTED_EDGE ( 'NONE', *, *, #37729, .T. ) ;
#30812=CARTESIAN_POINT ( 'NONE',  ( 108.3989733795248753, -8.938348069036489818, -17.46756447353520159 ) ) ;
#30828=CARTESIAN_POINT ( 'NONE',  ( 109.2294421295247844, -9.051693226400931991, -21.89321520033831447 ) ) ;
#30832=CARTESIAN_POINT ( 'NONE',  ( 116.0831764669098760, -0.01868118798763890309, -12.14321520033834290 ) ) ;
#30833=CARTESIAN_POINT ( 'NONE',  ( 110.5520202545248054, -10.62599879583958717, -15.77991374673208469 ) ) ;
#30834=CARTESIAN_POINT ( 'NONE',  ( 113.6774108795247997, -1.325403438956436419, -16.93181055722141792 ) ) ;
#30835=CARTESIAN_POINT ( 'NONE',  ( 115.8304577545247582, -2.791137627527939813, -18.39754474579286025 ) ) ;
#30838=ORIENTED_EDGE ( 'NONE', *, *, #14986, .T. ) ;
#30840=CARTESIAN_POINT ( 'NONE',  ( 112.5661608795247872, -8.938348069036489818, -9.318865927141430916 ) ) ;
#30848=CARTESIAN_POINT ( 'NONE',  ( 106.2459265045248173, -7.250697342233347165, -19.15521520033831138 ) ) ;
#30854=CARTESIAN_POINT ( 'NONE',  ( 108.2600671295247992, 0.1403307496149613920, -13.39321520033831447 ) ) ;
#30855=CARTESIAN_POINT ( 'NONE',  ( 106.5931921295248372, -9.868328341294093420, -13.39321520033831447 ) ) ;
#30860=ADVANCED_FACE ( 'NONE', ( #39019, #34897 ), #25123, .F. ) ;
#30864=ORIENTED_EDGE ( 'NONE', *, *, #24838, .F. ) ;
#30866=CIRCLE ( 'NONE', #7581, 5.000000000000004441 ) ;
#30873=EDGE_CURVE ( 'NONE', #14918, #16653, #20806, .T. ) ;
#30878=CARTESIAN_POINT ( 'NONE',  ( 114.1635827545248389, -2.477300249445798297, -19.15521520033831138 ) ) ;
#30886=CARTESIAN_POINT ( 'NONE',  ( 111.9228860982116913, 0.3867979994853637526, -12.14321520033831625 ) ) ;
#30888=CARTESIAN_POINT ( 'NONE',  ( 65.54186577906706646, -36.42801838861263519, -5.470407532193676481 ) ) ;
#30889=DIRECTION ( 'NONE',  ( 0.000000000000000000, 0.000000000000000000, -1.000000000000000000 ) ) ;
#30891=ORIENTED_EDGE ( 'NONE', *, *, #33209, .F. ) ;
#30894=CARTESIAN_POINT ( 'NONE',  ( 116.1082702545247827, -10.62599879583958717, -15.77991374673208469 ) ) ;
#30898=CARTESIAN_POINT ( 'NONE',  ( 114.9970202545248412, 0.1403307496149616695, -11.32035403202665336 ) ) ;
#30900=CARTESIAN_POINT ( 'NONE',  ( 111.5243640045248412, -10.62599879583958540, -11.00651665394455492 ) ) ;
#30901=CARTESIAN_POINT ( 'NONE',  ( 109.2296643047792060, -2.144085356277730448, -17.65426957299811761 ) ) ;
#30903=CARTESIAN_POINT ( 'NONE',  ( 106.8015515045248378, -2.477300249445798297, -7.631215200338321125 ) ) ;
#30905=CARTESIAN_POINT ( 'NONE',  ( 110.4131140045248287, -10.62599879583958717, -11.00651665394454604 ) ) ;
#30908=CARTESIAN_POINT ( 'NONE',  ( 114.4099712410415748, 0.7607806665037644134, -12.14321520033829316 ) ) ;
#30920=ORIENTED_EDGE ( 'NONE', *, *, #31239, .T. ) ;
#30924=CARTESIAN_POINT ( 'NONE',  ( 114.3024890045248156, 0.8980012041604421569, -15.77991374673208469 ) ) ;
#30926=ADVANCED_FACE ( 'NONE', ( #33053 ), #15757, .F. ) ;
#30927=EDGE_CURVE ( 'NONE', #2865, #44361, #42343, .T. ) ;
#30930=DIRECTION ( 'NONE',  ( 0.07634843047859296572, 0.9970811988817437355, 0.000000000000000000 ) ) ;
#30931=CARTESIAN_POINT ( 'NONE',  ( 92.26512299712632625, -23.76310523276723785, -21.89321520033831447 ) ) ;
#30934=CARTESIAN_POINT ( 'NONE',  ( 116.0286950891469786, 2.331313199634366118, -6.893215200338315363 ) ) ;
#30936=CARTESIAN_POINT ( 'NONE',  ( 107.9822546295247889, -4.863998795839590272, -18.39754474579285315 ) ) ;
#30949=CARTESIAN_POINT ( 'NONE',  ( 109.5796765045248122, -7.250697342233347165, -19.15521520033831138 ) ) ;
#30951=CARTESIAN_POINT ( 'NONE',  ( 115.4137390045248566, 0.8980012041604421569, -15.77991374673208469 ) ) ;
#30957=CARTESIAN_POINT ( 'NONE',  ( 111.2465515045248168, -6.936859964151250502, -18.39754474579286025 ) ) ;
#30961=DIRECTION ( 'NONE',  ( -0.6383198453882299450, -0.7697712484781087383, 0.000000000000000000 ) ) ;
#30970=DIRECTION ( 'NONE',  ( -1.000000000000000000, 0.000000000000000000, 0.000000000000000000 ) ) ;
#30974=CARTESIAN_POINT ( 'NONE',  ( 106.3153796295248412, -4.863998795839590272, -8.388885654883775800 ) ) ;
#30976=DIRECTION ( 'NONE',  ( 0.000000000000000000, 0.000000000000000000, -1.000000000000000000 ) ) ;
#30983=CARTESIAN_POINT ( 'NONE',  ( 115.1359265045248605, -7.250697342233347165, -19.15521520033831138 ) ) ;
#30984=CARTESIAN_POINT ( 'NONE',  ( 111.0762212410415799, 0.7607806665037644134, -12.14321520033829316 ) ) ;
#30985=DIRECTION ( 'NONE',  ( 0.000000000000000000, 0.000000000000000000, -1.000000000000000000 ) ) ;
#30986=DIRECTION ( 'NONE',  ( -0.8853218534579893051, 0.4649787261689617979, 0.000000000000000000 ) ) ;
#30987=CARTESIAN_POINT ( 'NONE',  ( 78.05848382472312608, -57.67750005573411443, -0.9577251715239786245 ) ) ;
#31000=CARTESIAN_POINT ( 'NONE',  ( 106.0375671295248310, -10.62599879583958540, -13.39321520033831447 ) ) ;
#31001=DIRECTION ( 'NONE',  ( 0.000000000000000000, -0.3713878862591665220, 0.9284778069183713400 ) ) ;
#31002=CARTESIAN_POINT ( 'NONE',  ( 105.2041296295248287, -4.863998795839590272, -8.388885654883775800 ) ) ;
#31009=CARTESIAN_POINT ( 'NONE',  ( 107.1488171295247867, -10.62599879583958540, -13.39321520033831447 ) ) ;
#31029=CARTESIAN_POINT ( 'NONE',  ( 106.9404577545248145, -7.250697342233347165, -7.631215200338321125 ) ) ;
#31038=CARTESIAN_POINT ( 'NONE',  ( 63.69189222814998175, -57.16572941273946640, -4.036072343195455936 ) ) ;
#31041=CARTESIAN_POINT ( 'NONE',  ( 69.69189222814998175, -41.76310523276723785, -24.89321520033831447 ) ) ;
#31051=CARTESIAN_POINT ( 'NONE',  ( 106.2459265045248173, -7.250697342233347165, -19.15521520033831138 ) ) ;
#31052=CARTESIAN_POINT ( 'NONE',  ( 108.6767858795247861, -8.402594152722688392, -9.854619843455216355 ) ) ;
#31053=CARTESIAN_POINT ( 'NONE',  ( 109.5102233795247884, -8.938348069036489818, -17.46756447353520159 ) ) ;
#31059=CARTESIAN_POINT ( 'NONE',  ( 111.5243640045248412, -10.62599879583958717, -11.00651665394454604 ) ) ;
#31062=DIRECTION ( 'NONE',  ( 1.000000000000000000, 0.000000000000000000, 0.000000000000000000 ) ) ;
#31066=CARTESIAN_POINT ( 'NONE',  ( 113.8857702545248003, 0.1403307496149616695, -11.32035403202665336 ) ) ;
#31072=CARTESIAN_POINT ( 'NONE',  ( 106.5931921295248372, -9.868328341294093420, -13.39321520033831447 ) ) ;
#31073=CARTESIAN_POINT ( 'NONE',  ( 105.1346765045248475, -2.791137627527939813, -8.388885654883777576 ) ) ;
#31078=AXIS2_PLACEMENT_3D ( 'NONE', #25684, #29549, #15419 ) ;
#31081=FACE_OUTER_BOUND ( 'NONE', #34904, .T. ) ;
#31084=CARTESIAN_POINT ( 'NONE',  ( 78.29371559379768541, 3.878430683262009016, -4.893215200338310922 ) ) ;
#31085=AXIS2_PLACEMENT_3D ( 'NONE', #2484, #41043, #37601 ) ;
#31086=ORIENTED_EDGE ( 'NONE', *, *, #6693, .F. ) ;
#31089=( BOUNDED_SURFACE ( )  B_SPLINE_SURFACE ( 1, 2, ( 
 ( #44241, #17263, #24544, #24758, #38647, #7200, #21564, #21339, #38432, #24328, #3998, #28194, #17697, #38214, #31817, #10640, #35224, #27972, #7418, #28412, #14499, #142, #17473, #20684, #45073, #6774, #17920, #20903, #21113, #34561, #34987, #3773, #31595, #589, #6992, #3344, #42321, #41664, #26896, #364, #40816, #27748, #11083, #24985, #13833, #14275, #4226, #35451, #41878, #34777, #42100, #38879, #10421, #10863, #3560, #7649, #18145, #9572, #23488, #31370, #14056, #32040, #29530, #28861, #807, #11985, #8334, #22683, #25215, #36581, #14725, #39114, #28638, #15171, #15624, #18815, #22233, #22459, #1703, #1260, #39788, #32486, #43445, #4673, #35908, #42773, #5124, #4898, #29304, #40014, #32706, #36129, #5357, #25886, #32927, #39345, #42545, #22013, #12209, #11306, #21790, #25666, #18594, #7882, #1479, #35682, #29077, #4456, #15400, #36353, #19040, #42989, #26107, #8558, #18377, #11756, #39571, #8779, #32265, #43217, #1033, #14950, #11536, #25443, #8112, #33152, #1928, #15854, #29750, #43662, #40244, #9013, #22910, #19273, #12438, #26337, #36803, #28463, #31416, #7037, #14546, #183, #6820, #38473, #409, #44908, #38700, #10688, #35039, #24590, #38927, #21613, #13879, #24369, #24152, #41923, #7249, #14325, #17967, #25035, #7468 ),
 ( #20727, #31866, #20947, #42371, #42148, #10468, #633, #21162, #31640, #35500, #35268, #24808, #11132, #7698, #34607, #17091, #17311, #3820, #21385, #3392, #10908, #30983, #4045, #17744, #41703, #13665, #28239, #27574, #38256, #41486, #28017, #10244, #14100, #38044, #31201, #45123, #17519, #34821, #27790, #3604, #35124, #35354, #38336, #13963, #16946, #21023, #21247, #7328, #20805, #3907, #38552, #34465, #6895, #34684, #24665, #492, #31276, #7113, #30840, #27431, #31499, #6679, #37901, #3244, #17170, #44987, #3472, #10769, #31722, #14405, #44763, #34896, #28315, #31059, #42227, #49, #17387, #10990, #27874, #20587, #3685, #270, #13522, #17825, #10545, #17606, #24445, #38785, #21471, #13746, #24231, #24013, #41788, #14179, #28097, #24892, #7556, #41353, #27654, #42005, #10109, #41569, #10328, #38122, #28547, #39698, #709, #39018, #22144, #4805, #18726, #1384, #14629, #36036, #43117, #39473, #15299, #25567, #35583, #32618, #32394, #29208, #18504, #22587, #11887, #32834, #4130, #1603, #940, #18050, #25789, #8237, #39922, #42451, #8683, #31943, #11217, #25122, #1163, #15523, #8463, #22366, #36262, #18944, #15079, #5029, #4579, #29430, #21916, #8007, #7788, #21697, #43344, #12114, #26017, #4355, #18275, #32171, #14859, #28768, #42674 ) ),
 .UNSPECIFIED., .F., .F., .F. ) 
 B_SPLINE_SURFACE_WITH_KNOTS ( ( 2, 2 ),
 ( 3, 2, 2, 2, 2, 2, 2, 2, 2, 2, 2, 2, 2, 2, 2, 2, 2, 2, 2, 2, 2, 2, 2, 2, 2, 2, 2, 2, 2, 2, 2, 2, 2, 2, 2, 2, 2, 2, 2, 2, 2, 2, 2, 2, 2, 2, 2, 2, 2, 2, 2, 2, 2, 2, 2, 2, 2, 2, 2, 2, 2, 2, 2, 2, 2, 2, 2, 2, 2, 2, 2, 2, 2, 2, 2, 2, 2, 2, 2, 2, 3 ),
 ( 0.000000000000000000, 1.000000000000000000 ),
 ( 0.000000000000000000, 0.01250000000000000069, 0.02500000000000000139, 0.03749999999999999861, 0.05000000000000000278, 0.06250000000000000000, 0.07499999999999999722, 0.08749999999999999445, 0.1000000000000000056, 0.1125000000000000028, 0.1250000000000000000, 0.1375000000000000111, 0.1499999999999999944, 0.1625000000000000056, 0.1749999999999999889, 0.1875000000000000000, 0.2000000000000000111, 0.2124999999999999944, 0.2250000000000000056, 0.2374999999999999889, 0.2500000000000000000, 0.2625000000000000111, 0.2750000000000000222, 0.2874999999999999778, 0.2999999999999999889, 0.3125000000000000000, 0.3250000000000000111, 0.3375000000000000222, 0.3499999999999999778, 0.3624999999999999889, 0.3750000000000000000, 0.3875000000000000111, 0.4000000000000000222, 0.4124999999999999778, 0.4249999999999999889, 0.4375000000000000000, 0.4500000000000000111, 0.4625000000000000222, 0.4749999999999999778, 0.4874999999999999889, 0.5000000000000000000, 0.5124999999999999556, 0.5250000000000000222, 0.5374999999999999778, 0.5500000000000000444, 0.5625000000000000000, 0.5749999999999999556, 0.5875000000000000222, 0.5999999999999999778, 0.6125000000000000444, 0.6250000000000000000, 0.6374999999999999556, 0.6500000000000000222, 0.6624999999999999778, 0.6750000000000000444, 0.6875000000000000000, 0.6999999999999999556, 0.7125000000000000222, 0.7249999999999999778, 0.7375000000000000444, 0.7500000000000000000, 0.7624999999999999556, 0.7750000000000000222, 0.7874999999999999778, 0.8000000000000000444, 0.8125000000000000000, 0.8249999999999999556, 0.8375000000000000222, 0.8499999999999999778, 0.8625000000000000444, 0.8750000000000000000, 0.8874999999999999556, 0.9000000000000000222, 0.9124999999999999778, 0.9250000000000000444, 0.9375000000000000000, 0.9499999999999999556, 0.9625000000000000222, 0.9749999999999999778, 0.9875000000000000444, 1.000000000000000000 ),
 .UNSPECIFIED. ) 
 GEOMETRIC_REPRESENTATION_ITEM ( )  RATIONAL_B_SPLINE_SURFACE ( (
 ( 1.000000000000000000, 0.9238795325112869605, 1.000000000000000000, 0.9238795325112869605, 1.000000000000000000, 0.9238795325112869605, 1.000000000000000000, 0.9238795325112869605, 1.000000000000000000, 0.9238795325112869605, 1.000000000000000000, 0.9238795325112869605, 1.000000000000000000, 0.9238795325112869605, 1.000000000000000000, 0.9238795325112869605, 1.000000000000000000, 0.9238795325112869605, 1.000000000000000000, 0.9238795325112869605, 1.000000000000000000, 0.9238795325112869605, 1.000000000000000000, 0.9238795325112869605, 1.000000000000000000, 0.9238795325112869605, 1.000000000000000000, 0.9238795325112869605, 1.000000000000000000, 0.9238795325112869605, 1.000000000000000000, 0.9238795325112869605, 1.000000000000000000, 0.9238795325112869605, 1.000000000000000000, 0.9238795325112869605, 1.000000000000000000, 0.9238795325112869605, 1.000000000000000000, 0.9238795325112869605, 1.000000000000000000, 0.9238795325112869605, 1.000000000000000000, 0.9238795325112869605, 1.000000000000000000, 0.9238795325112869605, 1.000000000000000000, 0.9238795325112869605, 1.000000000000000000, 0.9238795325112869605, 1.000000000000000000, 0.9238795325112869605, 1.000000000000000000, 0.9238795325112869605, 1.000000000000000000, 0.9238795325112869605, 1.000000000000000000, 0.9238795325112869605, 1.000000000000000000, 0.9238795325112869605, 1.000000000000000000, 0.9238795325112869605, 1.000000000000000000, 0.9238795325112869605, 1.000000000000000000, 0.9238795325112869605, 1.000000000000000000, 0.9238795325112869605, 1.000000000000000000, 0.9238795325112869605, 1.000000000000000000, 0.9238795325112869605, 1.000000000000000000, 0.9238795325112869605, 1.000000000000000000, 0.9238795325112869605, 1.000000000000000000, 0.9238795325112869605, 1.000000000000000000, 0.9238795325112869605, 1.000000000000000000, 0.9238795325112869605, 1.000000000000000000, 0.9238795325112869605, 1.000000000000000000, 0.9238795325112869605, 1.000000000000000000, 0.9238795325112869605, 1.000000000000000000, 0.9238795325112869605, 1.000000000000000000, 0.9238795325112869605, 1.000000000000000000, 0.9238795325112869605, 1.000000000000000000, 0.9238795325112869605, 1.000000000000000000, 0.9238795325112869605, 1.000000000000000000, 0.9238795325112869605, 1.000000000000000000, 0.9238795325112869605, 1.000000000000000000, 0.9238795325112869605, 1.000000000000000000, 0.9238795325112869605, 1.000000000000000000, 0.9238795325112869605, 1.000000000000000000, 0.9238795325112869605, 1.000000000000000000, 0.9238795325112869605, 1.000000000000000000, 0.9238795325112869605, 1.000000000000000000, 0.9238795325112869605, 1.000000000000000000, 0.9238795325112869605, 1.000000000000000000, 0.9238795325112869605, 1.000000000000000000, 0.9238795325112869605, 1.000000000000000000, 0.9238795325112869605, 1.000000000000000000, 0.9238795325112869605, 1.000000000000000000, 0.9238795325112869605, 1.000000000000000000, 0.9238795325112869605, 1.000000000000000000, 0.9238795325112869605, 1.000000000000000000, 0.9238795325112869605, 1.000000000000000000, 0.9238795325112869605, 1.000000000000000000, 0.9238795325112869605, 1.000000000000000000, 0.9238795325112869605, 1.000000000000000000, 0.9238795325112869605, 1.000000000000000000, 0.9238795325112869605, 1.000000000000000000, 0.9238795325112869605, 1.000000000000000000, 0.9238795325112869605, 1.000000000000000000, 0.9238795325112869605, 1.000000000000000000, 0.9238795325112869605, 1.000000000000000000, 0.9238795325112869605, 1.000000000000000000, 0.9238795325112869605, 1.000000000000000000, 0.9238795325112869605, 1.000000000000000000, 0.9238795325112869605, 1.000000000000000000),
 ( 1.000000000000000000, 0.9238795325112869605, 1.000000000000000000, 0.9238795325112869605, 1.000000000000000000, 0.9238795325112869605, 1.000000000000000000, 0.9238795325112869605, 1.000000000000000000, 0.9238795325112869605, 1.000000000000000000, 0.9238795325112869605, 1.000000000000000000, 0.9238795325112869605, 1.000000000000000000, 0.9238795325112869605, 1.000000000000000000, 0.9238795325112869605, 1.000000000000000000, 0.9238795325112869605, 1.000000000000000000, 0.9238795325112869605, 1.000000000000000000, 0.9238795325112869605, 1.000000000000000000, 0.9238795325112869605, 1.000000000000000000, 0.9238795325112869605, 1.000000000000000000, 0.9238795325112869605, 1.000000000000000000, 0.9238795325112869605, 1.000000000000000000, 0.9238795325112869605, 1.000000000000000000, 0.9238795325112869605, 1.000000000000000000, 0.9238795325112869605, 1.000000000000000000, 0.9238795325112869605, 1.000000000000000000, 0.9238795325112869605, 1.000000000000000000, 0.9238795325112869605, 1.000000000000000000, 0.9238795325112869605, 1.000000000000000000, 0.9238795325112869605, 1.000000000000000000, 0.9238795325112869605, 1.000000000000000000, 0.9238795325112869605, 1.000000000000000000, 0.9238795325112869605, 1.000000000000000000, 0.9238795325112869605, 1.000000000000000000, 0.9238795325112869605, 1.000000000000000000, 0.9238795325112869605, 1.000000000000000000, 0.9238795325112869605, 1.000000000000000000, 0.9238795325112869605, 1.000000000000000000, 0.9238795325112869605, 1.000000000000000000, 0.9238795325112869605, 1.000000000000000000, 0.9238795325112869605, 1.000000000000000000, 0.9238795325112869605, 1.000000000000000000, 0.9238795325112869605, 1.000000000000000000, 0.9238795325112869605, 1.000000000000000000, 0.9238795325112869605, 1.000000000000000000, 0.9238795325112869605, 1.000000000000000000, 0.9238795325112869605, 1.000000000000000000, 0.9238795325112869605, 1.000000000000000000, 0.9238795325112869605, 1.000000000000000000, 0.9238795325112869605, 1.000000000000000000, 0.9238795325112869605, 1.000000000000000000, 0.9238795325112869605, 1.000000000000000000, 0.9238795325112869605, 1.000000000000000000, 0.9238795325112869605, 1.000000000000000000, 0.9238795325112869605, 1.000000000000000000, 0.9238795325112869605, 1.000000000000000000, 0.9238795325112869605, 1.000000000000000000, 0.9238795325112869605, 1.000000000000000000, 0.9238795325112869605, 1.000000000000000000, 0.9238795325112869605, 1.000000000000000000, 0.9238795325112869605, 1.000000000000000000, 0.9238795325112869605, 1.000000000000000000, 0.9238795325112869605, 1.000000000000000000, 0.9238795325112869605, 1.000000000000000000, 0.9238795325112869605, 1.000000000000000000, 0.9238795325112869605, 1.000000000000000000, 0.9238795325112869605, 1.000000000000000000, 0.9238795325112869605, 1.000000000000000000, 0.9238795325112869605, 1.000000000000000000, 0.9238795325112869605, 1.000000000000000000, 0.9238795325112869605, 1.000000000000000000, 0.9238795325112869605, 1.000000000000000000, 0.9238795325112869605, 1.000000000000000000, 0.9238795325112869605, 1.000000000000000000, 0.9238795325112869605, 1.000000000000000000, 0.9238795325112869605, 1.000000000000000000, 0.9238795325112869605, 1.000000000000000000, 0.9238795325112869605, 1.000000000000000000, 0.9238795325112869605, 1.000000000000000000, 0.9238795325112869605, 1.000000000000000000, 0.9238795325112869605, 1.000000000000000000, 0.9238795325112869605, 1.000000000000000000, 0.9238795325112869605, 1.000000000000000000, 0.9238795325112869605, 1.000000000000000000, 0.9238795325112869605, 1.000000000000000000, 0.9238795325112869605, 1.000000000000000000) ) ) 
 REPRESENTATION_ITEM ( '' )  SURFACE ( )  );
#31095=CARTESIAN_POINT ( 'NONE',  ( 113.8163171295247764, -10.62599879583958540, -13.39321520033831447 ) ) ;
#31097=CARTESIAN_POINT ( 'NONE',  ( 115.0207045411902413, -0.3595008806742185925, -10.82052240173742064 ) ) ;
#31104=CARTESIAN_POINT ( 'NONE',  ( 85.82609049628328535, -26.41178087463453750, -7.893215200339676052 ) ) ;
#31105=CARTESIAN_POINT ( 'NONE',  ( 64.43535090723580083, -36.95092036245521427, -5.467054258871676176 ) ) ;
#31108=ORIENTED_EDGE ( 'NONE', *, *, #28630, .T. ) ;
#31111=CARTESIAN_POINT ( 'NONE',  ( 115.2053796295247849, -4.863998795839590272, -19.15521520033831493 ) ) ;
#31117=CARTESIAN_POINT ( 'NONE',  ( 109.7185827545247889, -6.936859964151250502, -8.388885654883777576 ) ) ;
#31118=CARTESIAN_POINT ( 'NONE',  ( 111.6632702545248605, -10.62599879583958540, -15.77991374673208469 ) ) ;
#31122=DIRECTION ( 'NONE',  ( 0.3445294493088594256, 0.9387755102040817867, 0.000000000000000000 ) ) ;
#31123=CARTESIAN_POINT ( 'NONE',  ( 109.3018640045248304, -10.62599879583958717, -11.00651665394454604 ) ) ;
#31126=CARTESIAN_POINT ( 'NONE',  ( 111.6402504229301940, 0.1075849324168598464, -14.64321520033829671 ) ) ;
#31128=EDGE_CURVE ( 'NONE', #44558, #7488, #19776, .T. ) ;
#31130=ORIENTED_EDGE ( 'NONE', *, *, #38212, .F. ) ;
#31139=CARTESIAN_POINT ( 'NONE',  ( 116.8567633678298705, -0.4761927928726716885, -16.29842386168302681 ) ) ;
#31140=CARTESIAN_POINT ( 'NONE',  ( 112.5661608795247872, -8.938348069036489818, -9.318865927141430916 ) ) ;
#31141=EDGE_LOOP ( 'NONE', ( #30920, #28254, #7121, #9678, #18520, #22681 ) ) ;
#31146=CARTESIAN_POINT ( 'NONE',  ( 70.19189222814998175, -63.19092768811421479, -43.86431829041166708 ) ) ;
#31157=CARTESIAN_POINT ( 'NONE',  ( 115.8111041094426810, 0.3591747506842615789, -12.14321520033831625 ) ) ;
#31161=EDGE_LOOP ( 'NONE', ( #7387, #26441, #25565, #8300 ) ) ;
#31166=EDGE_CURVE ( 'NONE', #44941, #35019, #32619, .T. ) ;
#31168=CARTESIAN_POINT ( 'NONE',  ( 112.3578015045248861, -2.477300249445798297, -7.631215200338321125 ) ) ;
#31169=CARTESIAN_POINT ( 'NONE',  ( 106.4542858795248179, -8.402594152722688392, -9.854619843455216355 ) ) ;
#31170=CARTESIAN_POINT ( 'NONE',  ( 113.8857702545248003, -10.62599879583958717, -15.77991374673208469 ) ) ;
#31173=CARTESIAN_POINT ( 'NONE',  ( 109.2294421295247844, -8.865838614420134434, -9.247624522711900497 ) ) ;
#31175=CARTESIAN_POINT ( 'NONE',  ( 110.8992858795247827, -8.402594152722688392, -9.854619843455216355 ) ) ;
#31176=ADVANCED_FACE ( 'NONE', ( #19173 ), #11888, .F. ) ;
#31184=CARTESIAN_POINT ( 'NONE',  ( 113.2987212410415765, 0.7607806665037644134, -12.14321520033829493 ) ) ;
#31193=CARTESIAN_POINT ( 'NONE',  ( 107.2182702545248105, 0.1403307496149616695, -11.32035403202665336 ) ) ;
#31196=EDGE_LOOP ( 'NONE', ( #26091, #25673, #41239, #678, #4212, #22467, #8144, #34198, #16334, #6273, #15116, #20075, #16177, #32453, #10508, #33322, #11733 ) ) ;
#31201=CARTESIAN_POINT ( 'NONE',  ( 114.2330358795247776, -0.7896495226426338832, -17.46756447353520159 ) ) ;
#31205=CARTESIAN_POINT ( 'NONE',  ( 78.69189222814998175, -59.80879295971297438, 0.4535904759388441621 ) ) ;
#31207=CARTESIAN_POINT ( 'NONE',  ( 115.9294421295247872, 1.035107641088057973, -14.64321520033831447 ) ) ;
#31209=ADVANCED_FACE ( 'NONE', ( #37626 ), #23735, .F. ) ;
#31217=CARTESIAN_POINT ( 'NONE',  ( 105.8292077545248446, -7.250697342233347165, -7.631215200338321125 ) ) ;
#31218=CARTESIAN_POINT ( 'NONE',  ( 106.5237390045248418, -9.868328341294098749, -11.32035403202665869 ) ) ;
#31229=CARTESIAN_POINT ( 'NONE',  ( 112.3578015045248861, -6.936859964151250502, -18.39754474579286025 ) ) ;
#31238=DIRECTION ( 'NONE',  ( 0.000000000000000000, 0.000000000000000000, -1.000000000000000000 ) ) ;
#31239=EDGE_CURVE ( 'NONE', #408, #31466, #2510, .T. ) ;
#31249=CARTESIAN_POINT ( 'NONE',  ( 106.4542858795248179, -0.7896495226426338832, -17.46756447353520159 ) ) ;
#31252=ORIENTED_EDGE ( 'NONE', *, *, #16397, .T. ) ;
#31256=TOROIDAL_SURFACE ( 'NONE', #40007, 18.00000000000000000, 2.000000000000000000 ) ;
#31267=EDGE_CURVE ( 'NONE', #20890, #28792, #30646, .T. ) ;
#31268=CARTESIAN_POINT ( 'NONE',  ( 116.0829010812576882, -0.01829820670803256055, -12.14321520033834290 ) ) ;
#31269=CARTESIAN_POINT ( 'NONE',  ( 106.6626452545248611, 0.8980012041604421569, -11.00651665394454071 ) ) ;
#31270=CARTESIAN_POINT ( 'NONE',  ( 109.3018640045248304, 0.1403307496149616695, -15.46607636864997204 ) ) ;
#31271=CARTESIAN_POINT ( 'NONE',  ( 108.3295202545248657, -10.62599879583958717, -15.77991374673208469 ) ) ;
#31276=CARTESIAN_POINT ( 'NONE',  ( 112.7050671295247923, -10.62599879583958540, -13.39321520033831447 ) ) ;
#31282=CARTESIAN_POINT ( 'NONE',  ( 116.3860827545247787, -2.477300249445798297, -19.15521520033831138 ) ) ;
#31283=CARTESIAN_POINT ( 'NONE',  ( 116.0388171295248014, 0.1403307496149613920, -13.39321520033831447 ) ) ;
#31289=CARTESIAN_POINT ( 'NONE',  ( 114.7192077545248594, -7.250697342233347165, -7.631215200338321125 ) ) ;
#31290=CARTESIAN_POINT ( 'NONE',  ( 107.7738952545248310, -9.868328341294098749, -15.46607636864997204 ) ) ;
#31296=AXIS2_PLACEMENT_3D ( 'NONE', #15958, #40351, #19595 ) ;
#31302=CARTESIAN_POINT ( 'NONE',  ( 110.4825671295247815, 0.1403307496149613920, -13.39321520033831447 ) ) ;
#31311=CARTESIAN_POINT ( 'NONE',  ( 113.4690515045247992, -2.477300249445798297, -7.631215200338321125 ) ) ;
#31312=AXIS2_PLACEMENT_3D ( 'NONE', #29601, #43063, #18215 ) ;
#31317=VERTEX_POINT ( 'NONE', #27147 ) ;
#31318=CARTESIAN_POINT ( 'NONE',  ( 66.69189222814998175, -41.76310523276723785, -24.89321520033831447 ) ) ;
#31322=CARTESIAN_POINT ( 'NONE',  ( 85.06864399163163171, -29.49003633093008858, -10.37873928275900504 ) ) ;
#31323=LINE ( 'NONE', #34944, #11605 ) ;
#31325=EDGE_LOOP ( 'NONE', ( #16910, #6136, #19171, #14357 ) ) ;
#31329=CARTESIAN_POINT ( 'NONE',  ( 112.4967077545247633, -7.250697342233347165, -7.631215200338321125 ) ) ;
#31334=CARTESIAN_POINT ( 'NONE',  ( 111.1076452545248259, -9.868328341294098749, -15.46607636864997204 ) ) ;
#31336=CARTESIAN_POINT ( 'NONE',  ( 109.2292941585266703, -5.295636273138023320, -18.58536345472597517 ) ) ;
#31339=CARTESIAN_POINT ( 'NONE',  ( 106.1764733795248219, -8.938348069036489818, -17.46756447353520159 ) ) ;
#31340=CARTESIAN_POINT ( 'NONE',  ( 115.6220983795247861, -8.402594152722688392, -16.93181055722141792 ) ) ;
#31341=CARTESIAN_POINT ( 'NONE',  ( 108.3989733795248753, -8.938348069036489818, -17.46756447353520159 ) ) ;
#31355=( BOUNDED_SURFACE ( )  B_SPLINE_SURFACE ( 1, 2, ( 
 ( #35404, #755, #32218, #35175, #39068, #18775, #28817, #11710, #35855, #3953, #28360, #7838, #42274, #21292, #14906, #1432, #15353, #21744, #11037, #11492, #17875, #21518, #25397, #39294, #4629, #31771, #1215, #8063, #18550, #32442, #15129, #29036, #8288, #42945, #22190, #36086, #32664, #40197, #5745, #26290, #33553, #22863, #37204, #25836, #29260, #5524, #12391, #43171, #36756, #19444, #33327, #15802, #5976, #29936, #26064, #8964, #19902, #30162, #9189, #39968, #22637, #39743, #44081, #8730, #36535, #33787, #40653, #2101, #15576, #19665, #2331, #12161, #12845, #9408, #16028, #2558, #5309, #11940, #26746, #8511, #43850, #22415, #12619, #1875, #23095, #23318, #36308, #26520, #5076, #18993, #29481, #32881, #43617, #1655, #19225, #43394, #16261, #40429, #33105, #36977, #29704, #34891, #31053, #20800, #10104, #6451, #16487, #10538, #37895, #20135, #17165, #3465, #9876, #23786, #6674, #9639, #37675, #24440, #3239, #31271, #41563, #23561, #2790, #16940, #34021, #44310, #20581, #21017, #30387, #20359, #30610, #13517, #13065, #16717, #34245, #3018, #24226, #26964, #34680, #27426, #24008, #6890, #27649, #44528, #13958, #44982, #27869, #37442, #13291, #41347, #38116, #34460, #17382, #13740, #38331, #40885, #6214, #10323, #44758, #27199, #44 ),
 ( #41117, #41783, #7107, #30835, #28763, #486, #42222, #14174, #4574, #14399, #10983, #11655, #15074, #31938, #35119, #25344, #39238, #31717, #18499, #28986, #42446, #39468, #21466, #1158, #35577, #10763, #4124, #21691, #8002, #934, #21242, #22139, #42893, #265, #28541, #704, #28310, #28091, #42000, #35349, #7551, #24887, #3902, #24660, #21910, #25116, #32166, #25561, #8232, #31494, #3680, #4350, #18043, #35804, #7321, #14623, #11212, #38546, #39013, #17601, #42669, #17820, #38780, #18270, #7783, #14854, #11439, #32389, #43340, #32612, #40599, #29202, #36257, #5024, #18721, #30108, #1822, #9357, #40370, #2275, #43112, #36701, #18940, #9133, #8458, #19613, #36031, #36483, #5469, #5251, #11882, #1379, #23037, #16206, #22582, #33048, #1599, #43795, #12561, #19168, #32829, #4800, #8908, #15294, #26013, #25785, #36924, #44024, #12110, #39917, #43565, #39693, #29426, #19389, #5694, #22806, #22362, #33278, #15519, #33497, #8679, #12786, #26466, #15750, #29651, #12334, #26234, #40143, #2052, #26689, #15976, #29879, #2961, #6394, #34626, #6160, #13687, #9820, #13238, #2505, #33965, #17329, #37621, #3187, #10265, #44705, #20079, #27596, #3413, #20302, #27809, #41290, #30330, #41724, #41063, #6841, #31002, #34187, #9586, #44256, #17112 ) ),
 .UNSPECIFIED., .F., .F., .F. ) 
 B_SPLINE_SURFACE_WITH_KNOTS ( ( 2, 2 ),
 ( 3, 2, 2, 2, 2, 2, 2, 2, 2, 2, 2, 2, 2, 2, 2, 2, 2, 2, 2, 2, 2, 2, 2, 2, 2, 2, 2, 2, 2, 2, 2, 2, 2, 2, 2, 2, 2, 2, 2, 2, 2, 2, 2, 2, 2, 2, 2, 2, 2, 2, 2, 2, 2, 2, 2, 2, 2, 2, 2, 2, 2, 2, 2, 2, 2, 2, 2, 2, 2, 2, 2, 2, 2, 2, 2, 2, 2, 2, 2, 2, 3 ),
 ( 0.000000000000000000, 1.000000000000000000 ),
 ( 0.000000000000000000, 0.01250000000000000069, 0.02500000000000000139, 0.03749999999999999861, 0.05000000000000000278, 0.06250000000000000000, 0.07499999999999999722, 0.08749999999999999445, 0.1000000000000000056, 0.1125000000000000028, 0.1250000000000000000, 0.1375000000000000111, 0.1499999999999999944, 0.1625000000000000056, 0.1749999999999999889, 0.1875000000000000000, 0.2000000000000000111, 0.2124999999999999944, 0.2250000000000000056, 0.2374999999999999889, 0.2500000000000000000, 0.2625000000000000111, 0.2750000000000000222, 0.2874999999999999778, 0.2999999999999999889, 0.3125000000000000000, 0.3250000000000000111, 0.3375000000000000222, 0.3499999999999999778, 0.3624999999999999889, 0.3750000000000000000, 0.3875000000000000111, 0.4000000000000000222, 0.4124999999999999778, 0.4249999999999999889, 0.4375000000000000000, 0.4500000000000000111, 0.4625000000000000222, 0.4749999999999999778, 0.4874999999999999889, 0.5000000000000000000, 0.5124999999999999556, 0.5250000000000000222, 0.5374999999999999778, 0.5500000000000000444, 0.5625000000000000000, 0.5749999999999999556, 0.5875000000000000222, 0.5999999999999999778, 0.6125000000000000444, 0.6250000000000000000, 0.6374999999999999556, 0.6500000000000000222, 0.6624999999999999778, 0.6750000000000000444, 0.6875000000000000000, 0.6999999999999999556, 0.7125000000000000222, 0.7249999999999999778, 0.7375000000000000444, 0.7500000000000000000, 0.7624999999999999556, 0.7750000000000000222, 0.7874999999999999778, 0.8000000000000000444, 0.8125000000000000000, 0.8249999999999999556, 0.8375000000000000222, 0.8499999999999999778, 0.8625000000000000444, 0.8750000000000000000, 0.8874999999999999556, 0.9000000000000000222, 0.9124999999999999778, 0.9250000000000000444, 0.9375000000000000000, 0.9499999999999999556, 0.9625000000000000222, 0.9749999999999999778, 0.9875000000000000444, 1.000000000000000000 ),
 .UNSPECIFIED. ) 
 GEOMETRIC_REPRESENTATION_ITEM ( )  RATIONAL_B_SPLINE_SURFACE ( (
 ( 1.000000000000000000, 0.9238795325112869605, 1.000000000000000000, 0.9238795325112869605, 1.000000000000000000, 0.9238795325112869605, 1.000000000000000000, 0.9238795325112869605, 1.000000000000000000, 0.9238795325112869605, 1.000000000000000000, 0.9238795325112869605, 1.000000000000000000, 0.9238795325112869605, 1.000000000000000000, 0.9238795325112869605, 1.000000000000000000, 0.9238795325112869605, 1.000000000000000000, 0.9238795325112869605, 1.000000000000000000, 0.9238795325112869605, 1.000000000000000000, 0.9238795325112869605, 1.000000000000000000, 0.9238795325112869605, 1.000000000000000000, 0.9238795325112869605, 1.000000000000000000, 0.9238795325112869605, 1.000000000000000000, 0.9238795325112869605, 1.000000000000000000, 0.9238795325112869605, 1.000000000000000000, 0.9238795325112869605, 1.000000000000000000, 0.9238795325112869605, 1.000000000000000000, 0.9238795325112869605, 1.000000000000000000, 0.9238795325112869605, 1.000000000000000000, 0.9238795325112869605, 1.000000000000000000, 0.9238795325112869605, 1.000000000000000000, 0.9238795325112869605, 1.000000000000000000, 0.9238795325112869605, 1.000000000000000000, 0.9238795325112869605, 1.000000000000000000, 0.9238795325112869605, 1.000000000000000000, 0.9238795325112869605, 1.000000000000000000, 0.9238795325112869605, 1.000000000000000000, 0.9238795325112869605, 1.000000000000000000, 0.9238795325112869605, 1.000000000000000000, 0.9238795325112869605, 1.000000000000000000, 0.9238795325112869605, 1.000000000000000000, 0.9238795325112869605, 1.000000000000000000, 0.9238795325112869605, 1.000000000000000000, 0.9238795325112869605, 1.000000000000000000, 0.9238795325112869605, 1.000000000000000000, 0.9238795325112869605, 1.000000000000000000, 0.9238795325112869605, 1.000000000000000000, 0.9238795325112869605, 1.000000000000000000, 0.9238795325112869605, 1.000000000000000000, 0.9238795325112869605, 1.000000000000000000, 0.9238795325112869605, 1.000000000000000000, 0.9238795325112869605, 1.000000000000000000, 0.9238795325112869605, 1.000000000000000000, 0.9238795325112869605, 1.000000000000000000, 0.9238795325112869605, 1.000000000000000000, 0.9238795325112869605, 1.000000000000000000, 0.9238795325112869605, 1.000000000000000000, 0.9238795325112869605, 1.000000000000000000, 0.9238795325112869605, 1.000000000000000000, 0.9238795325112869605, 1.000000000000000000, 0.9238795325112869605, 1.000000000000000000, 0.9238795325112869605, 1.000000000000000000, 0.9238795325112869605, 1.000000000000000000, 0.9238795325112869605, 1.000000000000000000, 0.9238795325112869605, 1.000000000000000000, 0.9238795325112869605, 1.000000000000000000, 0.9238795325112869605, 1.000000000000000000, 0.9238795325112869605, 1.000000000000000000, 0.9238795325112869605, 1.000000000000000000, 0.9238795325112869605, 1.000000000000000000, 0.9238795325112869605, 1.000000000000000000, 0.9238795325112869605, 1.000000000000000000, 0.9238795325112869605, 1.000000000000000000, 0.9238795325112869605, 1.000000000000000000, 0.9238795325112869605, 1.000000000000000000, 0.9238795325112869605, 1.000000000000000000, 0.9238795325112869605, 1.000000000000000000, 0.9238795325112869605, 1.000000000000000000, 0.9238795325112869605, 1.000000000000000000, 0.9238795325112869605, 1.000000000000000000, 0.9238795325112869605, 1.000000000000000000, 0.9238795325112869605, 1.000000000000000000, 0.9238795325112869605, 1.000000000000000000, 0.9238795325112869605, 1.000000000000000000, 0.9238795325112869605, 1.000000000000000000, 0.9238795325112869605, 1.000000000000000000, 0.9238795325112869605, 1.000000000000000000, 0.9238795325112869605, 1.000000000000000000),
 ( 1.000000000000000000, 0.9238795325112869605, 1.000000000000000000, 0.9238795325112869605, 1.000000000000000000, 0.9238795325112869605, 1.000000000000000000, 0.9238795325112869605, 1.000000000000000000, 0.9238795325112869605, 1.000000000000000000, 0.9238795325112869605, 1.000000000000000000, 0.9238795325112869605, 1.000000000000000000, 0.9238795325112869605, 1.000000000000000000, 0.9238795325112869605, 1.000000000000000000, 0.9238795325112869605, 1.000000000000000000, 0.9238795325112869605, 1.000000000000000000, 0.9238795325112869605, 1.000000000000000000, 0.9238795325112869605, 1.000000000000000000, 0.9238795325112869605, 1.000000000000000000, 0.9238795325112869605, 1.000000000000000000, 0.9238795325112869605, 1.000000000000000000, 0.9238795325112869605, 1.000000000000000000, 0.9238795325112869605, 1.000000000000000000, 0.9238795325112869605, 1.000000000000000000, 0.9238795325112869605, 1.000000000000000000, 0.9238795325112869605, 1.000000000000000000, 0.9238795325112869605, 1.000000000000000000, 0.9238795325112869605, 1.000000000000000000, 0.9238795325112869605, 1.000000000000000000, 0.9238795325112869605, 1.000000000000000000, 0.9238795325112869605, 1.000000000000000000, 0.9238795325112869605, 1.000000000000000000, 0.9238795325112869605, 1.000000000000000000, 0.9238795325112869605, 1.000000000000000000, 0.9238795325112869605, 1.000000000000000000, 0.9238795325112869605, 1.000000000000000000, 0.9238795325112869605, 1.000000000000000000, 0.9238795325112869605, 1.000000000000000000, 0.9238795325112869605, 1.000000000000000000, 0.9238795325112869605, 1.000000000000000000, 0.9238795325112869605, 1.000000000000000000, 0.9238795325112869605, 1.000000000000000000, 0.9238795325112869605, 1.000000000000000000, 0.9238795325112869605, 1.000000000000000000, 0.9238795325112869605, 1.000000000000000000, 0.9238795325112869605, 1.000000000000000000, 0.9238795325112869605, 1.000000000000000000, 0.9238795325112869605, 1.000000000000000000, 0.9238795325112869605, 1.000000000000000000, 0.9238795325112869605, 1.000000000000000000, 0.9238795325112869605, 1.000000000000000000, 0.9238795325112869605, 1.000000000000000000, 0.9238795325112869605, 1.000000000000000000, 0.9238795325112869605, 1.000000000000000000, 0.9238795325112869605, 1.000000000000000000, 0.9238795325112869605, 1.000000000000000000, 0.9238795325112869605, 1.000000000000000000, 0.9238795325112869605, 1.000000000000000000, 0.9238795325112869605, 1.000000000000000000, 0.9238795325112869605, 1.000000000000000000, 0.9238795325112869605, 1.000000000000000000, 0.9238795325112869605, 1.000000000000000000, 0.9238795325112869605, 1.000000000000000000, 0.9238795325112869605, 1.000000000000000000, 0.9238795325112869605, 1.000000000000000000, 0.9238795325112869605, 1.000000000000000000, 0.9238795325112869605, 1.000000000000000000, 0.9238795325112869605, 1.000000000000000000, 0.9238795325112869605, 1.000000000000000000, 0.9238795325112869605, 1.000000000000000000, 0.9238795325112869605, 1.000000000000000000, 0.9238795325112869605, 1.000000000000000000, 0.9238795325112869605, 1.000000000000000000, 0.9238795325112869605, 1.000000000000000000, 0.9238795325112869605, 1.000000000000000000, 0.9238795325112869605, 1.000000000000000000, 0.9238795325112869605, 1.000000000000000000, 0.9238795325112869605, 1.000000000000000000, 0.9238795325112869605, 1.000000000000000000, 0.9238795325112869605, 1.000000000000000000, 0.9238795325112869605, 1.000000000000000000, 0.9238795325112869605, 1.000000000000000000, 0.9238795325112869605, 1.000000000000000000, 0.9238795325112869605, 1.000000000000000000, 0.9238795325112869605, 1.000000000000000000) ) ) 
 REPRESENTATION_ITEM ( '' )  SURFACE ( )  );
#31359=CARTESIAN_POINT ( 'NONE',  ( 114.6497546295247929, -4.863998795839590272, -7.631215200338315796 ) ) ;
#31360=ORIENTED_EDGE ( 'NONE', *, *, #33165, .F. ) ;
#31363=LINE ( 'NONE', #13825, #5518 ) ;
#31364=DIRECTION ( 'NONE',  ( 0.9970811988817434024, -0.07634843047859724008, 0.000000000000000000 ) ) ;
#31369=PLANE ( 'NONE',  #11297 ) ;
#31370=CARTESIAN_POINT ( 'NONE',  ( 113.0523327545247838, -6.936859964151250502, -8.388885654883777576 ) ) ;
#31380=CARTESIAN_POINT ( 'NONE',  ( 116.7333483795247844, -8.402594152722688392, -16.93181055722141792 ) ) ;
#31384=CARTESIAN_POINT ( 'NONE',  ( 114.9275671295247889, -10.62599879583958540, -13.39321520033831447 ) ) ;
#31388=CARTESIAN_POINT ( 'NONE',  ( 109.2294421309014751, -0.2315968891612809610, -10.77178248650439940 ) ) ;
#31390=CARTESIAN_POINT ( 'NONE',  ( 108.0517077545248696, -2.791137627527939813, -18.39754474579286025 ) ) ;
#31395=CARTESIAN_POINT ( 'NONE',  ( 108.9545983795247821, -0.7896495226426338832, -9.318865927141430916 ) ) ;
#31397=ORIENTED_EDGE ( 'NONE', *, *, #3335, .T. ) ;
#31407=CARTESIAN_POINT ( 'NONE',  ( 109.5796765045248122, -2.791137627527939813, -8.388885654883777576 ) ) ;
#31410=FACE_OUTER_BOUND ( 'NONE', #29463, .T. ) ;
#31411=ORIENTED_EDGE ( 'NONE', *, *, #3535, .F. ) ;
#31416=CARTESIAN_POINT ( 'NONE',  ( 107.5655358795247736, -8.402594152722688392, -9.854619843455216355 ) ) ;
#31417=VECTOR ( 'NONE', #42006, 1000.000000000000000 ) ;
#31435=CARTESIAN_POINT ( 'NONE',  ( 107.7044421295247929, 0.8980012041604618078, -13.39321520033831447 ) ) ;
#31437=CARTESIAN_POINT ( 'NONE',  ( 113.9552233795247815, -1.325403438956533675, -9.854619843455175499 ) ) ;
#31441=ORIENTED_EDGE ( 'NONE', *, *, #16225, .F. ) ;
#31447=CARTESIAN_POINT ( 'NONE',  ( 111.5243640045248412, 0.1403307496149616695, -15.46607636864997204 ) ) ;
#31450=VERTEX_POINT ( 'NONE', #31891 ) ;
#31455=CARTESIAN_POINT ( 'NONE',  ( 82.43378680891619581, -31.75787105231993479, -22.77522651806478748 ) ) ;
#31466=VERTEX_POINT ( 'NONE', #21413 ) ;
#31469=CARTESIAN_POINT ( 'NONE',  ( 107.9128015045248219, -2.477300249445798297, -7.631215200338321125 ) ) ;
#31486=EDGE_CURVE ( 'NONE', #21469, #24351, #29283, .T. ) ;
#31492=CARTESIAN_POINT ( 'NONE',  ( 113.5385046295247804, -4.863998795839590272, -18.39754474579285315 ) ) ;
#31493=CARTESIAN_POINT ( 'NONE',  ( 108.6073327545248048, -6.936859964151250502, -8.388885654883777576 ) ) ;
#31494=CARTESIAN_POINT ( 'NONE',  ( 112.6356140045247827, 0.1403307496149616695, -15.46607636864997204 ) ) ;
#31499=CARTESIAN_POINT ( 'NONE',  ( 112.4272546295247821, -4.863998795839590272, -7.631215200338315796 ) ) ;
#31505=CARTESIAN_POINT ( 'NONE',  ( 115.5526452545247622, 0.8980012041604421569, -11.00651665394454071 ) ) ;
#31506=CARTESIAN_POINT ( 'NONE',  ( 114.8581140045248361, 0.1403307496149616695, -15.46607636864997204 ) ) ;
#31510=AXIS2_PLACEMENT_3D ( 'NONE', #765, #14688, #7165 ) ;
#31512=CARTESIAN_POINT ( 'NONE',  ( 113.4690515045247992, -2.477300249445798297, -7.631215200338321125 ) ) ;
#31513=CARTESIAN_POINT ( 'NONE',  ( 107.7044421295247929, -9.868328341294093420, -13.39321520033831447 ) ) ;
#31523=VERTEX_POINT ( 'NONE', #3630 ) ;
#31526=CARTESIAN_POINT ( 'NONE',  ( 105.6208483795248299, -0.7896495226426338832, -9.318865927141430916 ) ) ;
#31527=CARTESIAN_POINT ( 'NONE',  ( 108.9545983795247821, -8.402594152722688392, -16.93181055722141792 ) ) ;
#31537=CARTESIAN_POINT ( 'NONE',  ( 114.9970202545248412, -10.62599879583958717, -15.77991374673208469 ) ) ;
#31543=ORIENTED_EDGE ( 'NONE', *, *, #45139, .T. ) ;
#31548=CARTESIAN_POINT ( 'NONE',  ( 85.85157537343363288, -26.34233955809028060, -8.371160363714436059 ) ) ;
#31554=CARTESIAN_POINT ( 'NONE',  ( 112.2883483795247770, -0.7896495226426338832, -9.318865927141430916 ) ) ;
#31559=CARTESIAN_POINT ( 'NONE',  ( 110.8298327545248299, -6.936859964151250502, -8.388885654883777576 ) ) ;
#31562=CARTESIAN_POINT ( 'NONE',  ( 109.2294420515965783, -4.107973114216393995, -18.49262090093784039 ) ) ;
#31564=CARTESIAN_POINT ( 'NONE',  ( 106.7320983795247855, -0.7896495226426338832, -9.318865927141430916 ) ) ;
#31565=CARTESIAN_POINT ( 'NONE',  ( 116.5944421295247793, -9.868328341294093420, -13.39321520033831447 ) ) ;
#31566=CARTESIAN_POINT ( 'NONE',  ( 109.5796765045248122, -7.250697342233347165, -19.15521520033831138 ) ) ;
#31584=DIRECTION ( 'NONE',  ( 0.000000000000000000, -1.000000000000000000, 0.000000000000000000 ) ) ;
#31585=CARTESIAN_POINT ( 'NONE',  ( 108.7462390045248242, 0.8980012041604421569, -15.77991374673208469 ) ) ;
#31586=FACE_OUTER_BOUND ( 'NONE', #41786, .T. ) ;
#31588=FACE_OUTER_BOUND ( 'NONE', #19049, .T. ) ;
#31595=CARTESIAN_POINT ( 'NONE',  ( 114.9275671295247889, 0.1403307496149613920, -13.39321520033831447 ) ) ;
#31598=( NAMED_UNIT ( * ) SI_UNIT ( $, .STERADIAN. ) SOLID_ANGLE_UNIT ( ) );
#31607=CARTESIAN_POINT ( 'NONE',  ( 115.5526452545247622, -9.868328341294098749, -15.46607636864997204 ) ) ;
#31611=CARTESIAN_POINT ( 'NONE',  ( 114.0941296295247867, -4.863998795839590272, -19.15521520033831493 ) ) ;
#31617=CARTESIAN_POINT ( 'NONE',  ( 109.5796765045248122, -2.791137627527939813, -8.388885654883777576 ) ) ;
#31618=CARTESIAN_POINT ( 'NONE',  ( 116.4579757138558023, 2.222835611391195343, -20.43720749888801080 ) ) ;
#31621=CARTESIAN_POINT ( 'NONE',  ( 110.4131140045248287, -10.62599879583958717, -11.00651665394454604 ) ) ;
#31632=CARTESIAN_POINT ( 'NONE',  ( 108.3989733795247759, -1.325403438956436419, -9.854619843455211026 ) ) ;
#31634=DIRECTION ( 'NONE',  ( 0.07634843047859296572, 0.9970811988817437355, 0.000000000000000000 ) ) ;
#31635=ORIENTED_EDGE ( 'NONE', *, *, #9691, .F. ) ;
#31640=CARTESIAN_POINT ( 'NONE',  ( 116.0388171295248014, -10.62599879583958540, -13.39321520033831447 ) ) ;
#31649=CIRCLE ( 'NONE', #26594, 0.5000000000000004441 ) ;
#31658=CARTESIAN_POINT ( 'NONE',  ( 114.3719421295247827, -9.868328341294093420, -13.39321520033831447 ) ) ;
#31668=CARTESIAN_POINT ( 'NONE',  ( 70.19189222814998175, -49.76310523276723785, -29.87698278062876511 ) ) ;
#31669=CARTESIAN_POINT ( 'NONE',  ( 113.8163171295247764, 0.1403307496149613920, -13.39321520033831447 ) ) ;
#31693=CARTESIAN_POINT ( 'NONE',  ( 107.7738952545248310, 0.8980012041604421569, -11.00651665394454071 ) ) ;
#31699=DIRECTION ( 'NONE',  ( 0.000000000000000000, 0.000000000000000000, -1.000000000000000000 ) ) ;
#31702=FACE_OUTER_BOUND ( 'NONE', #30690, .T. ) ;
#31708=CARTESIAN_POINT ( 'NONE',  ( 70.98136983621358809, -24.64626890834123785, -5.214987668974215396 ) ) ;
#31711=ORIENTED_EDGE ( 'NONE', *, *, #42676, .F. ) ;
#31712=CARTESIAN_POINT ( 'NONE',  ( 112.7050671295247923, -10.62599879583958540, -13.39321520033831980 ) ) ;
#31715=CARTESIAN_POINT ( 'NONE',  ( 114.0941296295247867, -4.863998795839590272, -8.388885654883775800 ) ) ;
#31716=CARTESIAN_POINT ( 'NONE',  ( 107.2182702545248105, 0.1403307496149616695, -11.32035403202665336 ) ) ;
#31717=CARTESIAN_POINT ( 'NONE',  ( 114.8581140045248361, 0.1403307496149616695, -15.46607636864997204 ) ) ;
#31722=CARTESIAN_POINT ( 'NONE',  ( 111.8716296295247901, -4.863998795839590272, -19.15521520033831493 ) ) ;
#31728=ADVANCED_FACE ( 'NONE', ( #40648 ), #26355, .F. ) ;
#31729=CARTESIAN_POINT ( 'NONE',  ( 116.1777233795247781, -8.938348069036489818, -17.46756447353520159 ) ) ;
#31730=CARTESIAN_POINT ( 'NONE',  ( 112.0105358795248804, -8.402594152722688392, -9.854619843455216355 ) ) ;
#31731=ORIENTED_EDGE ( 'NONE', *, *, #17584, .T. ) ;
#31736=CARTESIAN_POINT ( 'NONE',  ( 115.8304577545247582, -7.250697342233347165, -7.631215200338321125 ) ) ;
#31744=EDGE_CURVE ( 'NONE', #27865, #9168, #44076, .T. ) ;
#31751=DIRECTION ( 'NONE',  ( 0.2588190451025191297, -0.9659258262890686453, 0.000000000000000000 ) ) ;
#31752=CARTESIAN_POINT ( 'NONE',  ( 109.5796765045248122, -2.791137627527939813, -8.388885654883777576 ) ) ;
#31762=CARTESIAN_POINT ( 'NONE',  ( 112.6356140045247827, -10.62599879583958717, -11.00651665394454604 ) ) ;
#31769=CARTESIAN_POINT ( 'NONE',  ( 115.8304577545247582, -7.250697342233347165, -7.631215200338321125 ) ) ;
#31770=CARTESIAN_POINT ( 'NONE',  ( 84.86020291624818412, -29.99489077589588959, -11.86952202423883485 ) ) ;
#31771=CARTESIAN_POINT ( 'NONE',  ( 114.8581140045248361, -10.62599879583958717, -11.00651665394454604 ) ) ;
#31774=VERTEX_POINT ( 'NONE', #34017 ) ;
#31776=DIRECTION ( 'NONE',  ( 0.000000000000000000, 0.000000000000000000, -1.000000000000000000 ) ) ;
#31777=CARTESIAN_POINT ( 'NONE',  ( 113.4690515045247992, -2.477300249445798297, -7.631215200338321125 ) ) ;
#31782=CARTESIAN_POINT ( 'NONE',  ( 110.4825671295247815, 0.1403307496149613920, -13.39321520033831447 ) ) ;
#31786=CARTESIAN_POINT ( 'NONE',  ( 109.2294363213805610, -4.465500680915763354, -18.55270374900329600 ) ) ;
#31790=CARTESIAN_POINT ( 'NONE',  ( 107.9128015045248219, -2.477300249445798297, -7.631215200338321125 ) ) ;
#31796=ORIENTED_EDGE ( 'NONE', *, *, #23804, .F. ) ;
#31807=CARTESIAN_POINT ( 'NONE',  ( 109.3713171295247832, -10.62599879583958540, -13.39321520033831447 ) ) ;
#31811=DIRECTION ( 'NONE',  ( 6.830048575890719297E-16, 0.5905882410490338463, 0.8069730661766898461 ) ) ;
#31815=CARTESIAN_POINT ( 'NONE',  ( 111.1729021944299944, 0.6269505268395592079, -12.14321520033830026 ) ) ;
#31816=CARTESIAN_POINT ( 'NONE',  ( 112.2358197905468984, 0.6938714319018670640, -12.14321520033833579 ) ) ;
#31817=CARTESIAN_POINT ( 'NONE',  ( 116.1777233795247781, -1.325403438956436419, -9.854619843455211026 ) ) ;
#31829=CARTESIAN_POINT ( 'NONE',  ( 73.47343079648352671, -1.934511955536642791, -14.64321520033831447 ) ) ;
#31831=CARTESIAN_POINT ( 'NONE',  ( 115.8999108795247821, -1.325403438956436419, -16.93181055722141792 ) ) ;
#31836=CARTESIAN_POINT ( 'NONE',  ( 111.0381921295247878, 0.8980012041604618078, -13.39321520033831447 ) ) ;
#31840=CARTESIAN_POINT ( 'NONE',  ( 109.2295198960366776, -5.481997562533197588, -7.823790098599812559 ) ) ;
#31842=CARTESIAN_POINT ( 'NONE',  ( 116.5249890045247980, 0.8980012041604421569, -15.77991374673208469 ) ) ;
#31846=CARTESIAN_POINT ( 'NONE',  ( 111.5938171295247940, -10.62599879583958540, -13.39321520033831447 ) ) ;
#31857=CARTESIAN_POINT ( 'NONE',  ( 113.1912390045248031, 0.8980012041604421569, -15.77991374673208469 ) ) ;
#31859=LINE ( 'NONE', #28456, #44691 ) ;
#31865=ORIENTED_EDGE ( 'NONE', *, *, #5509, .F. ) ;
#31866=CARTESIAN_POINT ( 'NONE',  ( 116.5249890045247980, 0.8980012041604421569, -15.77991374673208469 ) ) ;
#31881=DIRECTION ( 'NONE',  ( -1.000000000000000000, 0.000000000000000000, 0.000000000000000000 ) ) ;
#31883=ORIENTED_EDGE ( 'NONE', *, *, #20391, .F. ) ;
#31885=CARTESIAN_POINT ( 'NONE',  ( 115.5526452545247622, -9.868328341294098749, -15.46607636864997204 ) ) ;
#31890=ORIENTED_EDGE ( 'NONE', *, *, #25861, .T. ) ;
#31891=CARTESIAN_POINT ( 'NONE',  ( 66.06194382436763135, -14.97931106434683635, -4.893215200338314474 ) ) ;
#31895=CARTESIAN_POINT ( 'NONE',  ( 76.19189222814999596, -49.76310523276725206, -36.33917278160905084 ) ) ;
#31896=CARTESIAN_POINT ( 'NONE',  ( 112.9828796295247884, -4.863998795839590272, -8.388885654883775800 ) ) ;
#31902=EDGE_CURVE ( 'NONE', #40888, #424, #7940, .T. ) ;
#31903=AXIS2_PLACEMENT_3D ( 'NONE', #24389, #428, #24610 ) ;
#31910=CARTESIAN_POINT ( 'NONE',  ( 114.3024890045248156, -9.868328341294098749, -11.32035403202665869 ) ) ;
#31916=CARTESIAN_POINT ( 'NONE',  ( 110.6214733795247867, -1.325403438956533675, -9.854619843455175499 ) ) ;
#31922=CARTESIAN_POINT ( 'NONE',  ( 79.62450370917392206, 5.105616368456423082, -20.14282611309224436 ) ) ;
#31925=CYLINDRICAL_SURFACE ( 'NONE', #18218, 5.000000000000004441 ) ;
#31931=CARTESIAN_POINT ( 'NONE',  ( 115.5212212410415873, 0.7607806665037644134, -12.14321520033829493 ) ) ;
#31933=VERTEX_POINT ( 'NONE', #17981 ) ;
#31934=CARTESIAN_POINT ( 'NONE',  ( 111.8752889883689932, 0.3193521225029610777, -12.14321520033831625 ) ) ;
#31935=CARTESIAN_POINT ( 'NONE',  ( 116.1082702545247827, -10.62599879583958717, -15.77991374673208469 ) ) ;
#31936=CARTESIAN_POINT ( 'NONE',  ( 114.9970202545248412, 0.1403307496149616695, -11.32035403202665336 ) ) ;
#31937=CARTESIAN_POINT ( 'NONE',  ( 109.2324108795247923, -1.325403438956436419, -16.93181055722141792 ) ) ;
#31938=CARTESIAN_POINT ( 'NONE',  ( 115.1359265045248605, -2.791137627527939813, -8.388885654883777576 ) ) ;
#31943=CARTESIAN_POINT ( 'NONE',  ( 107.2182702545248105, -10.62599879583958717, -15.77991374673208469 ) ) ;
#31949=CARTESIAN_POINT ( 'NONE',  ( 116.2471765045247594, -7.250697342233347165, -19.15521520033831138 ) ) ;
#31950=CARTESIAN_POINT ( 'NONE',  ( 111.2465515045248168, -6.936859964151250502, -18.39754474579286025 ) ) ;
#31951=ORIENTED_EDGE ( 'NONE', *, *, #15843, .T. ) ;
#31960=EDGE_CURVE ( 'NONE', #14735, #41199, #20539, .T. ) ;
#31963=DIRECTION ( 'NONE',  ( -1.000000000000000000, 0.000000000000000000, 0.000000000000000000 ) ) ;
#31969=CARTESIAN_POINT ( 'NONE',  ( 106.8710046295248759, -4.863998795839590272, -7.631215200338315796 ) ) ;
#31971=CARTESIAN_POINT ( 'NONE',  ( 111.0381921295247878, -9.868328341294093420, -13.39321520033831447 ) ) ;
#31981=CARTESIAN_POINT ( 'NONE',  ( 111.5243640045248412, -10.62599879583958717, -11.00651665394454604 ) ) ;
#31982=CARTESIAN_POINT ( 'NONE',  ( 117.1329525761119186, -11.25461401719748977, -21.76703976714820143 ) ) ;
#31991=CARTESIAN_POINT ( 'NONE',  ( 116.3860827545247787, -2.477300249445798297, -19.15521520033831138 ) ) ;
#31997=DIRECTION ( 'NONE',  ( 0.000000000000000000, 0.000000000000000000, 1.000000000000000000 ) ) ;
#31998=CARTESIAN_POINT ( 'NONE',  ( 110.8992858795247827, -0.7896495226426338832, -17.46756447353520159 ) ) ;
#32002=FACE_OUTER_BOUND ( 'NONE', #34996, .T. ) ;
#32003=CARTESIAN_POINT ( 'NONE',  ( 109.0240515045248202, -6.936859964151250502, -18.39754474579286025 ) ) ;
#32006=CARTESIAN_POINT ( 'NONE',  ( 109.2294421271526943, -7.422887316267482660, -18.05243104752941719 ) ) ;
#32009=CARTESIAN_POINT ( 'NONE',  ( 116.5249890045247980, -9.868328341294098749, -11.32035403202665869 ) ) ;
#32010=CARTESIAN_POINT ( 'NONE',  ( 114.3024890045248156, -9.868328341294098749, -11.32035403202665869 ) ) ;
#32023=VERTEX_POINT ( 'NONE', #646 ) ;
#32027=FACE_OUTER_BOUND ( 'NONE', #32069, .T. ) ;
#32028=CARTESIAN_POINT ( 'NONE',  ( 111.0381921295247878, 0.8980012041604618078, -13.39321520033831447 ) ) ;
#32030=DIRECTION ( 'NONE',  ( -0.9970811988817434024, 0.07634843047859724008, 9.125038414728753042E-18 ) ) ;
#32031=CARTESIAN_POINT ( 'NONE',  ( 116.8689275254964883, 0.3188565254943556693, -14.64321520033831447 ) ) ;
#32032=CARTESIAN_POINT ( 'NONE',  ( 113.1217858795247935, -8.402594152722688392, -9.854619843455216355 ) ) ;
#32037=DIRECTION ( 'NONE',  ( -1.000000000000000000, 0.000000000000000000, 0.000000000000000000 ) ) ;
#32040=CARTESIAN_POINT ( 'NONE',  ( 112.9134265045247645, -2.791137627527939813, -8.388885654883777576 ) ) ;
#32043=CARTESIAN_POINT ( 'NONE',  ( 69.69189222814998175, -41.76310523276723785, -20.39321520033831447 ) ) ;
#32050=ADVANCED_FACE ( 'NONE', ( #38946 ), #25505, .T. ) ;
#32052=CARTESIAN_POINT ( 'NONE',  ( 112.4272546295247821, -4.863998795839590272, -18.39754474579285315 ) ) ;
#32055=CARTESIAN_POINT ( 'NONE',  ( 85.90931634775512293, -27.45388746120685397, -8.668790192341086609 ) ) ;
#32056=CARTESIAN_POINT ( 'NONE',  ( 114.3719421295247827, 0.8980012041604618078, -13.39321520033831447 ) ) ;
#32059=CARTESIAN_POINT ( 'NONE',  ( 116.5249890045247980, -9.868328341294102302, -11.32035403202661428 ) ) ;
#32061=CARTESIAN_POINT ( 'NONE',  ( 109.2294456423300915, -1.194640643069894370, -9.436217729478444838 ) ) ;
#32063=CARTESIAN_POINT ( 'NONE',  ( 115.2053796295247849, -4.863998795839590272, -19.15521520033831493 ) ) ;
#32064=DIRECTION ( 'NONE',  ( 1.000000000000000000, 0.000000000000000000, 0.000000000000000000 ) ) ;
#32067=CARTESIAN_POINT ( 'NONE',  ( 112.2188952545247531, 0.8980012041604421569, -11.00651665394454071 ) ) ;
#32069=EDGE_LOOP ( 'NONE', ( #23098, #40398, #42130, #36396 ) ) ;
#32074=TOROIDAL_SURFACE ( 'NONE', #12431, 10.00000000000000000, 2.000000000000000000 ) ;
#32077=CARTESIAN_POINT ( 'NONE',  ( 112.0105358795247810, -0.7896495226426338832, -17.46756447353520159 ) ) ;
#32081=VERTEX_POINT ( 'NONE', #32104 ) ;
#32090=DIRECTION ( 'NONE',  ( -1.000000000000000000, 0.000000000000000000, 0.000000000000000000 ) ) ;
#32091=CARTESIAN_POINT ( 'NONE',  ( 64.22825944749166638, -35.92680753996140197, -5.785566283887345840 ) ) ;
#32097=EDGE_CURVE ( 'NONE', #21089, #31317, #21851, .T. ) ;
#32104=CARTESIAN_POINT ( 'NONE',  ( 83.49267580666517574, -32.76310523276723785, -23.89321520033831803 ) ) ;
#32108=CARTESIAN_POINT ( 'NONE',  ( 111.6632702545248605, 0.1403307496149616695, -11.32035403202665336 ) ) ;
#32119=CARTESIAN_POINT ( 'NONE',  ( 113.6774108795247997, -1.325403438956436419, -16.93181055722141792 ) ) ;
#32130=CARTESIAN_POINT ( 'NONE',  ( 63.27883505452616930, -30.76310523276723785, -21.89321520033831447 ) ) ;
#32131=CARTESIAN_POINT ( 'NONE',  ( 110.2548541094426895, 0.3591747506842615789, -12.14321520033831625 ) ) ;
#32134=CARTESIAN_POINT ( 'NONE',  ( 117.0111608795247946, -1.325403438956436419, -16.93181055722141792 ) ) ;
#32144=VERTEX_POINT ( 'NONE', #21403 ) ;
#32147=CARTESIAN_POINT ( 'NONE',  ( 112.1114130180079798, 0.7607806665037644134, -14.64321520033833046 ) ) ;
#32151=CIRCLE ( 'NONE', #12523, 2.000000000000001776 ) ;
#32152=EDGE_CURVE ( 'NONE', #6107, #35524, #15014, .T. ) ;
#32162=CARTESIAN_POINT ( 'NONE',  ( 111.7802383310706773, 0.1843591316377651834, -12.14321520033831625 ) ) ;
#32163=CARTESIAN_POINT ( 'NONE',  ( 114.9970202545248412, -10.62599879583958717, -15.77991374673208469 ) ) ;
#32164=CARTESIAN_POINT ( 'NONE',  ( 113.3995983795247895, -8.402594152722688392, -16.93181055722141792 ) ) ;
#32166=CARTESIAN_POINT ( 'NONE',  ( 112.8439733795247832, -1.325403438956436419, -9.854619843455211026 ) ) ;
#32169=EDGE_LOOP ( 'NONE', ( #44782, #29038 ) ) ;
#32171=CARTESIAN_POINT ( 'NONE',  ( 105.6903015045248253, -2.477300249445798297, -7.631215200338321125 ) ) ;
#32178=CARTESIAN_POINT ( 'NONE',  ( 110.6214733795247867, -1.325403438956436419, -9.854619843455211026 ) ) ;
#32194=CARTESIAN_POINT ( 'NONE',  ( 106.3153796295248412, -4.863998795839590272, -8.388885654883775800 ) ) ;
#32207=CARTESIAN_POINT ( 'NONE',  ( 109.6491296295247793, -4.863998795839590272, -19.15521520033831493 ) ) ;
#32208=CARTESIAN_POINT ( 'NONE',  ( 61.69189222814998175, -69.76310523276724496, -16.89321520033831447 ) ) ;
#32211=CARTESIAN_POINT ( 'NONE',  ( 61.69189222814998175, -80.85404093559408523, -31.07034979220001603 ) ) ;
#32212=ORIENTED_EDGE ( 'NONE', *, *, #27452, .F. ) ;
#32215=CARTESIAN_POINT ( 'NONE',  ( 116.1777233795247781, -8.938348069036489818, -17.46756447353520159 ) ) ;
#32217=FACE_OUTER_BOUND ( 'NONE', #30299, .T. ) ;
#32218=CARTESIAN_POINT ( 'NONE',  ( 116.4555358795247884, -0.7896495226426338832, -17.46756447353520159 ) ) ;
#32222=DIRECTION ( 'NONE',  ( 0.3445294493088594256, 0.9387755102040817867, 0.000000000000000000 ) ) ;
#32223=CARTESIAN_POINT ( 'NONE',  ( 112.6356140045247827, -10.62599879583958717, -11.00651665394454604 ) ) ;
#32229=LINE ( 'NONE', #1001, #4437 ) ;
#32230=EDGE_LOOP ( 'NONE', ( #25393, #32465 ) ) ;
#32232=CARTESIAN_POINT ( 'NONE',  ( 116.1082702545247827, -10.62599879583958540, -15.77991374673208469 ) ) ;
#32233=CARTESIAN_POINT ( 'NONE',  ( 109.2295226117709603, -5.526696438288506208, -18.58224487948997350 ) ) ;
#32237=CARTESIAN_POINT ( 'NONE',  ( 113.9552233795247815, -1.325403438956436419, -9.854619843455211026 ) ) ;
#32255=CARTESIAN_POINT ( 'NONE',  ( 110.2047546295247855, -4.863998795839590272, -7.631215200338315796 ) ) ;
#32256=DIRECTION ( 'NONE',  ( 0.000000000000000000, -1.000000000000000000, -1.195183497228115774E-16 ) ) ;
#32257=CARTESIAN_POINT ( 'NONE',  ( 116.7329504682427768, 0.5115630086001619059, -14.64321520033831447 ) ) ;
#32258=CARTESIAN_POINT ( 'NONE',  ( 111.6632702545248605, 0.1403307496149616695, -11.32035403202665336 ) ) ;
#32265=CARTESIAN_POINT ( 'NONE',  ( 108.9545983795247821, -8.402594152722688392, -16.93181055722141792 ) ) ;
#32268=ADVANCED_FACE ( 'NONE', ( #19104 ), #29441, .T. ) ;
#32277=CARTESIAN_POINT ( 'NONE',  ( 113.1217858795247935, -8.402594152722688392, -9.854619843455216355 ) ) ;
#32285=CARTESIAN_POINT ( 'NONE',  ( 107.7044421295247929, 0.8980012041604618078, -13.39321520033831447 ) ) ;
#32287=CIRCLE ( 'NONE', #18472, 4.999999999999999112 ) ;
#32289=CARTESIAN_POINT ( 'NONE',  ( 115.9473434012278830, 0.04929351793716424401, -14.64321520033828961 ) ) ;
#32290=CARTESIAN_POINT ( 'NONE',  ( 109.2294483239461016, -0.3417072992519313845, -10.56426903870459810 ) ) ;
#32292=CARTESIAN_POINT ( 'NONE',  ( 106.7320983795247855, -8.402594152722688392, -16.93181055722141792 ) ) ;
#32293=CARTESIAN_POINT ( 'NONE',  ( 117.1067020526858897, 1.586544940016389571, -21.37821035455269936 ) ) ;
#32294=CARTESIAN_POINT ( 'NONE',  ( 83.47365629695968892, -32.82170496130314064, -21.84607615589008489 ) ) ;
#32297=CARTESIAN_POINT ( 'NONE',  ( 111.2465515045248168, -2.477300249445798297, -7.631215200338321125 ) ) ;
#32299=EDGE_LOOP ( 'NONE', ( #4176, #41956, #17192, #25635 ) ) ;
#32309=CARTESIAN_POINT ( 'NONE',  ( 115.8304577545247582, -7.250697342233347165, -7.631215200338321125 ) ) ;
#32313=ORIENTED_EDGE ( 'NONE', *, *, #6940, .T. ) ;
#32322=CARTESIAN_POINT ( 'NONE',  ( 77.43858880758799046, -56.71620948281238839, -1.734724326163099350 ) ) ;
#32336=CARTESIAN_POINT ( 'NONE',  ( 111.5243640045248412, 0.1403307496149616695, -15.46607636864997204 ) ) ;
#32345=EDGE_CURVE ( 'NONE', #25696, #4599, #4127, .T. ) ;
#32348=CARTESIAN_POINT ( 'NONE',  ( 107.6349890045248401, -9.868328341294098749, -11.32035403202665869 ) ) ;
#32360=CARTESIAN_POINT ( 'NONE',  ( 115.8999108795247821, -1.325403438956436419, -16.93181055722141792 ) ) ;
#32370=ORIENTED_EDGE ( 'NONE', *, *, #8425, .F. ) ;
#32372=DIRECTION ( 'NONE',  ( 0.9999995469159186356, 0.0009519285464175526951, 0.000000000000000000 ) ) ;
#32373=CARTESIAN_POINT ( 'NONE',  ( 79.49708691561605178, 5.079251341110372131, -20.33566263698374144 ) ) ;
#32381=CARTESIAN_POINT ( 'NONE',  ( 116.6774435224926094, -8.419877142191296571, -17.02538347942430619 ) ) ;
#32387=CARTESIAN_POINT ( 'NONE',  ( 116.5944421295247793, 0.8980012041604618078, -13.39321520033831447 ) ) ;
#32388=CARTESIAN_POINT ( 'NONE',  ( 115.9693640045247776, 0.1403307496149616695, -15.46607636864997204 ) ) ;
#32389=CARTESIAN_POINT ( 'NONE',  ( 111.3854577545248645, -2.791137627527939813, -18.39754474579286025 ) ) ;
#32394=CARTESIAN_POINT ( 'NONE',  ( 108.2600671295247992, -10.62599879583958540, -13.39321520033831447 ) ) ;
#32398=PLANE ( 'NONE',  #21386 ) ;
#32400=CARTESIAN_POINT ( 'NONE',  ( 112.4967077545247633, -7.250697342233347165, -7.631215200338321125 ) ) ;
#32401=CARTESIAN_POINT ( 'NONE',  ( 110.9687390045248350, -9.868328341294098749, -11.32035403202665869 ) ) ;
#32407=CYLINDRICAL_SURFACE ( 'NONE', #43074, 3.000000000000001332 ) ;
#32420=CARTESIAN_POINT ( 'NONE',  ( 115.4831921295247952, 0.8980012041604618078, -13.39321520033831447 ) ) ;
#32422=VERTEX_POINT ( 'NONE', #4325 ) ;
#32428=ORIENTED_EDGE ( 'NONE', *, *, #39772, .F. ) ;
#32430=CARTESIAN_POINT ( 'NONE',  ( 61.99939684703689124, -65.50319228955336825, -44.43454011388369906 ) ) ;
#32431=CARTESIAN_POINT ( 'NONE',  ( 110.7603796295247918, -4.863998795839590272, -19.15521520033831493 ) ) ;
#32436=LINE ( 'NONE', #32211, #37841 ) ;
#32442=CARTESIAN_POINT ( 'NONE',  ( 114.5803015045248117, -2.477300249445798297, -7.631215200338321125 ) ) ;
#32447=CARTESIAN_POINT ( 'NONE',  ( 106.5931921295248372, 0.8980012041604618078, -13.39321520033831447 ) ) ;
#32452=CARTESIAN_POINT ( 'NONE',  ( 105.5513952545248060, -9.868328341294098749, -15.46607636864997204 ) ) ;
#32453=ORIENTED_EDGE ( 'NONE', *, *, #28576, .T. ) ;
#32454=CARTESIAN_POINT ( 'NONE',  ( 116.5043621053768703, 0.3967854368539331933, -16.28112951403851838 ) ) ;
#32455=CARTESIAN_POINT ( 'NONE',  ( 109.2295493080124231, -10.35223054996752623, -12.16705481747161599 ) ) ;
#32458=CARTESIAN_POINT ( 'NONE',  ( 112.6356140045247827, 0.1403307496149616695, -15.46607636864997204 ) ) ;
#32459=CARTESIAN_POINT ( 'NONE',  ( 113.6079577545248043, -2.791137627527939813, -18.39754474579286025 ) ) ;
#32465=ORIENTED_EDGE ( 'NONE', *, *, #26305, .T. ) ;
#32477=DIRECTION ( 'NONE',  ( 0.000000000000000000, 0.000000000000000000, 1.000000000000000000 ) ) ;
#32478=CARTESIAN_POINT ( 'NONE',  ( 115.6915515045247531, -6.936859964151250502, -18.39754474579286025 ) ) ;
#32480=AXIS2_PLACEMENT_3D ( 'NONE', #33567, #19236, #19005 ) ;
#32486=CARTESIAN_POINT ( 'NONE',  ( 111.5243640045248412, 0.1403307496149616695, -15.46607636864997204 ) ) ;
#32488=DIRECTION ( 'NONE',  ( 0.7071067811865520136, 0.000000000000000000, -0.7071067811865431318 ) ) ;
#32497=CARTESIAN_POINT ( 'NONE',  ( 116.6638952545248031, -9.868328341294098749, -15.46607636864997204 ) ) ;
#32502=CARTESIAN_POINT ( 'NONE',  ( 85.78840348512180469, -27.74674259770401719, -8.784702801739287636 ) ) ;
#32503=CARTESIAN_POINT ( 'NONE',  ( 109.7185827545247889, -2.477300249445798297, -19.15521520033831138 ) ) ;
#32506=FACE_OUTER_BOUND ( 'NONE', #1130, .T. ) ;
#32509=CARTESIAN_POINT ( 'NONE',  ( 114.3719421295247827, 0.8980012041604618078, -13.39321520033831447 ) ) ;
#32510=CARTESIAN_POINT ( 'NONE',  ( 117.2294421295247844, 1.035107641088057973, -4.893215200338314474 ) ) ;
#32511=CARTESIAN_POINT ( 'NONE',  ( 82.44760263944102974, -31.73904833139433279, -23.17969760592469441 ) ) ;
#32516=CARTESIAN_POINT ( 'NONE',  ( 73.53114257624162065, -54.10809544429395856, -7.393215200338315363 ) ) ;
#32526=CARTESIAN_POINT ( 'NONE',  ( 114.3024890045248156, 0.8980012041604421569, -15.77991374673208469 ) ) ;
#32528=CARTESIAN_POINT ( 'NONE',  ( 116.7904600221807669, -3.161398967842792285, -18.30238421764784462 ) ) ;
#32554=EDGE_CURVE ( 'NONE', #9687, #574, #23243, .T. ) ;
#32559=CARTESIAN_POINT ( 'NONE',  ( 112.6356140045247827, 0.1403307496149616695, -15.46607636864997204 ) ) ;
#32569=CARTESIAN_POINT ( 'NONE',  ( 61.43583762032555029, 4.505738898882963639, -12.14321520033831625 ) ) ;
#32570=CARTESIAN_POINT ( 'NONE',  ( 108.8851452545248151, -9.868328341294098749, -15.46607636864997204 ) ) ;
#32575=CARTESIAN_POINT ( 'NONE',  ( 79.05243529145373316, 4.793396140045460108, -4.893215200338314474 ) ) ;
#32579=VERTEX_POINT ( 'NONE', #16634 ) ;
#32580=CARTESIAN_POINT ( 'NONE',  ( 114.8581140045248361, 0.1403307496149616695, -15.46607636864997204 ) ) ;
#32585=DIRECTION ( 'NONE',  ( 1.000000000000000000, -1.084202172485504040E-15, 0.000000000000000000 ) ) ;
#32587=CARTESIAN_POINT ( 'NONE',  ( 111.5006797178593700, -0.3595008806742178709, -15.96590799893915857 ) ) ;
#32590=EDGE_LOOP ( 'NONE', ( #6429, #31252, #10204, #12062 ) ) ;
#32593=DIRECTION ( 'NONE',  ( 0.000000000000000000, 0.000000000000000000, 1.000000000000000000 ) ) ;
#32594=CARTESIAN_POINT ( 'NONE',  ( 115.2518531537514832, 0.4930828106259610433, -14.64321520033831447 ) ) ;
#32607=ADVANCED_FACE ( 'NONE', ( #1798, #26209 ), #5446, .F. ) ;
#32608=ORIENTED_EDGE ( 'NONE', *, *, #42087, .F. ) ;
#32610=DIRECTION ( 'NONE',  ( 0.000000000000000000, -0.9284778069183718952, -0.3713878862591650232 ) ) ;
#32611=CARTESIAN_POINT ( 'NONE',  ( 110.5520202545248054, 0.1403307496149616695, -11.32035403202665336 ) ) ;
#32612=CARTESIAN_POINT ( 'NONE',  ( 111.2465515045248168, -6.936859964151250502, -18.39754474579286025 ) ) ;
#32618=CARTESIAN_POINT ( 'NONE',  ( 108.3295202545248657, -10.62599879583958717, -15.77991374673208469 ) ) ;
#32619=LINE ( 'NONE', #21917, #10321 ) ;
#32620=EDGE_CURVE ( 'NONE', #12113, #11479, #2027, .T. ) ;
#32623=CARTESIAN_POINT ( 'NONE',  ( 113.8604010812576774, -0.01829820670803256055, -12.14321520033831625 ) ) ;
#32625=CARTESIAN_POINT ( 'NONE',  ( 109.1629577545248395, -7.250697342233347165, -7.631215200338321125 ) ) ;
#32626=CARTESIAN_POINT ( 'NONE',  ( 113.2606921295247702, -9.868328341294093420, -13.39321520033831447 ) ) ;
#32628=DIRECTION ( 'NONE',  ( 0.000000000000000000, 0.000000000000000000, -1.000000000000000000 ) ) ;
#32637=CARTESIAN_POINT ( 'NONE',  ( 113.6773954522301864, 0.1168444861213632779, -14.64321520033831447 ) ) ;
#32641=CARTESIAN_POINT ( 'NONE',  ( 106.6626452545248611, -9.868328341294098749, -15.46607636864997204 ) ) ;
#32652=CARTESIAN_POINT ( 'NONE',  ( 61.79265099467970401, -65.87623890127542836, -43.58359585756122101 ) ) ;
#32653=CARTESIAN_POINT ( 'NONE',  ( 112.2883483795247770, -0.7896495226426338832, -9.318865927141430916 ) ) ;
#32662=CARTESIAN_POINT ( 'NONE',  ( 111.5938171295247940, -10.62599879583958540, -13.39321520033831447 ) ) ;
#32663=CARTESIAN_POINT ( 'NONE',  ( 116.4555358795247884, -8.402594152722688392, -9.854619843455216355 ) ) ;
#32664=CARTESIAN_POINT ( 'NONE',  ( 114.0941296295247867, -4.863998795839590272, -19.15521520033831493 ) ) ;
#32670=CARTESIAN_POINT ( 'NONE',  ( 106.3153796295248412, -4.863998795839590272, -19.15521520033831493 ) ) ;
#32674=CARTESIAN_POINT ( 'NONE',  ( 117.0832711243935051, -11.36631965120432319, -5.665662734129918832 ) ) ;
#32675=CARTESIAN_POINT ( 'NONE',  ( 107.2877233795247776, -1.325403438956436419, -9.854619843455211026 ) ) ;
#32676=ORIENTED_EDGE ( 'NONE', *, *, #1678, .F. ) ;
#32677=CARTESIAN_POINT ( 'NONE',  ( 116.3860827545247787, -2.477300249445798297, -19.15521520033830427 ) ) ;
#32678=CARTESIAN_POINT ( 'NONE',  ( 109.2294433879109761, -10.43664627197690642, -13.07502879523307016 ) ) ;
#32680=CARTESIAN_POINT ( 'NONE',  ( 112.7745202545247878, 0.1403307496149616695, -11.32035403202665336 ) ) ;
#32681=CARTESIAN_POINT ( 'NONE',  ( 114.9275671295247889, 0.1403307496149613920, -13.39321520033831447 ) ) ;
#32699=CARTESIAN_POINT ( 'NONE',  ( 112.4272546295247821, -4.863998795839590272, -18.39754474579285315 ) ) ;
#32705=PLANE ( 'NONE',  #21397 ) ;
#32706=CARTESIAN_POINT ( 'NONE',  ( 110.8992858795247827, -8.402594152722688392, -9.854619843455216355 ) ) ;
#32717=CARTESIAN_POINT ( 'NONE',  ( 109.4407702545248355, 0.1403307496149616695, -11.32035403202665336 ) ) ;
#32722=CARTESIAN_POINT ( 'NONE',  ( 108.5378796295247810, -4.863998795839590272, -19.15521520033831493 ) ) ;
#32725=LINE ( 'NONE', #22256, #23838 ) ;
#32728=CARTESIAN_POINT ( 'NONE',  ( 116.1082702545247827, -10.62599879583958717, -15.77991374673208469 ) ) ;
#32730=CARTESIAN_POINT ( 'NONE',  ( 83.38637814964508266, -33.05952087933068384, -23.46618001151087540 ) ) ;
#32733=CARTESIAN_POINT ( 'NONE',  ( 107.6349890045248401, 0.8980012041604421569, -15.77991374673208469 ) ) ;
#32741=PRODUCT_CONTEXT ( 'NONE', #37879, 'mechanical' ) ;
#32744=CARTESIAN_POINT ( 'NONE',  ( 114.9275671295247889, -10.62599879583958540, -13.39321520033831447 ) ) ;
#32753=CARTESIAN_POINT ( 'NONE',  ( 77.77634386988368931, 3.254514819260763581, -4.893215200338314474 ) ) ;
#32768=CARTESIAN_POINT ( 'NONE',  ( 114.2330358795247776, -8.402594152722688392, -9.854619843455216355 ) ) ;
#32772=CARTESIAN_POINT ( 'NONE',  ( 115.4831921295247952, 0.8980012041604618078, -13.39321520033831447 ) ) ;
#32773=CARTESIAN_POINT ( 'NONE',  ( 110.8298327545248299, -6.936859964151250502, -8.388885654883777576 ) ) ;
#32776=CIRCLE ( 'NONE', #37876, 2.999999999999998224 ) ;
#32778=FACE_OUTER_BOUND ( 'NONE', #2508, .T. ) ;
#32780=AXIS2_PLACEMENT_3D ( 'NONE', #27965, #21103, #20677 ) ;
#32786=CARTESIAN_POINT ( 'NONE',  ( 105.5513952545248060, -9.868328341294098749, -15.46607636864997204 ) ) ;
#32787=ORIENTED_EDGE ( 'NONE', *, *, #1678, .T. ) ;
#32792=LINE ( 'NONE', #1564, #19109 ) ;
#32794=CARTESIAN_POINT ( 'NONE',  ( 116.0388171295248014, 0.1403307496149613920, -13.39321520033831447 ) ) ;
#32802=EDGE_CURVE ( 'NONE', #14918, #34483, #27857, .T. ) ;
#32812=CARTESIAN_POINT ( 'NONE',  ( 115.3968144685026829, 0.6938714319017630361, -14.64321520033829849 ) ) ;
#32819=CARTESIAN_POINT ( 'NONE',  ( 116.7131856665309186, -6.970574376166484676, -18.05871830232659292 ) ) ;
#32826=CARTESIAN_POINT ( 'NONE',  ( 114.3024890045248156, 0.8980012041604421569, -15.77991374673208469 ) ) ;
#32828=CARTESIAN_POINT ( 'NONE',  ( 112.2188952545247531, -9.868328341294098749, -15.46607636864997204 ) ) ;
#32829=CARTESIAN_POINT ( 'NONE',  ( 109.0935046295247872, -4.863998795839590272, -18.39754474579285315 ) ) ;
#32833=ORIENTED_EDGE ( 'NONE', *, *, #27537, .T. ) ;
#32834=CARTESIAN_POINT ( 'NONE',  ( 107.9128015045248219, -2.477300249445798297, -7.631215200338321125 ) ) ;
#32835=DIRECTION ( 'NONE',  ( -1.000000000000000000, 0.000000000000000000, 0.000000000000000000 ) ) ;
#32841=CARTESIAN_POINT ( 'NONE',  ( 110.1353015045248469, -2.477300249445798297, -7.631215200338321125 ) ) ;
#32842=DIRECTION ( 'NONE',  ( 0.000000000000000000, 0.000000000000000000, -1.000000000000000000 ) ) ;
#32848=DIRECTION ( 'NONE',  ( 1.000000000000000000, 0.000000000000000000, 0.000000000000000000 ) ) ;
#32851=VERTEX_POINT ( 'NONE', #13876 ) ;
#32859=CARTESIAN_POINT ( 'NONE',  ( 107.6349890045248401, -9.868328341294098749, -11.32035403202665869 ) ) ;
#32869=CARTESIAN_POINT ( 'NONE',  ( 62.10597993692722696, -65.36243247205813134, -44.73744814048375673 ) ) ;
#32870=CARTESIAN_POINT ( 'NONE',  ( 107.8433483795247838, -0.7896495226426338832, -9.318865927141430916 ) ) ;
#32875=CARTESIAN_POINT ( 'NONE',  ( 79.05243529145373316, 4.793396140045460108, -12.14321520033831625 ) ) ;
#32879=CARTESIAN_POINT ( 'NONE',  ( 111.1770983795247787, -0.7896495226426338832, -9.318865927141430916 ) ) ;
#32881=CARTESIAN_POINT ( 'NONE',  ( 110.2742077545248094, -7.250697342233347165, -7.631215200338321125 ) ) ;
#32883=ORIENTED_EDGE ( 'NONE', *, *, #3646, .F. ) ;
#32886=CARTESIAN_POINT ( 'NONE',  ( 106.2459265045248173, -7.250697342233347165, -19.15521520033831138 ) ) ;
#32889=CARTESIAN_POINT ( 'NONE',  ( 117.1901992640912908, -11.08276418064105862, -5.403345540909042732 ) ) ;
#32892=CARTESIAN_POINT ( 'NONE',  ( 109.2295201380737097, -10.43748051877606464, -13.15408167448229193 ) ) ;
#32894=CARTESIAN_POINT ( 'NONE',  ( 110.4825671295247815, 0.1403307496149613920, -13.39321520033831447 ) ) ;
#32895=CARTESIAN_POINT ( 'NONE',  ( 115.3442858795247759, -8.402594152722688392, -9.854619843455216355 ) ) ;
#32898=CARTESIAN_POINT ( 'NONE',  ( 70.76896822304256318, -26.49227693691338814, -5.467054258871666406 ) ) ;
#32902=ORIENTED_EDGE ( 'NONE', *, *, #35208, .T. ) ;
#32913=EDGE_CURVE ( 'NONE', #36261, #27061, #27140, .T. ) ;
#32914=CARTESIAN_POINT ( 'NONE',  ( 105.4819421295248247, 0.8980012041604618078, -13.39321520033831447 ) ) ;
#32918=CARTESIAN_POINT ( 'NONE',  ( 112.1494421295248003, -9.868328341294093420, -13.39321520033831447 ) ) ;
#32924=DIRECTION ( 'NONE',  ( -1.000000000000000000, 0.000000000000000000, 0.000000000000000000 ) ) ;
#32926=CARTESIAN_POINT ( 'NONE',  ( 117.0837890045247747, 0.1360012041604422017, -15.46428301220378998 ) ) ;
#32927=CARTESIAN_POINT ( 'NONE',  ( 110.6214733795247867, -1.325403438956436419, -9.854619843455211026 ) ) ;
#32937=DIRECTION ( 'NONE',  ( -1.000000000000000000, -2.775557561562889810E-17, 0.000000000000000000 ) ) ;
#32938=CARTESIAN_POINT ( 'NONE',  ( 109.6491296295247793, -4.863998795839590272, -8.388885654883775800 ) ) ;
#32943=CARTESIAN_POINT ( 'NONE',  ( 108.3295202545248657, -10.62599879583958717, -15.77991374673208469 ) ) ;
#32944=CARTESIAN_POINT ( 'NONE',  ( 61.69189222814998175, -69.76310523276724496, -0.9932152003383157846 ) ) ;
#32945=PLANE ( 'NONE',  #15781 ) ;
#32947=CARTESIAN_POINT ( 'NONE',  ( 112.6356140045247827, -10.62599879583958717, -11.00651665394454604 ) ) ;
#32949=CARTESIAN_POINT ( 'NONE',  ( 83.86184402137078564, -31.76396917189504521, -22.70990857689603004 ) ) ;
#32952=CARTESIAN_POINT ( 'NONE',  ( 106.4542858795248179, -0.7896495226426338832, -17.46756447353520159 ) ) ;
#32965=CARTESIAN_POINT ( 'NONE',  ( 107.2877233795247776, -8.938348069036489818, -17.46756447353520159 ) ) ;
#32966=AXIS2_PLACEMENT_3D ( 'NONE', #11298, #18367, #1251 ) ;
#32969=CARTESIAN_POINT ( 'NONE',  ( 115.8999108795247821, -8.938348069036489818, -9.318865927141430916 ) ) ;
#32991=CARTESIAN_POINT ( 'NONE',  ( 115.4137390045248566, -9.868328341294098749, -11.32035403202665869 ) ) ;
#32995=CARTESIAN_POINT ( 'NONE',  ( 114.7886608795247696, -8.938348069036489818, -9.318865927141430916 ) ) ;
#32996=CARTESIAN_POINT ( 'NONE',  ( 108.3989733795248753, -1.325403438956436419, -9.854619843455211026 ) ) ;
#33006=CARTESIAN_POINT ( 'NONE',  ( 107.2294421295247844, -9.051693226400931991, -21.89321520033831447 ) ) ;
#33007=CARTESIAN_POINT ( 'NONE',  ( 108.9545983795247821, -8.402594152722688392, -16.93181055722141792 ) ) ;
#33011=B_SPLINE_CURVE_WITH_KNOTS ( 'NONE', 3,
 ( #4691, #21353, #7896, #11550, #38665, #35924, #4472, #39129, #7433, #24559, #18610, #18159, #29092, #38445, #35237, #11099, #42117, #28654, #28427, #25232, #32055, #1276, #10877, #32502, #15188, #42340, #43003, #822, #35003, #14291, #14964, #3786, #38895, #21803, #39361, #4013, #14743, #7216, #21128, #1049, #42560, #28877, #17936, #18392, #42789 ),
 .UNSPECIFIED., .F., .F.,
 ( 4, 2, 2, 1, 1, 1, 2, 2, 2, 2, 1, 1, 1, 2, 2, 2, 2, 1, 1, 1, 2, 2, 2, 2, 2, 2, 4 ),
 ( 0.000000000000000000, 0.06250000000006793177, 0.09375000000010108581, 0.1093750000001167677, 0.1171875000001246087, 0.1210937500001285361, 0.1230468750001315892, 0.1250000000001346423, 0.1875000000002185752, 0.2187500000002587930, 0.2343750000002789158, 0.2421875000002898515, 0.2460937500002960687, 0.2480468750002971789, 0.2500000000002982614, 0.3750000000003029799, 0.4375000000003045897, 0.4687500000003050338, 0.4843750000003049228, 0.4921875000003033129, 0.4960937500003007039, 0.5000000000002979839, 0.6250000000002219336, 0.6875000000001831868, 0.7187500000001638689, 0.7500000000001444400, 1.000000000000000000 ),
 .UNSPECIFIED. ) ;
#33018=CARTESIAN_POINT ( 'NONE',  ( 112.8439733795247832, -1.325403438956436419, -9.854619843455211026 ) ) ;
#33030=CARTESIAN_POINT ( 'NONE',  ( 65.49983523453742862, -18.16718729050178993, -4.893215200338314474 ) ) ;
#33031=CARTESIAN_POINT ( 'NONE',  ( 65.19189222814998175, -41.76310523276723785, -24.39321520033831447 ) ) ;
#33038=CARTESIAN_POINT ( 'NONE',  ( 116.7263990467714194, -6.377543297015642487, -18.31558037743933909 ) ) ;
#33046=CARTESIAN_POINT ( 'NONE',  ( 113.1912390045248031, 0.8980012041604421569, -15.77991374673208469 ) ) ;
#33047=CARTESIAN_POINT ( 'NONE',  ( 111.5938171295247940, 0.1403307496149613920, -13.39321520033831447 ) ) ;
#33048=CARTESIAN_POINT ( 'NONE',  ( 109.4407702545248355, 0.1403307496149616695, -11.32035403202665336 ) ) ;
#33053=FACE_OUTER_BOUND ( 'NONE', #31161, .T. ) ;
#33058=CARTESIAN_POINT ( 'NONE',  ( 109.4407702545248355, -10.62599879583958717, -15.77991374673208469 ) ) ;
#33059=CARTESIAN_POINT ( 'NONE',  ( 66.06194382436763135, -14.97931106434683635, -4.893215200338314474 ) ) ;
#33060=ORIENTED_EDGE ( 'NONE', *, *, #28100, .T. ) ;
#33067=( BOUNDED_CURVE ( )  B_SPLINE_CURVE ( 3, ( #23365, #27468, #40930, #13339 ),
 .UNSPECIFIED., .F., .T. ) 
 B_SPLINE_CURVE_WITH_KNOTS ( ( 4, 4 ),
 ( 0.000000000000000000, 3.141592653589795336 ),
 .UNSPECIFIED. ) 
 CURVE ( )  GEOMETRIC_REPRESENTATION_ITEM ( )  RATIONAL_B_SPLINE_CURVE ( ( 1.000000000000000000, 0.3333333333333335369, 0.3333333333333335369, 1.000000000000000000 ) ) 
 REPRESENTATION_ITEM ( '' )  );
#33075=ORIENTED_EDGE ( 'NONE', *, *, #16974, .T. ) ;
#33079=CARTESIAN_POINT ( 'NONE',  ( 115.3442858795247759, -0.7896495226426338832, -17.46756447353520159 ) ) ;
#33090=CARTESIAN_POINT ( 'NONE',  ( 61.80337255853385869, -65.85056717495680800, -43.64372168240947758 ) ) ;
#33097=LINE ( 'NONE', #14900, #3629 ) ;
#33103=CARTESIAN_POINT ( 'NONE',  ( 110.7603796295247918, -4.863998795839590272, -19.15521520033831493 ) ) ;
#33105=CARTESIAN_POINT ( 'NONE',  ( 109.7880358795247986, -0.7896495226426338832, -17.46756447353520159 ) ) ;
#33108=ADVANCED_FACE ( 'NONE', ( #13391 ), #3336, .F. ) ;
#33110=CARTESIAN_POINT ( 'NONE',  ( 63.14350240710648876, -37.75742606650420896, -4.969760221102785813 ) ) ;
#33111=CARTESIAN_POINT ( 'NONE',  ( 108.6073327545248048, -2.477300249445798297, -19.15521520033831138 ) ) ;
#33114=EDGE_CURVE ( 'NONE', #28792, #40778, #24320, .T. ) ;
#33118=CARTESIAN_POINT ( 'NONE',  ( 116.7327219861001879, -11.78583009060342413, -6.254644069865828548 ) ) ;
#33119=ORIENTED_EDGE ( 'NONE', *, *, #16104, .F. ) ;
#33120=CARTESIAN_POINT ( 'NONE',  ( 109.2294424962575050, -10.05627679606856795, -15.17422528748209665 ) ) ;
#33122=CARTESIAN_POINT ( 'NONE',  ( 113.4690515045247992, -6.936859964151250502, -18.39754474579286025 ) ) ;
#33123=CARTESIAN_POINT ( 'NONE',  ( 109.5102233795247884, -1.325403438956436419, -9.854619843455211026 ) ) ;
#33125=FACE_OUTER_BOUND ( 'NONE', #34638, .T. ) ;
#33126=CARTESIAN_POINT ( 'NONE',  ( 69.77898898320889032, -25.66191150022318723, -5.787138065658675501 ) ) ;
#33136=AXIS2_PLACEMENT_3D ( 'NONE', #31041, #44971, #13728 ) ;
#33144=CARTESIAN_POINT ( 'NONE',  ( 110.4131140045248287, 0.1403307496149616695, -15.46607636864997204 ) ) ;
#33149=CARTESIAN_POINT ( 'NONE',  ( 87.44708369096657918, -25.99489077589583630, -8.393215200338314474 ) ) ;
#33151=CARTESIAN_POINT ( 'NONE',  ( 116.2503515045248719, -2.792930983974093007, -8.393215200338321580 ) ) ;
#33152=CARTESIAN_POINT ( 'NONE',  ( 108.4684265045247997, -2.791137627527939813, -8.388885654883777576 ) ) ;
#33159=CIRCLE ( 'NONE', #6243, 4.000000000000000000 ) ;
#33164=CARTESIAN_POINT ( 'NONE',  ( 110.9687390045248350, -9.868328341294098749, -11.32035403202665869 ) ) ;
#33165=EDGE_CURVE ( 'NONE', #22218, #17767, #27516, .T. ) ;
#33169=CARTESIAN_POINT ( 'NONE',  ( 107.0099108795247815, -8.938348069036489818, -9.318865927141430916 ) ) ;
#33172=CARTESIAN_POINT ( 'NONE',  ( 111.9410827545248708, -2.477300249445798297, -19.15521520033831138 ) ) ;
#33174=CARTESIAN_POINT ( 'NONE',  ( 117.2294421295248270, 0.5103437856549055684, -21.89321520033831803 ) ) ;
#33177=CARTESIAN_POINT ( 'NONE',  ( 108.3295202545248657, -10.62599879583958717, -15.77991374673208469 ) ) ;
#33180=CARTESIAN_POINT ( 'NONE',  ( 61.69189222814998175, -49.76310523276723785, -13.39321520033831447 ) ) ;
#33182=DIRECTION ( 'NONE',  ( 0.000000000000000000, 0.000000000000000000, -1.000000000000000000 ) ) ;
#33192=CARTESIAN_POINT ( 'NONE',  ( 110.4131140045248287, -10.62599879583958717, -11.00651665394454604 ) ) ;
#33194=CARTESIAN_POINT ( 'NONE',  ( 116.7654395844541284, -4.393248286083126786, -18.55097782704973497 ) ) ;
#33204=CARTESIAN_POINT ( 'NONE',  ( 115.1139883310706722, 0.1843591316377651834, -12.14321520033831625 ) ) ;
#33209=EDGE_CURVE ( 'NONE', #35524, #24941, #34769, .T. ) ;
#33210=CARTESIAN_POINT ( 'NONE',  ( 109.7922320646196823, 0.6269505268395592079, -14.64321520033831447 ) ) ;
#33217=ORIENTED_EDGE ( 'NONE', *, *, #32152, .F. ) ;
#33220=CARTESIAN_POINT ( 'NONE',  ( 116.9417077545247992, -2.791137627527939813, -18.39754474579286025 ) ) ;
#33224=CARTESIAN_POINT ( 'NONE',  ( 113.3995983795247895, -0.7896495226426338832, -9.318865927141430916 ) ) ;
#33225=CARTESIAN_POINT ( 'NONE',  ( 108.4684265045248424, -2.791137627527939813, -8.388885654883777576 ) ) ;
#33230=VECTOR ( 'NONE', #25798, 1000.000000000000000 ) ;
#33231=CARTESIAN_POINT ( 'NONE',  ( 113.7468640045248236, 0.1403307496149616695, -15.46607636864997204 ) ) ;
#33237=DIRECTION ( 'NONE',  ( -1.000000000000000000, 0.000000000000000000, 0.000000000000000000 ) ) ;
#33238=CARTESIAN_POINT ( 'NONE',  ( 109.7185827545247889, -6.936859964151250502, -8.388885654883777576 ) ) ;
#33248=CARTESIAN_POINT ( 'NONE',  ( 112.6356140045247827, 0.1403307496149616695, -15.46607636864997204 ) ) ;
#33249=EDGE_CURVE ( 'NONE', #31523, #37055, #7641, .T. ) ;
#33260=DIRECTION ( 'NONE',  ( -1.000000000000000000, 0.000000000000000000, 0.000000000000000000 ) ) ;
#33276=CARTESIAN_POINT ( 'NONE',  ( 113.3995983795247895, -0.7896495226426338832, -9.318865927141430916 ) ) ;
#33277=CARTESIAN_POINT ( 'NONE',  ( 110.7603796295247918, -4.863998795839590272, -8.388885654883775800 ) ) ;
#33278=CARTESIAN_POINT ( 'NONE',  ( 107.9128015045248219, -6.936859964151250502, -18.39754474579286025 ) ) ;
#33281=ORIENTED_EDGE ( 'NONE', *, *, #5077, .T. ) ;
#33284=DIRECTION ( 'NONE',  ( 1.000000000000000000, 0.000000000000000000, 0.000000000000000000 ) ) ;
#33287=CARTESIAN_POINT ( 'NONE',  ( 110.2742077545248094, -7.250697342233347165, -7.631215200338321125 ) ) ;
#33288=DIRECTION ( 'NONE',  ( 0.000000000000000000, 0.000000000000000000, 1.000000000000000000 ) ) ;
#33295=DIRECTION ( 'NONE',  ( -1.000000000000000000, 0.000000000000000000, 0.000000000000000000 ) ) ;
#33298=EDGE_LOOP ( 'NONE', ( #31108, #43586, #10467, #10790 ) ) ;
#33306=CARTESIAN_POINT ( 'NONE',  ( 112.7745202545247878, -10.62599879583958717, -15.77991374673208469 ) ) ;
#33313=DIRECTION ( 'NONE',  ( 0.000000000000000000, 1.000000000000000000, 1.069961080215129965E-32 ) ) ;
#33315=CARTESIAN_POINT ( 'NONE',  ( 105.6208483795248299, -0.7896495226426338832, -9.318865927141430916 ) ) ;
#33321=CARTESIAN_POINT ( 'NONE',  ( 143.3676850761856940, -59.27884951796255564, -42.87418841894956500 ) ) ;
#33322=ORIENTED_EDGE ( 'NONE', *, *, #30301, .T. ) ;
#33325=CARTESIAN_POINT ( 'NONE',  ( 112.0105358795247810, -0.7896495226426338832, -17.46756447353520159 ) ) ;
#33326=CARTESIAN_POINT ( 'NONE',  ( 114.7192077545248594, -2.791137627527939813, -18.39754474579286025 ) ) ;
#33327=CARTESIAN_POINT ( 'NONE',  ( 113.1217858795247935, -0.7896495226426338832, -17.46756447353520159 ) ) ;
#33329=ORIENTED_EDGE ( 'NONE', *, *, #43752, .T. ) ;
#33332=CARTESIAN_POINT ( 'NONE',  ( 107.0099108795247815, -8.938348069036489818, -9.318865927141430916 ) ) ;
#33340=CARTESIAN_POINT ( 'NONE',  ( 109.2292810560890786, -10.43422423177587000, -12.93205439691941017 ) ) ;
#33342=CARTESIAN_POINT ( 'NONE',  ( 112.4967077545247633, -2.791137627527939813, -18.39754474579286025 ) ) ;
#33343=CARTESIAN_POINT ( 'NONE',  ( 111.8716296295247901, -4.863998795839590272, -8.388885654883775800 ) ) ;
#33346=CARTESIAN_POINT ( 'NONE',  ( 69.68376945742858197, -25.46719311063753466, -5.786137840895125173 ) ) ;
#33356=ORIENTED_EDGE ( 'NONE', *, *, #17301, .T. ) ;
#33362=CARTESIAN_POINT ( 'NONE',  ( 107.9128015045248219, -2.477300249445798297, -7.631215200338321125 ) ) ;
#33367=CARTESIAN_POINT ( 'NONE',  ( 110.6214733795247867, -1.325403438956436419, -9.854619843455211026 ) ) ;
#33379=CARTESIAN_POINT ( 'NONE',  ( 70.79387962571317416, -26.49875194020793501, -5.426084794384776977 ) ) ;
#33382=ORIENTED_EDGE ( 'NONE', *, *, #19468, .T. ) ;
#33385=CARTESIAN_POINT ( 'NONE',  ( 111.6632702545248605, 0.1403307496149616695, -11.32035403202665336 ) ) ;
#33389=CARTESIAN_POINT ( 'NONE',  ( 115.8304577545247582, -2.791137627527939813, -18.39754474579286025 ) ) ;
#33392=CARTESIAN_POINT ( 'NONE',  ( 61.69189222814998175, -40.21211973637273474, -19.39321520033831447 ) ) ;
#33393=CARTESIAN_POINT ( 'NONE',  ( 111.1770983795247787, -0.7896495226426338832, -9.318865927141430916 ) ) ;
#33395=CARTESIAN_POINT ( 'NONE',  ( 113.0523327545247838, -2.477300249445798297, -19.15521520033831138 ) ) ;
#33398=CARTESIAN_POINT ( 'NONE',  ( 106.7320983795247855, -0.7896495226426338832, -9.318865927141430916 ) ) ;
#33410=CARTESIAN_POINT ( 'NONE',  ( 108.3989733795248753, -8.938348069036489818, -17.46756447353520159 ) ) ;
#33412=CARTESIAN_POINT ( 'NONE',  ( 116.7902762465598840, -3.170093105002864231, -18.30519083512918854 ) ) ;
#33413=CARTESIAN_POINT ( 'NONE',  ( 64.80455967515507609, -63.24213094532785107, -47.38765000594077037 ) ) ;
#33416=ADVANCED_FACE ( 'NONE', ( #4218 ), #18134, .T. ) ;
#33422=ADVANCED_FACE ( 'NONE', ( #31586 ), #42537, .T. ) ;
#33423=DIRECTION ( 'NONE',  ( 0.000000000000000000, 0.000000000000000000, 1.000000000000000000 ) ) ;
#33424=CARTESIAN_POINT ( 'NONE',  ( 105.6208483795248299, -8.402594152722688392, -16.93181055722141792 ) ) ;
#33434=CARTESIAN_POINT ( 'NONE',  ( 113.9552233795247815, -1.325403438956436419, -9.854619843455211026 ) ) ;
#33438=CARTESIAN_POINT ( 'NONE',  ( 115.1359265045248605, -7.250697342233347165, -19.15521520033831138 ) ) ;
#33439=CARTESIAN_POINT ( 'NONE',  ( 107.2182702545248105, 0.1403307496149616695, -11.32035403202665336 ) ) ;
#33440=CARTESIAN_POINT ( 'NONE',  ( 83.23380393269211197, -31.93623664265597739, -23.45566856608283501 ) ) ;
#33445=CARTESIAN_POINT ( 'NONE',  ( 111.3854577545248645, -2.791137627527939813, -18.39754474579286025 ) ) ;
#33447=CARTESIAN_POINT ( 'NONE',  ( 109.2296023670620571, -0.1266929509688458910, -15.29689100126300083 ) ) ;
#33452=CARTESIAN_POINT ( 'NONE',  ( 143.3676850761856940, -55.76602098829192755, -2.607500914624014232 ) ) ;
#33453=CARTESIAN_POINT ( 'NONE',  ( 116.9052633095559770, -11.62205044407607879, -21.51620027165634497 ) ) ;
#33461=CYLINDRICAL_SURFACE ( 'NONE', #30049, 3.000000000000001332 ) ;
#33462=CARTESIAN_POINT ( 'NONE',  ( 71.83824405425508530, -26.34469659010723674, -4.893215200338314474 ) ) ;
#33464=ADVANCED_FACE ( 'NONE', ( #356 ), #14267, .F. ) ;
#33465=CARTESIAN_POINT ( 'NONE',  ( 113.8163171295247764, 0.1403307496149613920, -13.39321520033831447 ) ) ;
#33473=ORIENTED_EDGE ( 'NONE', *, *, #26253, .F. ) ;
#33475=EDGE_CURVE ( 'NONE', #38699, #40576, #7874, .T. ) ;
#33479=LINE ( 'NONE', #41044, #27699 ) ;
#33480=CARTESIAN_POINT ( 'NONE',  ( 114.8834831777918879, -0.01829820670803256055, -14.64321520033831447 ) ) ;
#33493=ORIENTED_EDGE ( 'NONE', *, *, #16277, .F. ) ;
#33495=CARTESIAN_POINT ( 'NONE',  ( 113.9552233795247815, -8.938348069036489818, -17.46756447353520159 ) ) ;
#33496=CARTESIAN_POINT ( 'NONE',  ( 109.2324108795247923, -1.325403438956436419, -16.93181055722141792 ) ) ;
#33497=CARTESIAN_POINT ( 'NONE',  ( 107.7738952545248310, -9.868328341294098749, -15.46607636864997204 ) ) ;
#33498=CARTESIAN_POINT ( 'NONE',  ( 64.25426170852544772, -36.05670985702485609, -5.755590974858822761 ) ) ;
#33502=CARTESIAN_POINT ( 'NONE',  ( 109.2294601086458954, -8.543441930476365798, -8.974638458010995024 ) ) ;
#33505=CARTESIAN_POINT ( 'NONE',  ( 105.9681140045248355, 0.1403307496149616695, -15.46607636864997204 ) ) ;
#33507=CARTESIAN_POINT ( 'NONE',  ( 108.1211608795247798, -8.938348069036489818, -9.318865927141430916 ) ) ;
#33509=ORIENTED_EDGE ( 'NONE', *, *, #27537, .F. ) ;
#33525=CIRCLE ( 'NONE', #13894, 2.000000000000003109 ) ;
#33529=CARTESIAN_POINT ( 'NONE',  ( 114.1635827545248389, -2.477300249445798297, -19.15521520033831138 ) ) ;
#33534=EDGE_CURVE ( 'NONE', #32851, #34946, #25655, .T. ) ;
#33539=CARTESIAN_POINT ( 'NONE',  ( 106.0375671295248310, -10.62599879583958540, -13.39321520033831447 ) ) ;
#33546=ORIENTED_EDGE ( 'NONE', *, *, #6115, .F. ) ;
#33550=CARTESIAN_POINT ( 'NONE',  ( 113.3995983795247895, -0.7896495226426338832, -9.318865927141430916 ) ) ;
#33552=CARTESIAN_POINT ( 'NONE',  ( 111.8716296295247901, -4.863998795839590272, -8.388885654883775800 ) ) ;
#33553=CARTESIAN_POINT ( 'NONE',  ( 113.8163171295247764, -10.62599879583958540, -13.39321520033831447 ) ) ;
#33555=ORIENTED_EDGE ( 'NONE', *, *, #37683, .T. ) ;
#33559=FACE_OUTER_BOUND ( 'NONE', #7759, .T. ) ;
#33567=CARTESIAN_POINT ( 'NONE',  ( 70.36267391504958368, -5.685877709920885259, -4.893215200338314474 ) ) ;
#33571=CARTESIAN_POINT ( 'NONE',  ( 109.2324108795247923, -1.325403438956436419, -16.93181055722141792 ) ) ;
#33572=CARTESIAN_POINT ( 'NONE',  ( 111.9410827545248708, -6.936859964151250502, -8.388885654883777576 ) ) ;
#33575=CARTESIAN_POINT ( 'NONE',  ( 70.87679208027947197, -26.22245083233618601, -5.471004667883966555 ) ) ;
#33583=PRODUCT_DEFINITION ( 'UNKNOWN', '', #3109, #36051 ) ;
#33587=AXIS2_PLACEMENT_3D ( 'NONE', #39923, #22588, #33284 ) ;
#33591=CARTESIAN_POINT ( 'NONE',  ( 108.6073327545248048, -2.477300249445798297, -19.15521520033831138 ) ) ;
#33595=CARTESIAN_POINT ( 'NONE',  ( 110.9687390045248350, -9.868328341294098749, -11.32035403202665869 ) ) ;
#33596=DIRECTION ( 'NONE',  ( 0.000000000000000000, 0.000000000000000000, -1.000000000000000000 ) ) ;
#33601=DIRECTION ( 'NONE',  ( 0.000000000000000000, 0.7876185884367603585, -0.6161630946014904353 ) ) ;
#33603=DIRECTION ( 'NONE',  ( 1.000000000000000000, 0.000000000000000000, 0.000000000000000000 ) ) ;
#33610=ORIENTED_EDGE ( 'NONE', *, *, #25664, .F. ) ;
#33611=CARTESIAN_POINT ( 'NONE',  ( 114.6460952706805756, 0.3193521225029610777, -14.64321520033831447 ) ) ;
#33613=CARTESIAN_POINT ( 'NONE',  ( 109.5796765045248122, -2.791137627527939813, -8.388885654883777576 ) ) ;
#33617=CARTESIAN_POINT ( 'NONE',  ( 106.0375671295248310, -10.62599879583958540, -13.39321520033831447 ) ) ;
#33619=LINE ( 'NONE', #40953, #37540 ) ;
#33622=CARTESIAN_POINT ( 'NONE',  ( 112.0105358795247810, -0.7896495226426338832, -17.46756447353520159 ) ) ;
#33624=CARTESIAN_POINT ( 'NONE',  ( 113.1217858795247935, -0.7896495226426338832, -17.46756447353520159 ) ) ;
#33627=CARTESIAN_POINT ( 'NONE',  ( 114.5803015045248259, -2.477300249445798297, -7.631215200338321125 ) ) ;
#33642=CARTESIAN_POINT ( 'NONE',  ( 111.2465515045248168, -2.477300249445798297, -7.631215200338321125 ) ) ;
#33649=EDGE_CURVE ( 'NONE', #29947, #25821, #19482, .T. ) ;
#33650=CARTESIAN_POINT ( 'NONE',  ( 113.6079577545248185, -2.791137627527887410, -18.39754474579284249 ) ) ;
#33655=CARTESIAN_POINT ( 'NONE',  ( 107.8433483795247838, -8.402594152722688392, -16.93181055722141792 ) ) ;
#33666=CARTESIAN_POINT ( 'NONE',  ( 115.2053796295247849, -4.863998795839590272, -8.388885654883775800 ) ) ;
#33672=CARTESIAN_POINT ( 'NONE',  ( 115.4137390045248566, 0.8980012041604421569, -15.77991374673208469 ) ) ;
#33673=CARTESIAN_POINT ( 'NONE',  ( 108.6767858795247861, -8.402594152722688392, -9.854619843455216355 ) ) ;
#33678=CARTESIAN_POINT ( 'NONE',  ( 70.19189222814998175, -42.69543048370626792, -27.04993751765913501 ) ) ;
#33679=CARTESIAN_POINT ( 'NONE',  ( 115.2748327545248657, -6.936859964151250502, -8.388885654883777576 ) ) ;
#33681=EDGE_CURVE ( 'NONE', #35835, #8254, #17691, .T. ) ;
#33691=CARTESIAN_POINT ( 'NONE',  ( 116.8978462035280330, -11.63045278355507328, -21.50838919663385340 ) ) ;
#33697=( LENGTH_UNIT ( ) NAMED_UNIT ( * ) SI_UNIT ( .MILLI., .METRE. ) );
#33701=CARTESIAN_POINT ( 'NONE',  ( 113.3301452545248083, -9.868328341294098749, -15.46607636864997204 ) ) ;
#33703=DIRECTION ( 'NONE',  ( 0.000000000000000000, 0.000000000000000000, -1.000000000000000000 ) ) ;
#33707=TOROIDAL_SURFACE ( 'NONE', #43926, 7.132259260909269649, 2.000000000000000000 ) ;
#33708=DIRECTION ( 'NONE',  ( 0.000000000000000000, -0.9284778069183718952, -0.3713878862591650232 ) ) ;
#33713=PLANE ( 'NONE',  #38327 ) ;
#33714=CARTESIAN_POINT ( 'NONE',  ( 110.0658483795247804, -8.402594152722633325, -16.93181055722145345 ) ) ;
#33732=CARTESIAN_POINT ( 'NONE',  ( 112.7050671295247923, -10.62599879583958540, -13.39321520033831447 ) ) ;
#33733=CARTESIAN_POINT ( 'NONE',  ( 105.4819421295248247, -9.868328341294093420, -13.39321520033831447 ) ) ;
#33745=CARTESIAN_POINT ( 'NONE',  ( 107.9822546295247889, -4.863998795839590272, -7.631215200338315796 ) ) ;
#33746=FACE_OUTER_BOUND ( 'NONE', #39016, .T. ) ;
#33747=ORIENTED_EDGE ( 'NONE', *, *, #35001, .T. ) ;
#33754=LINE ( 'NONE', #12581, #3801 ) ;
#33766=CARTESIAN_POINT ( 'NONE',  ( 111.3160046295247838, -4.863998795839590272, -7.631215200338315796 ) ) ;
#33775=CARTESIAN_POINT ( 'NONE',  ( 105.8292077545248446, -7.250697342233347165, -7.631215200338321125 ) ) ;
#33785=CARTESIAN_POINT ( 'NONE',  ( 108.3989733795248753, -8.938348069036489818, -17.46756447353520159 ) ) ;
#33786=CARTESIAN_POINT ( 'NONE',  ( 111.1770983795247787, -8.402594152722688392, -16.93181055722141792 ) ) ;
#33787=CARTESIAN_POINT ( 'NONE',  ( 112.0799890045248475, 0.8980012041604421569, -15.77991374673208469 ) ) ;
#33805=CARTESIAN_POINT ( 'NONE',  ( 106.7320983795247855, -8.402594152722688392, -16.93181055722141792 ) ) ;
#33806=CARTESIAN_POINT ( 'NONE',  ( 110.4131140045248287, 0.1403307496149616695, -15.46607636864997204 ) ) ;
#33808=CARTESIAN_POINT ( 'NONE',  ( 70.72798458804651034, -25.12338242182658732, -5.471004667884126427 ) ) ;
#33830=CARTESIAN_POINT ( 'NONE',  ( 109.1629577545248395, -2.791137627527939813, -18.39754474579286025 ) ) ;
#33840=FACE_OUTER_BOUND ( 'NONE', #177, .T. ) ;
#33848=CARTESIAN_POINT ( 'NONE',  ( 115.6220983795247861, -0.7896495226426338832, -9.318865927141430916 ) ) ;
#33851=CARTESIAN_POINT ( 'NONE',  ( 112.2188952545247531, -9.868328341294102302, -15.46607636865001645 ) ) ;
#33852=CARTESIAN_POINT ( 'NONE',  ( 115.1359265045248605, -2.791137627527939813, -8.388885654883777576 ) ) ;
#33853=DIRECTION ( 'NONE',  ( -0.6836572958096076569, 0.7298031939408696767, 0.000000000000000000 ) ) ;
#33856=CARTESIAN_POINT ( 'NONE',  ( 111.2465515045248168, -2.477300249445798297, -7.631215200338321125 ) ) ;
#33858=CARTESIAN_POINT ( 'NONE',  ( 112.2188952545247531, 0.8980012041604421569, -11.00651665394454071 ) ) ;
#33861=CARTESIAN_POINT ( 'NONE',  ( 114.8581140045248361, -10.62599879583958540, -11.00651665394454604 ) ) ;
#33864=ORIENTED_EDGE ( 'NONE', *, *, #15526, .F. ) ;
#33875=CARTESIAN_POINT ( 'NONE',  ( 111.6632702545248605, 0.1403307496149616695, -11.32035403202665336 ) ) ;
#33877=CARTESIAN_POINT ( 'NONE',  ( 116.8415777867357406, -0.9725888463086822533, -16.91308624977476072 ) ) ;
#33878=CARTESIAN_POINT ( 'NONE',  ( 116.5944421295247793, 0.8980012041604618078, -13.39321520033831447 ) ) ;
#33884=CARTESIAN_POINT ( 'NONE',  ( 117.0283149730835959, 1.730878968199667245, -5.544651811887305826 ) ) ;
#33885=CARTESIAN_POINT ( 'NONE',  ( 114.1406031537514849, 0.4930828106259610433, -14.64321520033831447 ) ) ;
#33886=CARTESIAN_POINT ( 'NONE',  ( 105.6903015045248253, -6.936859964151250502, -18.39754474579286025 ) ) ;
#33890=CIRCLE ( 'NONE', #9873, 0.9999999999999952260 ) ;
#33902=CARTESIAN_POINT ( 'NONE',  ( 111.8716296295247901, -4.863998795839590272, -19.15521520033831493 ) ) ;
#33904=CARTESIAN_POINT ( 'NONE',  ( 83.11819775781678743, -31.88128537155179743, -23.36558840204159537 ) ) ;
#33907=CARTESIAN_POINT ( 'NONE',  ( 112.8439888068194819, 0.1168444861213632779, -12.14321520033831625 ) ) ;
#33908=CARTESIAN_POINT ( 'NONE',  ( 115.6915515045247531, -6.936859964151250502, -18.39754474579286025 ) ) ;
#33909=ORIENTED_EDGE ( 'NONE', *, *, #8308, .F. ) ;
#33917=CARTESIAN_POINT ( 'NONE',  ( 116.5799884964095270, -11.88873078449987375, -21.18799803434260554 ) ) ;
#33929=CARTESIAN_POINT ( 'NONE',  ( 110.1353015045248469, -6.936859964151250502, -18.39754474579286025 ) ) ;
#33932=CARTESIAN_POINT ( 'NONE',  ( 86.51169734173754478, -25.99489077589583630, -8.393215200338314474 ) ) ;
#33939=VERTEX_POINT ( 'NONE', #21132 ) ;
#33948=EDGE_CURVE ( 'NONE', #7036, #35580, #37011, .T. ) ;
#33962=CARTESIAN_POINT ( 'NONE',  ( 111.1076452545248259, 0.8980012041604421569, -11.00651665394454071 ) ) ;
#33964=CARTESIAN_POINT ( 'NONE',  ( 105.3430358795248338, -8.402594152722688392, -9.854619843455216355 ) ) ;
#33965=CARTESIAN_POINT ( 'NONE',  ( 106.3153796295248412, -4.863998795839590272, -8.388885654883775800 ) ) ;
#33975=CARTESIAN_POINT ( 'NONE',  ( 114.3719421295247827, -9.868328341294093420, -13.39321520033831447 ) ) ;
#33996=CARTESIAN_POINT ( 'NONE',  ( 110.6214733795247867, -8.938348069036489818, -17.46756447353520159 ) ) ;
#34004=EDGE_CURVE ( 'NONE', #34659, #42684, #40479, .T. ) ;
#34012=( BOUNDED_SURFACE ( )  B_SPLINE_SURFACE ( 1, 2, ( 
 ( #44645, #38009, #6783, #20693, #34571, #24338, #31380, #32497, #34999, #1045, #7212, #376, #28650, #11318, #25228, #18156, #24997, #17707, #31831, #3783, #11096, #42114, #42335, #31607, #10650, #4685, #8124, #14512, #22026, #10874, #24556, #35919, #7429, #38442, #35693, #4469, #39126, #14287, #21125, #28206, #24769, #38660, #38892, #39356, #42556, #819, #14961, #21350, #35234, #4010, #7893, #25454, #28424, #7661, #17932, #21799, #18389, #601, #32277, #28873, #14738, #29087, #42786, #11547, #21576, #1272, #35463, #4238, #32052, #18606, #15184, #19506, #16086, #16318, #19285, #40026, #42999, #1940, #2157, #33385, #1713, #29991, #43908, #12677, #2390, #5809, #26575, #40489, #12221, #33164, #11767, #29315, #26120, #8790, #15866, #15411, #43228, #25897, #15637, #36814, #9248, #23157, #25676, #29762, #37039, #11995, #19727, #22696, #32938, #33613, #36593, #32717, #43674, #26350, #39582, #8344, #5368, #12449, #40258, #22245, #36141, #39801, #5136, #4909, #9024, #22922, #5582, #29541, #43457, #18825, #1489, #8570, #22470, #36364, #19052, #10159, #23616, #45036, #23847, #40712, #37958, #34080, #37267, #2847, #26802, #9702, #24287, #9472, #20643, #27708, #41622, #40946, #3298, #41174, #16777, #12906, #30221, #10378, #34735, #23383, #37502 ),
 ( #13796, #17005, #20420, #34520, #6037, #19959, #16549, #30894, #38173, #30671, #44592, #6276, #41403, #6733, #33848, #13574, #3076, #34303, #3518, #24067, #31111, #20196, #20857, #13355, #30445, #44364, #6952, #44141, #17221, #2617, #13126, #6505, #27259, #27031, #44816, #9934, #37734, #27484, #21749, #39074, #7843, #21973, #25402, #35640, #996, #31777, #38840, #35860, #3735, #548, #14460, #7609, #34949, #17658, #322, #35181, #11268, #32223, #14911, #31329, #21523, #28822, #31554, #42732, #28367, #7381, #11497, #42280, #7160, #35410, #761, #103, #4416, #11042, #4185, #24944, #39300, #17436, #14235, #24716, #24503, #18103, #31998, #14683, #21298, #17880, #18330, #14016, #28597, #42508, #21072, #10600, #8070, #41840, #27931, #38387, #28151, #42061, #10819, #25176, #38605, #3958, #39973, #40203, #11716, #25627, #36091, #5314, #19449, #22420, #8517, #15360, #15808, #12396, #39532, #33111, #22644, #8736, #23102, #29709, #5530, #11945, #40434, #39749, #4862, #18780, #29942, #43855, #26296, #22868, #4634, #26069, #1660, #18555, #36540, #8969, #36761, #36313, #33332, #2106, #16034, #9195, #12627, #26525, #32447, #18999, #19230, #1221, #32670, #32886, #15582, #1881, #22195, #1438, #29265, #5083, #43622, #15135, #29041, #42950, #8293 ) ),
 .UNSPECIFIED., .F., .F., .T. ) 
 B_SPLINE_SURFACE_WITH_KNOTS ( ( 2, 2 ),
 ( 3, 2, 2, 2, 2, 2, 2, 2, 2, 2, 2, 2, 2, 2, 2, 2, 2, 2, 2, 2, 2, 2, 2, 2, 2, 2, 2, 2, 2, 2, 2, 2, 2, 2, 2, 2, 2, 2, 2, 2, 2, 2, 2, 2, 2, 2, 2, 2, 2, 2, 2, 2, 2, 2, 2, 2, 2, 2, 2, 2, 2, 2, 2, 2, 2, 2, 2, 2, 2, 2, 2, 2, 2, 2, 2, 2, 2, 2, 2, 2, 3 ),
 ( 0.000000000000000000, 1.000000000000000000 ),
 ( 0.000000000000000000, 0.01250000000000000069, 0.02500000000000000139, 0.03749999999999999861, 0.05000000000000000278, 0.06250000000000000000, 0.07499999999999999722, 0.08749999999999999445, 0.1000000000000000056, 0.1125000000000000028, 0.1250000000000000000, 0.1375000000000000111, 0.1499999999999999944, 0.1625000000000000056, 0.1749999999999999889, 0.1875000000000000000, 0.2000000000000000111, 0.2124999999999999944, 0.2250000000000000056, 0.2374999999999999889, 0.2500000000000000000, 0.2625000000000000111, 0.2750000000000000222, 0.2874999999999999778, 0.2999999999999999889, 0.3125000000000000000, 0.3250000000000000111, 0.3375000000000000222, 0.3499999999999999778, 0.3624999999999999889, 0.3750000000000000000, 0.3875000000000000111, 0.4000000000000000222, 0.4124999999999999778, 0.4249999999999999889, 0.4375000000000000000, 0.4500000000000000111, 0.4625000000000000222, 0.4749999999999999778, 0.4874999999999999889, 0.5000000000000000000, 0.5124999999999999556, 0.5250000000000000222, 0.5374999999999999778, 0.5500000000000000444, 0.5625000000000000000, 0.5749999999999999556, 0.5875000000000000222, 0.5999999999999999778, 0.6125000000000000444, 0.6250000000000000000, 0.6374999999999999556, 0.6500000000000000222, 0.6624999999999999778, 0.6750000000000000444, 0.6875000000000000000, 0.6999999999999999556, 0.7125000000000000222, 0.7249999999999999778, 0.7375000000000000444, 0.7500000000000000000, 0.7624999999999999556, 0.7750000000000000222, 0.7874999999999999778, 0.8000000000000000444, 0.8125000000000000000, 0.8249999999999999556, 0.8375000000000000222, 0.8499999999999999778, 0.8625000000000000444, 0.8750000000000000000, 0.8874999999999999556, 0.9000000000000000222, 0.9124999999999999778, 0.9250000000000000444, 0.9375000000000000000, 0.9499999999999999556, 0.9625000000000000222, 0.9749999999999999778, 0.9875000000000000444, 1.000000000000000000 ),
 .UNSPECIFIED. ) 
 GEOMETRIC_REPRESENTATION_ITEM ( )  RATIONAL_B_SPLINE_SURFACE ( (
 ( 1.000000000000000000, 0.9238795325112869605, 1.000000000000000000, 0.9238795325112869605, 1.000000000000000000, 0.9238795325112869605, 1.000000000000000000, 0.9238795325112869605, 1.000000000000000000, 0.9238795325112869605, 1.000000000000000000, 0.9238795325112869605, 1.000000000000000000, 0.9238795325112869605, 1.000000000000000000, 0.9238795325112869605, 1.000000000000000000, 0.9238795325112869605, 1.000000000000000000, 0.9238795325112869605, 1.000000000000000000, 0.9238795325112869605, 1.000000000000000000, 0.9238795325112869605, 1.000000000000000000, 0.9238795325112869605, 1.000000000000000000, 0.9238795325112869605, 1.000000000000000000, 0.9238795325112869605, 1.000000000000000000, 0.9238795325112869605, 1.000000000000000000, 0.9238795325112869605, 1.000000000000000000, 0.9238795325112869605, 1.000000000000000000, 0.9238795325112869605, 1.000000000000000000, 0.9238795325112869605, 1.000000000000000000, 0.9238795325112869605, 1.000000000000000000, 0.9238795325112869605, 1.000000000000000000, 0.9238795325112869605, 1.000000000000000000, 0.9238795325112869605, 1.000000000000000000, 0.9238795325112869605, 1.000000000000000000, 0.9238795325112869605, 1.000000000000000000, 0.9238795325112869605, 1.000000000000000000, 0.9238795325112869605, 1.000000000000000000, 0.9238795325112869605, 1.000000000000000000, 0.9238795325112869605, 1.000000000000000000, 0.9238795325112869605, 1.000000000000000000, 0.9238795325112869605, 1.000000000000000000, 0.9238795325112869605, 1.000000000000000000, 0.9238795325112869605, 1.000000000000000000, 0.9238795325112869605, 1.000000000000000000, 0.9238795325112869605, 1.000000000000000000, 0.9238795325112869605, 1.000000000000000000, 0.9238795325112869605, 1.000000000000000000, 0.9238795325112869605, 1.000000000000000000, 0.9238795325112869605, 1.000000000000000000, 0.9238795325112869605, 1.000000000000000000, 0.9238795325112869605, 1.000000000000000000, 0.9238795325112869605, 1.000000000000000000, 0.9238795325112869605, 1.000000000000000000, 0.9238795325112869605, 1.000000000000000000, 0.9238795325112869605, 1.000000000000000000, 0.9238795325112869605, 1.000000000000000000, 0.9238795325112869605, 1.000000000000000000, 0.9238795325112869605, 1.000000000000000000, 0.9238795325112869605, 1.000000000000000000, 0.9238795325112869605, 1.000000000000000000, 0.9238795325112869605, 1.000000000000000000, 0.9238795325112869605, 1.000000000000000000, 0.9238795325112869605, 1.000000000000000000, 0.9238795325112869605, 1.000000000000000000, 0.9238795325112869605, 1.000000000000000000, 0.9238795325112869605, 1.000000000000000000, 0.9238795325112869605, 1.000000000000000000, 0.9238795325112869605, 1.000000000000000000, 0.9238795325112869605, 1.000000000000000000, 0.9238795325112869605, 1.000000000000000000, 0.9238795325112869605, 1.000000000000000000, 0.9238795325112869605, 1.000000000000000000, 0.9238795325112869605, 1.000000000000000000, 0.9238795325112869605, 1.000000000000000000, 0.9238795325112869605, 1.000000000000000000, 0.9238795325112869605, 1.000000000000000000, 0.9238795325112869605, 1.000000000000000000, 0.9238795325112869605, 1.000000000000000000, 0.9238795325112869605, 1.000000000000000000, 0.9238795325112869605, 1.000000000000000000, 0.9238795325112869605, 1.000000000000000000, 0.9238795325112869605, 1.000000000000000000, 0.9238795325112869605, 1.000000000000000000, 0.9238795325112869605, 1.000000000000000000, 0.9238795325112869605, 1.000000000000000000, 0.9238795325112869605, 1.000000000000000000, 0.9238795325112869605, 1.000000000000000000, 0.9238795325112869605, 1.000000000000000000, 0.9238795325112869605, 1.000000000000000000),
 ( 1.000000000000000000, 0.9238795325112869605, 1.000000000000000000, 0.9238795325112869605, 1.000000000000000000, 0.9238795325112869605, 1.000000000000000000, 0.9238795325112869605, 1.000000000000000000, 0.9238795325112869605, 1.000000000000000000, 0.9238795325112869605, 1.000000000000000000, 0.9238795325112869605, 1.000000000000000000, 0.9238795325112869605, 1.000000000000000000, 0.9238795325112869605, 1.000000000000000000, 0.9238795325112869605, 1.000000000000000000, 0.9238795325112869605, 1.000000000000000000, 0.9238795325112869605, 1.000000000000000000, 0.9238795325112869605, 1.000000000000000000, 0.9238795325112869605, 1.000000000000000000, 0.9238795325112869605, 1.000000000000000000, 0.9238795325112869605, 1.000000000000000000, 0.9238795325112869605, 1.000000000000000000, 0.9238795325112869605, 1.000000000000000000, 0.9238795325112869605, 1.000000000000000000, 0.9238795325112869605, 1.000000000000000000, 0.9238795325112869605, 1.000000000000000000, 0.9238795325112869605, 1.000000000000000000, 0.9238795325112869605, 1.000000000000000000, 0.9238795325112869605, 1.000000000000000000, 0.9238795325112869605, 1.000000000000000000, 0.9238795325112869605, 1.000000000000000000, 0.9238795325112869605, 1.000000000000000000, 0.9238795325112869605, 1.000000000000000000, 0.9238795325112869605, 1.000000000000000000, 0.9238795325112869605, 1.000000000000000000, 0.9238795325112869605, 1.000000000000000000, 0.9238795325112869605, 1.000000000000000000, 0.9238795325112869605, 1.000000000000000000, 0.9238795325112869605, 1.000000000000000000, 0.9238795325112869605, 1.000000000000000000, 0.9238795325112869605, 1.000000000000000000, 0.9238795325112869605, 1.000000000000000000, 0.9238795325112869605, 1.000000000000000000, 0.9238795325112869605, 1.000000000000000000, 0.9238795325112869605, 1.000000000000000000, 0.9238795325112869605, 1.000000000000000000, 0.9238795325112869605, 1.000000000000000000, 0.9238795325112869605, 1.000000000000000000, 0.9238795325112869605, 1.000000000000000000, 0.9238795325112869605, 1.000000000000000000, 0.9238795325112869605, 1.000000000000000000, 0.9238795325112869605, 1.000000000000000000, 0.9238795325112869605, 1.000000000000000000, 0.9238795325112869605, 1.000000000000000000, 0.9238795325112869605, 1.000000000000000000, 0.9238795325112869605, 1.000000000000000000, 0.9238795325112869605, 1.000000000000000000, 0.9238795325112869605, 1.000000000000000000, 0.9238795325112869605, 1.000000000000000000, 0.9238795325112869605, 1.000000000000000000, 0.9238795325112869605, 1.000000000000000000, 0.9238795325112869605, 1.000000000000000000, 0.9238795325112869605, 1.000000000000000000, 0.9238795325112869605, 1.000000000000000000, 0.9238795325112869605, 1.000000000000000000, 0.9238795325112869605, 1.000000000000000000, 0.9238795325112869605, 1.000000000000000000, 0.9238795325112869605, 1.000000000000000000, 0.9238795325112869605, 1.000000000000000000, 0.9238795325112869605, 1.000000000000000000, 0.9238795325112869605, 1.000000000000000000, 0.9238795325112869605, 1.000000000000000000, 0.9238795325112869605, 1.000000000000000000, 0.9238795325112869605, 1.000000000000000000, 0.9238795325112869605, 1.000000000000000000, 0.9238795325112869605, 1.000000000000000000, 0.9238795325112869605, 1.000000000000000000, 0.9238795325112869605, 1.000000000000000000, 0.9238795325112869605, 1.000000000000000000, 0.9238795325112869605, 1.000000000000000000, 0.9238795325112869605, 1.000000000000000000, 0.9238795325112869605, 1.000000000000000000, 0.9238795325112869605, 1.000000000000000000, 0.9238795325112869605, 1.000000000000000000, 0.9238795325112869605, 1.000000000000000000) ) ) 
 REPRESENTATION_ITEM ( '' )  SURFACE ( )  );
#34017=CARTESIAN_POINT ( 'NONE',  ( 117.2294421295247844, -4.863998795839590272, -7.758215200338314688 ) ) ;
#34019=CARTESIAN_POINT ( 'NONE',  ( 109.5102233795247884, -8.938348069036489818, -17.46756447353520159 ) ) ;
#34020=CARTESIAN_POINT ( 'NONE',  ( 111.9410827545248708, -6.936859964151250502, -8.388885654883777576 ) ) ;
#34021=CARTESIAN_POINT ( 'NONE',  ( 107.9822546295247889, -4.863998795839590272, -7.631215200338315796 ) ) ;
#34022=VECTOR ( 'NONE', #8382, 999.9999999999998863 ) ;
#34038=CARTESIAN_POINT ( 'NONE',  ( 108.8851452545248151, -9.868328341294098749, -15.46607636864997204 ) ) ;
#34039=CARTESIAN_POINT ( 'NONE',  ( 110.5520202545248054, 0.1403307496149616695, -11.32035403202665336 ) ) ;
#34055=VECTOR ( 'NONE', #14502, 1000.000000000000114 ) ;
#34057=CARTESIAN_POINT ( 'NONE',  ( 66.38809756183205479, -36.79083284667497367, -4.893215200338314474 ) ) ;
#34060=CARTESIAN_POINT ( 'NONE',  ( 67.69189222814998175, -49.76310523276723785, -40.89321520033831092 ) ) ;
#34062=CARTESIAN_POINT ( 'NONE',  ( 108.0517077545248696, -2.791137627527939813, -18.39754474579286025 ) ) ;
#34064=CARTESIAN_POINT ( 'NONE',  ( 115.6220983795247861, -8.402594152722633325, -16.93181055722144990 ) ) ;
#34068=ORIENTED_EDGE ( 'NONE', *, *, #20999, .T. ) ;
#34077=ORIENTED_EDGE ( 'NONE', *, *, #39257, .F. ) ;
#34080=CARTESIAN_POINT ( 'NONE',  ( 107.3571765045248299, -2.791137627527939813, -8.388885654883777576 ) ) ;
#34084=CARTESIAN_POINT ( 'NONE',  ( 106.1070202545248407, -10.62599879583958717, -15.77991374673208469 ) ) ;
#34085=CARTESIAN_POINT ( 'NONE',  ( 111.0762212410415799, 0.7607806665037644134, -12.14321520033829316 ) ) ;
#34089=VECTOR ( 'NONE', #40327, 1000.000000000000000 ) ;
#34091=CARTESIAN_POINT ( 'NONE',  ( 114.4413952545248350, 0.8980012041604421569, -11.00651665394454071 ) ) ;
#34094=CARTESIAN_POINT ( 'NONE',  ( 111.5497331777918788, -0.01829820670803256055, -14.64321520033831447 ) ) ;
#34107=CARTESIAN_POINT ( 'NONE',  ( 111.8021765045248372, -2.791137627527939813, -8.388885654883777576 ) ) ;
#34110=CARTESIAN_POINT ( 'NONE',  ( 114.0941296295247867, -4.863998795839590272, -19.15521520033831493 ) ) ;
#34115=CARTESIAN_POINT ( 'NONE',  ( 85.56953267055843071, -21.30583187727814121, -4.893215200338314474 ) ) ;
#34117=ADVANCED_FACE ( 'NONE', ( #43680 ), #16092, .F. ) ;
#34118=CARTESIAN_POINT ( 'NONE',  ( 116.4360542988829081, 2.232332096932356791, -6.377660291141232562 ) ) ;
#34120=CARTESIAN_POINT ( 'NONE',  ( 105.9681140045248355, 0.1403307496149616695, -15.46607636864997204 ) ) ;
#34134=CARTESIAN_POINT ( 'NONE',  ( 109.7880358795247986, -0.7896495226426338832, -17.46756447353520159 ) ) ;
#34135=CARTESIAN_POINT ( 'NONE',  ( 79.79010115959992788, 5.106172230548759572, -6.893215200338315363 ) ) ;
#34136=CARTESIAN_POINT ( 'NONE',  ( 83.01822478718537468, -31.84465705650555734, -23.29249428169273628 ) ) ;
#34140=CARTESIAN_POINT ( 'NONE',  ( 112.0799890045248475, -9.868328341294098749, -11.32035403202665869 ) ) ;
#34147=ORIENTED_EDGE ( 'NONE', *, *, #9440, .F. ) ;
#34148=CARTESIAN_POINT ( 'NONE',  ( 63.69189222814998175, -80.85404093559408523, -31.07034979220001603 ) ) ;
#34149=CARTESIAN_POINT ( 'NONE',  ( 116.8074716117156413, -11.72235701766462057, -21.41449971386014184 ) ) ;
#34158=CARTESIAN_POINT ( 'NONE',  ( 109.1629577545248395, -2.791137627527939813, -18.39754474579286025 ) ) ;
#34160=CARTESIAN_POINT ( 'NONE',  ( 65.82164714941100669, 4.169909004287361221, -19.39321520033831447 ) ) ;
#34163=DIRECTION ( 'NONE',  ( 0.9387755102040806765, -0.3445294493088623122, 0.000000000000000000 ) ) ;
#34165=VERTEX_POINT ( 'NONE', #11777 ) ;
#34169=CARTESIAN_POINT ( 'NONE',  ( 78.19609438264805590, -57.93615991906383300, -0.7640671700936263466 ) ) ;
#34177=VECTOR ( 'NONE', #40831, 1000.000000000000114 ) ;
#34184=EDGE_CURVE ( 'NONE', #7030, #14703, #24536, .T. ) ;
#34185=CARTESIAN_POINT ( 'NONE',  ( 105.4819421295248247, 0.8980012041604618078, -13.39321520033831447 ) ) ;
#34186=CARTESIAN_POINT ( 'NONE',  ( 106.3848327545248651, -6.936859964151250502, -8.388885654883777576 ) ) ;
#34187=CARTESIAN_POINT ( 'NONE',  ( 105.1346765045248475, -2.791137627527939813, -8.388885654883777576 ) ) ;
#34188=CARTESIAN_POINT ( 'NONE',  ( 64.40114967617560637, -36.78199758899061322, -5.510037480650538555 ) ) ;
#34191=CARTESIAN_POINT ( 'NONE',  ( 61.69189222814998175, -48.76310523276723785, -23.89321520033831803 ) ) ;
#34196=CARTESIAN_POINT ( 'NONE',  ( 106.8015515045248378, -2.477300249445798297, -7.631215200338321125 ) ) ;
#34198=ORIENTED_EDGE ( 'NONE', *, *, #37471, .F. ) ;
#34199=CARTESIAN_POINT ( 'NONE',  ( 143.3676850761856940, -69.76310523276724496, -16.89321520033831447 ) ) ;
#34206=CARTESIAN_POINT ( 'NONE',  ( 107.2294421295247844, -9.051693226400931991, -21.39321520033831447 ) ) ;
#34210=EDGE_CURVE ( 'NONE', #23154, #6107, #32725, .T. ) ;
#34219=CARTESIAN_POINT ( 'NONE',  ( 110.2742077545248094, -7.250697342233347165, -7.631215200338321125 ) ) ;
#34228=CARTESIAN_POINT ( 'NONE',  ( 61.69189222814998175, -69.76310523276724496, -32.79321520033831661 ) ) ;
#34231=CARTESIAN_POINT ( 'NONE',  ( 109.2294421295247844, 0.8460904216231607267, -19.39321520033831447 ) ) ;
#34243=CARTESIAN_POINT ( 'NONE',  ( 108.7462390045248242, 0.8980012041604421569, -15.77991374673208469 ) ) ;
#34244=CARTESIAN_POINT ( 'NONE',  ( 114.5108483795247878, -8.402594152722688392, -16.93181055722141792 ) ) ;
#34245=CARTESIAN_POINT ( 'NONE',  ( 107.2877233795247776, -8.938348069036489818, -17.46756447353520159 ) ) ;
#34258=CARTESIAN_POINT ( 'NONE',  ( 107.0099108795247815, -8.938348069036489818, -9.318865927141430916 ) ) ;
#34263=CARTESIAN_POINT ( 'NONE',  ( 106.1764733795248219, -1.325403438956436419, -9.854619843455211026 ) ) ;
#34264=CARTESIAN_POINT ( 'NONE',  ( 105.8292077545248446, -2.791137627527939813, -18.39754474579286025 ) ) ;
#34286=CARTESIAN_POINT ( 'NONE',  ( 114.3024890045248156, 0.8980012041604421569, -15.77991374673208469 ) ) ;
#34294=CARTESIAN_POINT ( 'NONE',  ( 69.69189222814998175, -41.76310523276723785, -20.39321520033831447 ) ) ;
#34295=CARTESIAN_POINT ( 'NONE',  ( 112.4272546295247821, -4.863998795839590272, -7.631215200338315796 ) ) ;
#34297=CARTESIAN_POINT ( 'NONE',  ( 65.15858969855669613, -37.34466124008154253, -5.220056341859305782 ) ) ;
#34303=CARTESIAN_POINT ( 'NONE',  ( 115.4137390045248566, 0.8980012041604421569, -15.77991374673208469 ) ) ;
#34308=CARTESIAN_POINT ( 'NONE',  ( 105.8292077545248446, -7.250697342233347165, -7.631215200338321125 ) ) ;
#34310=CARTESIAN_POINT ( 'NONE',  ( 63.02947104699595116, -32.17731879514034432, -23.89321520033831447 ) ) ;
#34311=AXIS2_PLACEMENT_3D ( 'NONE', #17118, #23961, #27818 ) ;
#34312=CARTESIAN_POINT ( 'NONE',  ( 108.1211608795247798, -8.938348069036489818, -9.318865927141430916 ) ) ;
#34314=CARTESIAN_POINT ( 'NONE',  ( 112.1494421295248003, 0.8980012041604618078, -13.39321520033831447 ) ) ;
#34332=CARTESIAN_POINT ( 'NONE',  ( 116.8308172556448596, -1.389150239195028114, -17.31318354165465578 ) ) ;
#34333=CARTESIAN_POINT ( 'NONE',  ( 114.4413952545248350, 0.8980012041604421569, -11.00651665394454071 ) ) ;
#34339=CARTESIAN_POINT ( 'NONE',  ( 116.4392337193178975, 2.230983512441839345, -6.373539596108586558 ) ) ;
#34340=CARTESIAN_POINT ( 'NONE',  ( 61.69189222814998175, -40.21211973637273474, -23.89321520033831803 ) ) ;
#34341=CARTESIAN_POINT ( 'NONE',  ( 108.6073327545248048, -6.936859964151250502, -8.388885654883777576 ) ) ;
#34354=CARTESIAN_POINT ( 'NONE',  ( 110.0658483795247804, -0.7896495226426338832, -9.318865927141430916 ) ) ;
#34355=CARTESIAN_POINT ( 'NONE',  ( 106.3848327545248651, -6.936859964151250502, -8.388885654883777576 ) ) ;
#34356=CARTESIAN_POINT ( 'NONE',  ( 115.3442858795247759, -0.7896495226426338832, -17.46756447353520159 ) ) ;
#34359=CARTESIAN_POINT ( 'NONE',  ( 109.2294426289140858, -7.739168762018897141, -8.465928987177235854 ) ) ;
#34361=CARTESIAN_POINT ( 'NONE',  ( 110.2742077545248094, -2.791137627527939813, -18.39754474579286025 ) ) ;
#34369=CARTESIAN_POINT ( 'NONE',  ( 113.6774108795247997, -8.938348069036441856, -9.318865927141430916 ) ) ;
#34374=ADVANCED_FACE ( 'NONE', ( #32506 ), #32945, .F. ) ;
#34379=CARTESIAN_POINT ( 'NONE',  ( 116.4555358795247884, -0.7896495226426338832, -17.46756447353520159 ) ) ;
#34381=CARTESIAN_POINT ( 'NONE',  ( 115.9294421295247872, 1.035107641088057973, -12.14321520033831625 ) ) ;
#34396=FACE_BOUND ( 'NONE', #32169, .T. ) ;
#34404=CARTESIAN_POINT ( 'NONE',  ( 105.9681140045248355, -10.62599879583958717, -11.00651665394454604 ) ) ;
#34405=CARTESIAN_POINT ( 'NONE',  ( 106.4542858795248179, -8.402594152722688392, -9.854619843455216355 ) ) ;
#34408=CARTESIAN_POINT ( 'NONE',  ( 64.08498584890432426, -35.21828807897666991, -5.893215200338318915 ) ) ;
#34411=DIRECTION ( 'NONE',  ( 0.000000000000000000, 0.000000000000000000, 1.000000000000000000 ) ) ;
#34415=CARTESIAN_POINT ( 'NONE',  ( 107.7738952545248310, 0.8980012041604421569, -11.00651665394454071 ) ) ;
#34433=ORIENTED_EDGE ( 'NONE', *, *, #40083, .F. ) ;
#34437=CARTESIAN_POINT ( 'NONE',  ( 109.8574890045247940, 0.8980012041604421569, -15.77991374673208469 ) ) ;
#34439=ORIENTED_EDGE ( 'NONE', *, *, #6657, .T. ) ;
#34451=CARTESIAN_POINT ( 'NONE',  ( 68.92755183904094451, -25.82220866885473853, -5.893215200338315363 ) ) ;
#34458=CARTESIAN_POINT ( 'NONE',  ( 106.3153796295248412, -4.863998795839590272, -19.15521520033831493 ) ) ;
#34459=CARTESIAN_POINT ( 'NONE',  ( 107.1488171295247867, 0.1403307496149613920, -13.39321520033831447 ) ) ;
#34460=CARTESIAN_POINT ( 'NONE',  ( 106.1070202545248407, -10.62599879583958717, -15.77991374673208469 ) ) ;
#34465=CARTESIAN_POINT ( 'NONE',  ( 113.0523327545247838, -2.477300249445798297, -19.15521520033831138 ) ) ;
#34468=PLANE ( 'NONE',  #21148 ) ;
#34472=CARTESIAN_POINT ( 'NONE',  ( 107.2877233795247776, -8.938348069036489818, -17.46756447353520159 ) ) ;
#34474=CIRCLE ( 'NONE', #39564, 7.132259260909268761 ) ;
#34478=CARTESIAN_POINT ( 'NONE',  ( 107.2182702545248105, 0.1403307496149616695, -11.32035403202665336 ) ) ;
#34479=CARTESIAN_POINT ( 'NONE',  ( 105.8986608795248401, -1.325403438956436419, -16.93181055722141792 ) ) ;
#34483=VERTEX_POINT ( 'NONE', #27491 ) ;
#34492=EDGE_CURVE ( 'NONE', #3445, #27212, #1206, .T. ) ;
#34493=ORIENTED_EDGE ( 'NONE', *, *, #12568, .F. ) ;
#34498=ORIENTED_EDGE ( 'NONE', *, *, #26557, .T. ) ;
#34502=CARTESIAN_POINT ( 'NONE',  ( 113.6774108795247997, -8.938348069036489818, -9.318865927141430916 ) ) ;
#34503=CARTESIAN_POINT ( 'NONE',  ( 115.7610046295247912, -4.863998795839541422, -18.39754474579285315 ) ) ;
#34512=CARTESIAN_POINT ( 'NONE',  ( 113.1217858795247935, -0.7896495226426338832, -17.46756447353520159 ) ) ;
#34514=CARTESIAN_POINT ( 'NONE',  ( 64.85279889734272274, -37.42711610596241911, -5.218367175100045330 ) ) ;
#34520=CARTESIAN_POINT ( 'NONE',  ( 116.3860827545247787, -2.477300249445798297, -19.15521520033831138 ) ) ;
#34525=CARTESIAN_POINT ( 'NONE',  ( 109.8574890045248509, -9.868328341294098749, -11.32035403202665869 ) ) ;
#34531=CARTESIAN_POINT ( 'NONE',  ( 109.7185827545247889, -2.477300249445798297, -19.15521520033831138 ) ) ;
#34534=CARTESIAN_POINT ( 'NONE',  ( 111.8698066399283704, 0.4261359969231631739, -14.64321520033831447 ) ) ;
#34537=VERTEX_POINT ( 'NONE', #37045 ) ;
#34548=CARTESIAN_POINT ( 'NONE',  ( 116.8699474989354741, -0.1023020899842886217, -15.73832783096735355 ) ) ;
#34549=CARTESIAN_POINT ( 'NONE',  ( 115.2053796295247849, -4.863998795839590272, -19.15521520033831493 ) ) ;
#34550=VERTEX_POINT ( 'NONE', #23390 ) ;
#34560=CARTESIAN_POINT ( 'NONE',  ( 111.3123452706805807, 0.3193521225029610777, -14.64321520033833757 ) ) ;
#34561=CARTESIAN_POINT ( 'NONE',  ( 115.1359265045248605, -2.791137627527939813, -8.388885654883777576 ) ) ;
#34571=CARTESIAN_POINT ( 'NONE',  ( 116.8722546295247895, -4.863998795839590272, -18.39754474579285315 ) ) ;
#34574=CARTESIAN_POINT ( 'NONE',  ( 111.2465515045248168, -2.477300249445798297, -7.631215200338321125 ) ) ;
#34575=CARTESIAN_POINT ( 'NONE',  ( 61.76986277844709861, -39.32091226840162079, -6.340220811149025693 ) ) ;
#34576=CARTESIAN_POINT ( 'NONE',  ( 112.2883483795247770, -0.7896495226426338832, -9.318865927141430916 ) ) ;
#34582=CARTESIAN_POINT ( 'NONE',  ( 110.1353015045248469, -6.936859964151250502, -18.39754474579286025 ) ) ;
#34588=CARTESIAN_POINT ( 'NONE',  ( 113.4690515045247992, -2.477300249445798297, -7.631215200338321125 ) ) ;
#34598=CARTESIAN_POINT ( 'NONE',  ( 107.9128015045248219, -6.936859964151250502, -18.39754474579286025 ) ) ;
#34607=CARTESIAN_POINT ( 'NONE',  ( 115.6220983795247861, -0.7896495226426338832, -9.318865927141430916 ) ) ;
#34616=CYLINDRICAL_SURFACE ( 'NONE', #7732, 5.999999999999998224 ) ;
#34624=CARTESIAN_POINT ( 'NONE',  ( 108.2600671295247992, -10.62599879583958540, -13.39321520033831447 ) ) ;
#34625=CARTESIAN_POINT ( 'NONE',  ( 107.7044421295247929, -9.868328341294093420, -13.39321520033831447 ) ) ;
#34626=CARTESIAN_POINT ( 'NONE',  ( 106.7320983795247855, -8.402594152722688392, -16.93181055722141792 ) ) ;
#34627=CARTESIAN_POINT ( 'NONE',  ( 113.8604010812576774, -0.01829820670803256055, -12.14321520033831625 ) ) ;
#34636=CARTESIAN_POINT ( 'NONE',  ( 113.4690515045247992, -6.936859964151250502, -18.39754474579286025 ) ) ;
#34638=EDGE_LOOP ( 'NONE', ( #43366, #1324, #16754, #24643 ) ) ;
#34643=CARTESIAN_POINT ( 'NONE',  ( 61.69189222814998175, -56.75720911921465728, -38.40793382609975737 ) ) ;
#34653=ORIENTED_EDGE ( 'NONE', *, *, #34004, .F. ) ;
#34657=CARTESIAN_POINT ( 'NONE',  ( 107.0099108795247815, -8.938348069036489818, -9.318865927141430916 ) ) ;
#34659=VERTEX_POINT ( 'NONE', #27037 ) ;
#34668=EDGE_CURVE ( 'NONE', #7297, #30491, #42575, .T. ) ;
#34673=DIRECTION ( 'NONE',  ( 1.000000000000000000, 0.000000000000000000, 0.000000000000000000 ) ) ;
#34675=VERTEX_POINT ( 'NONE', #39980 ) ;
#34677=CARTESIAN_POINT ( 'NONE',  ( 116.0861162244890892, -0.02276961308034231024, -12.14321520033833934 ) ) ;
#34678=CARTESIAN_POINT ( 'NONE',  ( 108.9545983795247821, -0.7896495226426338832, -9.318865927141430916 ) ) ;
#34679=CARTESIAN_POINT ( 'NONE',  ( 108.0517077545248696, -2.791137627527939813, -18.39754474579286025 ) ) ;
#34680=CARTESIAN_POINT ( 'NONE',  ( 107.0099108795247815, -8.938348069036489818, -9.318865927141430916 ) ) ;
#34684=CARTESIAN_POINT ( 'NONE',  ( 112.9134265045247645, -7.250697342233347165, -19.15521520033831138 ) ) ;
#34685=LINE ( 'NONE', #38553, #14668 ) ;
#34688=DIRECTION ( 'NONE',  ( 0.000000000000000000, 0.9284778069183720062, 0.3713878862591650232 ) ) ;
#34691=CARTESIAN_POINT ( 'NONE',  ( 107.4960827545248350, -2.477300249445798297, -19.15521520033831138 ) ) ;
#34693=DIRECTION ( 'NONE',  ( 1.000000000000000000, 0.000000000000000000, 0.000000000000000000 ) ) ;
#34697=CARTESIAN_POINT ( 'NONE',  ( 113.8163171295247764, -10.62599879583958540, -13.39321520033831447 ) ) ;
#34698=CARTESIAN_POINT ( 'NONE',  ( 106.2459265045248173, -2.791137627527939813, -8.388885654883777576 ) ) ;
#34702=ORIENTED_EDGE ( 'NONE', *, *, #40774, .T. ) ;
#34712=B_SPLINE_CURVE_WITH_KNOTS ( 'NONE', 3,
 ( #15469, #15240, #29148, #43061 ),
 .UNSPECIFIED., .F., .F.,
 ( 4, 4 ),
 ( 0.000000000000000000, 1.000000000000000000 ),
 .UNSPECIFIED. ) ;
#34716=EDGE_LOOP ( 'NONE', ( #13547, #32608, #33382, #26776 ) ) ;
#34719=CARTESIAN_POINT ( 'NONE',  ( 114.7192077545248594, -7.250697342233347165, -7.631215200338321125 ) ) ;
#34729=CARTESIAN_POINT ( 'NONE',  ( 64.01282776924008999, -34.86145050234443943, -5.893215200338315363 ) ) ;
#34734=CARTESIAN_POINT ( 'NONE',  ( 61.69189222814998175, -49.76310523276723785, -19.39321520033831447 ) ) ;
#34735=CARTESIAN_POINT ( 'NONE',  ( 106.1764733795248219, -1.325403438956436419, -9.854619843455211026 ) ) ;
#34741=CARTESIAN_POINT ( 'NONE',  ( 112.2883483795247770, -8.402594152722633325, -16.93181055722145345 ) ) ;
#34742=CARTESIAN_POINT ( 'NONE',  ( 108.9545983795247821, -8.402594152722688392, -16.93181055722141792 ) ) ;
#34744=CARTESIAN_POINT ( 'NONE',  ( 109.2294549733054652, -7.062974527347291698, -18.20822852925657998 ) ) ;
#34746=CARTESIAN_POINT ( 'NONE',  ( 61.58853448128274266, 6.499901296646661386, -12.14321520033831625 ) ) ;
#34747=CARTESIAN_POINT ( 'NONE',  ( 116.1082702545247827, 0.1403307496149616695, -11.32035403202665336 ) ) ;
#34748=CARTESIAN_POINT ( 'NONE',  ( 109.4407702545248355, -10.62599879583958717, -15.77991374673208469 ) ) ;
#34760=ORIENTED_EDGE ( 'NONE', *, *, #41032, .T. ) ;
#34767=CARTESIAN_POINT ( 'NONE',  ( 113.5385046295247804, -4.863998795839590272, -7.631215200338315796 ) ) ;
#34769=LINE ( 'NONE', #6983, #10415 ) ;
#34777=CARTESIAN_POINT ( 'NONE',  ( 113.7468640045248236, 0.1403307496149616695, -15.46607636864997204 ) ) ;
#34787=CARTESIAN_POINT ( 'NONE',  ( 117.2294421295247844, 1.035107641088057973, -12.14321520033831625 ) ) ;
#34791=DIRECTION ( 'NONE',  ( 0.000000000000000000, 0.000000000000000000, 1.000000000000000000 ) ) ;
#34792=CARTESIAN_POINT ( 'NONE',  ( 113.6079577545248043, -7.250697342233347165, -7.631215200338321125 ) ) ;
#34795=CARTESIAN_POINT ( 'NONE',  ( 109.2294886045864502, -1.390863055952577865, -9.246587650953511428 ) ) ;
#34797=CARTESIAN_POINT ( 'NONE',  ( 107.2182702545248105, 0.1403307496149616695, -11.32035403202665336 ) ) ;
#34801=CARTESIAN_POINT ( 'NONE',  ( 109.3018640045248304, -10.62599879583958717, -11.00651665394454604 ) ) ;
#34811=CARTESIAN_POINT ( 'NONE',  ( 108.8851452545248151, -9.868328341294098749, -15.46607636864997204 ) ) ;
#34815=ORIENTED_EDGE ( 'NONE', *, *, #22524, .T. ) ;
#34821=CARTESIAN_POINT ( 'NONE',  ( 114.0246765045248196, -7.250697342233347165, -19.15521520033831138 ) ) ;
#34829=DIRECTION ( 'NONE',  ( 0.000000000000000000, 0.000000000000000000, -1.000000000000000000 ) ) ;
#34837=CARTESIAN_POINT ( 'NONE',  ( 108.6073327545248048, -2.477300249445798297, -19.15521520033831138 ) ) ;
#34849=CARTESIAN_POINT ( 'NONE',  ( 112.2883483795247770, -8.402594152722688392, -16.93181055722141792 ) ) ;
#34856=LINE ( 'NONE', #3642, #23405 ) ;
#34860=EDGE_LOOP ( 'NONE', ( #43933, #7496, #5859, #38489 ) ) ;
#34863=EDGE_CURVE ( 'NONE', #43791, #44074, #29656, .T. ) ;
#34868=CARTESIAN_POINT ( 'NONE',  ( 106.1070202545248407, -10.62599879583958717, -15.77991374673208469 ) ) ;
#34870=ORIENTED_EDGE ( 'NONE', *, *, #37683, .F. ) ;
#34877=DIRECTION ( 'NONE',  ( 0.000000000000000000, 0.000000000000000000, -1.000000000000000000 ) ) ;
#34889=CARTESIAN_POINT ( 'NONE',  ( 105.9681140045248355, -10.62599879583958717, -11.00651665394454604 ) ) ;
#34890=CARTESIAN_POINT ( 'NONE',  ( 109.4407702545248355, 0.1403307496149616695, -11.32035403202665336 ) ) ;
#34891=CARTESIAN_POINT ( 'NONE',  ( 109.5796765045248122, -7.250697342233347165, -19.15521520033831138 ) ) ;
#34896=CARTESIAN_POINT ( 'NONE',  ( 111.6632702545248605, -10.62599879583958717, -15.77991374673208469 ) ) ;
#34897=FACE_OUTER_BOUND ( 'NONE', #31196, .T. ) ;
#34902=CARTESIAN_POINT ( 'NONE',  ( 116.5249890045247980, 0.8980012041604421569, -15.77991374673208469 ) ) ;
#34903=CARTESIAN_POINT ( 'NONE',  ( 106.7320983795247855, -0.7896495226426338832, -9.318865927141430916 ) ) ;
#34904=EDGE_LOOP ( 'NONE', ( #1847, #33555, #16944, #3925 ) ) ;
#34909=CARTESIAN_POINT ( 'NONE',  ( 113.6079577545248043, -7.250697342233347165, -7.631215200338321125 ) ) ;
#34910=CARTESIAN_POINT ( 'NONE',  ( 105.9681140045248355, 0.1403307496149616695, -15.46607636864997204 ) ) ;
#34914=ORIENTED_EDGE ( 'NONE', *, *, #20999, .F. ) ;
#34920=EDGE_LOOP ( 'NONE', ( #15260, #37358, #25339, #41171, #27371, #9619, #5652 ) ) ;
#34922=VECTOR ( 'NONE', #25265, 1000.000000000000114 ) ;
#34923=CARTESIAN_POINT ( 'NONE',  ( 77.77634386988383142, 3.254514819260860392, -4.893215200338314474 ) ) ;
#34924=CARTESIAN_POINT ( 'NONE',  ( 109.5102233795247884, -1.325403438956436419, -9.854619843455211026 ) ) ;
#34933=CARTESIAN_POINT ( 'NONE',  ( 116.0388171295248014, -10.62599879583958540, -13.39321520033831447 ) ) ;
#34934=AXIS2_PLACEMENT_3D ( 'NONE', #13688, #10266, #10929 ) ;
#34943=CARTESIAN_POINT ( 'NONE',  ( 65.06330879403716949, -35.71473443186641816, -5.721420406450495655 ) ) ;
#34944=CARTESIAN_POINT ( 'NONE',  ( 79.00611218289952831, -44.99489077589586827, -23.89321520033831803 ) ) ;
#34946=VERTEX_POINT ( 'NONE', #30112 ) ;
#34947=VECTOR ( 'NONE', #2090, 1000.000000000000000 ) ;
#34949=CARTESIAN_POINT ( 'NONE',  ( 112.9828796295247884, -4.863998795839590272, -19.15521520033831493 ) ) ;
#34954=CARTESIAN_POINT ( 'NONE',  ( 112.1494421295248003, -9.868328341294093420, -13.39321520033831447 ) ) ;
#34956=CARTESIAN_POINT ( 'NONE',  ( 109.2295631630446593, -8.625464214188930612, -17.23631248896216661 ) ) ;
#34958=CARTESIAN_POINT ( 'NONE',  ( 107.4960827545248350, -2.477300249445798297, -19.15521520033831138 ) ) ;
#34959=CARTESIAN_POINT ( 'NONE',  ( 114.5803015045248117, -6.936859964151250502, -18.39754474579286025 ) ) ;
#34960=CARTESIAN_POINT ( 'NONE',  ( 110.6909265045248247, -7.250697342233347165, -19.15521520033831138 ) ) ;
#34972=ORIENTED_EDGE ( 'NONE', *, *, #23975, .T. ) ;
#34977=CARTESIAN_POINT ( 'NONE',  ( 112.2188952545247531, 0.8980012041604421569, -11.00651665394454071 ) ) ;
#34981=CARTESIAN_POINT ( 'NONE',  ( 117.0806140045248185, 0.1403307496149616695, -15.46607636864997204 ) ) ;
#34985=DIRECTION ( 'NONE',  ( 0.000000000000000000, 0.000000000000000000, -1.000000000000000000 ) ) ;
#34987=CARTESIAN_POINT ( 'NONE',  ( 115.0664733795247798, -1.325403438956436419, -9.854619843455211026 ) ) ;
#34996=EDGE_LOOP ( 'NONE', ( #6687, #57 ) ) ;
#34999=CARTESIAN_POINT ( 'NONE',  ( 116.5944421295247793, -9.868328341294093420, -13.39321520033831447 ) ) ;
#35001=EDGE_CURVE ( 'NONE', #30513, #20890, #43800, .T. ) ;
#35003=CARTESIAN_POINT ( 'NONE',  ( 85.40866212614237440, -28.66666519958388193, -9.415214268655820007 ) ) ;
#35004=CARTESIAN_POINT ( 'NONE',  ( 110.6909265045248247, -7.250697342233347165, -19.15521520033831138 ) ) ;
#35008=CARTESIAN_POINT ( 'NONE',  ( 115.8998954522301830, 0.1168444861213632779, -14.64321520033831447 ) ) ;
#35009=CARTESIAN_POINT ( 'NONE',  ( 109.2291353395606421, 0.1491742553690190431, -11.67757420713069649 ) ) ;
#35011=CARTESIAN_POINT ( 'NONE',  ( 108.7462390045248242, -9.868328341294098749, -11.32035403202665869 ) ) ;
#35014=CARTESIAN_POINT ( 'NONE',  ( 116.6166916131588351, 2.139222853825150761, -20.64615525626918213 ) ) ;
#35017=CARTESIAN_POINT ( 'NONE',  ( 111.0381921295247878, 0.8980012041604618078, -13.39321520033831447 ) ) ;
#35019=VERTEX_POINT ( 'NONE', #12790 ) ;
#35027=EDGE_CURVE ( 'NONE', #10427, #7998, #9363, .T. ) ;
#35028=CARTESIAN_POINT ( 'NONE',  ( 109.4407702545248355, 0.1403307496149616695, -11.32035403202665336 ) ) ;
#35034=EDGE_CURVE ( 'NONE', #930, #2865, #13016, .T. ) ;
#35035=CARTESIAN_POINT ( 'NONE',  ( 83.16394245587648015, -30.76310523276723785, -20.89321520033831447 ) ) ;
#35036=EDGE_CURVE ( 'NONE', #42739, #7998, #40374, .T. ) ;
#35039=CARTESIAN_POINT ( 'NONE',  ( 106.8710046295248759, -4.863998795839590272, -18.39754474579285315 ) ) ;
#35047=EDGE_CURVE ( 'NONE', #25300, #34550, #20849, .T. ) ;
#35060=CARTESIAN_POINT ( 'NONE',  ( 106.3153796295248412, -4.863998795839590272, -19.15521520033831493 ) ) ;
#35063=CIRCLE ( 'NONE', #44584, 3.000000000000002665 ) ;
#35064=CARTESIAN_POINT ( 'NONE',  ( 113.5886041094426844, 0.3591747506842615789, -12.14321520033833046 ) ) ;
#35069=FACE_OUTER_BOUND ( 'NONE', #19255, .T. ) ;
#35070=CARTESIAN_POINT ( 'NONE',  ( 109.2309317933750634, -1.356617975920010322, -16.96302509418498161 ) ) ;
#35072=CARTESIAN_POINT ( 'NONE',  ( 110.4131140045248287, 0.1403307496149616695, -15.46607636864997204 ) ) ;
#35084=CARTESIAN_POINT ( 'NONE',  ( 63.17554510063945372, -31.34889167039416691, -21.89321520033831092 ) ) ;
#35095=CARTESIAN_POINT ( 'NONE',  ( 108.6767858795247861, -0.7896495226426338832, -17.46756447353520159 ) ) ;
#35101=CARTESIAN_POINT ( 'NONE',  ( 79.52666107723024425, 5.086845235696775269, -20.29072895152215494 ) ) ;
#35108=CARTESIAN_POINT ( 'NONE',  ( 105.2294421295247844, -9.051693226400931991, -21.89321520033831447 ) ) ;
#35116=CARTESIAN_POINT ( 'NONE',  ( 116.0842780030094872, -0.02021311778663964498, -12.14321520033831625 ) ) ;
#35117=CARTESIAN_POINT ( 'NONE',  ( 105.8292077545248446, -7.250697342233347165, -7.631215200338321125 ) ) ;
#35118=CARTESIAN_POINT ( 'NONE',  ( 110.0658483795247804, -8.402594152722688392, -16.93181055722141792 ) ) ;
#35119=CARTESIAN_POINT ( 'NONE',  ( 115.0664733795247798, -1.325403438956436419, -9.854619843455211026 ) ) ;
#35122=EDGE_LOOP ( 'NONE', ( #33546, #6171, #1957, #12141 ) ) ;
#35124=CARTESIAN_POINT ( 'NONE',  ( 113.8163171295247764, -10.62599879583958540, -13.39321520033831447 ) ) ;
#35125=CARTESIAN_POINT ( 'NONE',  ( 61.73532138647689038, -39.51680623670656445, -6.460275505913305238 ) ) ;
#35132=CARTESIAN_POINT ( 'NONE',  ( 114.0246765045248196, -7.250697342233347165, -19.15521520033831138 ) ) ;
#35133=CARTESIAN_POINT ( 'NONE',  ( 114.4413952545248350, -9.868328341294098749, -15.46607636864997204 ) ) ;
#35135=CYLINDRICAL_SURFACE ( 'NONE', #7761, 0.8718221387495478369 ) ;
#35140=CARTESIAN_POINT ( 'NONE',  ( 114.0941296295247867, -4.863998795839590272, -19.15521520033831493 ) ) ;
#35154=CARTESIAN_POINT ( 'NONE',  ( 112.4967077545247633, -2.791137627527939813, -18.39754474579286025 ) ) ;
#35159=EDGE_CURVE ( 'NONE', #4412, #11942, #2430, .T. ) ;
#35163=CARTESIAN_POINT ( 'NONE',  ( 83.82415148905927538, -46.76310523276723785, -6.893215200338315363 ) ) ;
#35165=CARTESIAN_POINT ( 'NONE',  ( 106.3848327545248651, -6.936859964151250502, -8.388885654883777576 ) ) ;
#35173=CARTESIAN_POINT ( 'NONE',  ( 116.5249890045247980, 0.8980012041604421569, -15.77991374673208469 ) ) ;
#35174=CARTESIAN_POINT ( 'NONE',  ( 85.02738910321417620, -28.58808629434043524, -8.794714412758365185 ) ) ;
#35175=CARTESIAN_POINT ( 'NONE',  ( 116.3860827545247787, -2.477300249445798297, -19.15521520033831138 ) ) ;
#35181=CARTESIAN_POINT ( 'NONE',  ( 112.7745202545247878, -10.62599879583958717, -15.77991374673208469 ) ) ;
#35184=DIRECTION ( 'NONE',  ( 0.000000000000000000, -1.000000000000000000, 0.000000000000000000 ) ) ;
#35186=CARTESIAN_POINT ( 'NONE',  ( 111.3854577545248645, -2.791137627527939813, -18.39754474579286025 ) ) ;
#35190=CARTESIAN_POINT ( 'NONE',  ( 109.2294493580808989, -5.173074444957243223, -18.58748577876895425 ) ) ;
#35195=CARTESIAN_POINT ( 'NONE',  ( 108.6767858795247861, -0.7896495226426338832, -17.46756447353520159 ) ) ;
#35208=EDGE_CURVE ( 'NONE', #37055, #11127, #40066, .T. ) ;
#35215=CARTESIAN_POINT ( 'NONE',  ( 109.9963952545248134, 0.8980012041604421569, -11.00651665394454071 ) ) ;
#35218=FACE_BOUND ( 'NONE', #43601, .T. ) ;
#35222=CARTESIAN_POINT ( 'NONE',  ( 111.6379010812576809, -0.01829820670803256055, -12.14321520033831625 ) ) ;
#35224=CARTESIAN_POINT ( 'NONE',  ( 116.0388171295248014, 0.1403307496149613920, -13.39321520033831447 ) ) ;
#35234=CARTESIAN_POINT ( 'NONE',  ( 113.8163171295247764, 0.1403307496149613920, -13.39321520033831447 ) ) ;
#35237=CARTESIAN_POINT ( 'NONE',  ( 86.02111790076683917, -27.18318332158748518, -8.573249023392461865 ) ) ;
#35238=CARTESIAN_POINT ( 'NONE',  ( 112.9828796295247884, -4.863998795839590272, -19.15521520033831493 ) ) ;
#35244=CARTESIAN_POINT ( 'NONE',  ( 111.1770983795247787, -8.402594152722688392, -16.93181055722141792 ) ) ;
#35245=CARTESIAN_POINT ( 'NONE',  ( 117.1385944202825442, 1.513614675977436264, -21.43912135226106486 ) ) ;
#35248=CARTESIAN_POINT ( 'NONE',  ( 112.8439733795247832, -8.938348069036489818, -17.46756447353520159 ) ) ;
#35250=ORIENTED_EDGE ( 'NONE', *, *, #32097, .T. ) ;
#35259=CARTESIAN_POINT ( 'NONE',  ( 115.0664733795247798, -8.938348069036489818, -17.46756447353520159 ) ) ;
#35268=CARTESIAN_POINT ( 'NONE',  ( 115.8999108795247821, -8.938348069036489818, -9.318865927141430916 ) ) ;
#35283=CARTESIAN_POINT ( 'NONE',  ( 109.2294421295247844, 0.8460904216231607267, -19.39321520033831447 ) ) ;
#35284=VECTOR ( 'NONE', #17209, 1000.000000000000000 ) ;
#35288=CARTESIAN_POINT ( 'NONE',  ( 114.7192077545248594, -2.791137627527939813, -18.39754474579286025 ) ) ;
#35301=EDGE_CURVE ( 'NONE', #10099, #21089, #25286, .T. ) ;
#35302=CARTESIAN_POINT ( 'NONE',  ( 111.0381921295247878, -9.868328341294093420, -13.39321520033831447 ) ) ;
#35309=DIRECTION ( 'NONE',  ( 0.9970811988817437355, -0.07634843047859309062, -9.125038414728249219E-18 ) ) ;
#35312=CARTESIAN_POINT ( 'NONE',  ( 63.10250807381770244, -31.76310523276724140, -22.30742876271141029 ) ) ;
#35315=ORIENTED_EDGE ( 'NONE', *, *, #41490, .F. ) ;
#35317=CARTESIAN_POINT ( 'NONE',  ( 116.1777233795247781, -1.325403438956436419, -9.854619843455211026 ) ) ;
#35322=DIRECTION ( 'NONE',  ( -1.734723475976807094E-15, -1.000000000000000000, 0.000000000000000000 ) ) ;
#35327=CARTESIAN_POINT ( 'NONE',  ( 108.5378796295247810, -4.863998795839590272, -19.15521520033831493 ) ) ;
#35331=DIRECTION ( 'NONE',  ( 1.000000000000000000, 0.000000000000000000, 0.000000000000000000 ) ) ;
#35333=DIRECTION ( 'NONE',  ( -0.0009519285464165692153, 0.9999995469159186356, 0.000000000000000000 ) ) ;
#35335=DIRECTION ( 'NONE',  ( 0.000000000000000000, 0.000000000000000000, 1.000000000000000000 ) ) ;
#35344=CARTESIAN_POINT ( 'NONE',  ( 112.2883483795247770, -0.7896495226426338832, -9.318865927141420258 ) ) ;
#35347=CARTESIAN_POINT ( 'NONE',  ( 114.0246765045248196, -2.791137627527939813, -8.388885654883777576 ) ) ;
#35348=CARTESIAN_POINT ( 'NONE',  ( 108.8156921295247912, -9.868328341294093420, -13.39321520033831447 ) ) ;
#35349=CARTESIAN_POINT ( 'NONE',  ( 113.3301452545248083, -9.868328341294098749, -15.46607636864997204 ) ) ;
#35352=ORIENTED_EDGE ( 'NONE', *, *, #12095, .F. ) ;
#35354=CARTESIAN_POINT ( 'NONE',  ( 113.7468640045248236, -10.62599879583958717, -11.00651665394454604 ) ) ;
#35362=CARTESIAN_POINT ( 'NONE',  ( 113.9552233795247815, -8.938348069036489818, -17.46756447353520159 ) ) ;
#35363=CARTESIAN_POINT ( 'NONE',  ( 112.4967077545247633, -2.791137627527939813, -18.39754474579286025 ) ) ;
#35377=ORIENTED_EDGE ( 'NONE', *, *, #20311, .T. ) ;
#35380=CARTESIAN_POINT ( 'NONE',  ( 105.4819421295248247, 0.8980012041604618078, -13.39321520033831447 ) ) ;
#35381=CARTESIAN_POINT ( 'NONE',  ( 111.4549108795247747, -1.325403438956436419, -16.93181055722141792 ) ) ;
#35384=VERTEX_POINT ( 'NONE', #34340 ) ;
#35395=CARTESIAN_POINT ( 'NONE',  ( 110.0658483795247804, -0.7896495226426338832, -9.318865927141430916 ) ) ;
#35402=CARTESIAN_POINT ( 'NONE',  ( 116.1082702545247827, -10.62599879583958717, -15.77991374673208469 ) ) ;
#35403=CARTESIAN_POINT ( 'NONE',  ( 66.04840902401572578, -36.51491089899629827, -5.214988841577086198 ) ) ;
#35404=CARTESIAN_POINT ( 'NONE',  ( 116.5944421295247793, 0.8980012041604618078, -13.39321520033831447 ) ) ;
#35409=CARTESIAN_POINT ( 'NONE',  ( 61.69189222814998175, -40.21211973637273474, -4.893215200338314474 ) ) ;
#35410=CARTESIAN_POINT ( 'NONE',  ( 111.8021765045248372, -7.250697342233347165, -19.15521520033831138 ) ) ;
#35415=CARTESIAN_POINT ( 'NONE',  ( 109.0935046295247872, -4.863998795839590272, -18.39754474579285315 ) ) ;
#35417=ORIENTED_EDGE ( 'NONE', *, *, #37729, .F. ) ;
#35419=CARTESIAN_POINT ( 'NONE',  ( 109.2294282733528519, -3.755413602395687445, -18.41110207307550084 ) ) ;
#35422=CARTESIAN_POINT ( 'NONE',  ( 116.2471765045247594, -2.791137627527939813, -8.388885654883777576 ) ) ;
#35423=CARTESIAN_POINT ( 'NONE',  ( 108.1211608795247798, -8.938348069036489818, -9.318865927141430916 ) ) ;
#35440=AXIS2_PLACEMENT_3D ( 'NONE', #22721, #4940, #11799 ) ;
#35441=CARTESIAN_POINT ( 'NONE',  ( 110.9687390045248350, 0.8980012041604421569, -15.77991374673208469 ) ) ;
#35443=CARTESIAN_POINT ( 'NONE',  ( 116.5944421295247793, -9.863109299026486809, -13.29890625629612622 ) ) ;
#35445=CARTESIAN_POINT ( 'NONE',  ( 113.3995983795247895, -8.402594152722688392, -16.93181055722141792 ) ) ;
#35451=CARTESIAN_POINT ( 'NONE',  ( 113.8857702545248003, 0.1403307496149616695, -11.32035403202665336 ) ) ;
#35453=CARTESIAN_POINT ( 'NONE',  ( 114.9716510812576757, -0.01829820670803256055, -12.14321520033831625 ) ) ;
#35455=FACE_BOUND ( 'NONE', #4841, .T. ) ;
#35463=CARTESIAN_POINT ( 'NONE',  ( 112.5661608795247872, -1.325403438956436419, -16.93181055722141792 ) ) ;
#35465=( BOUNDED_SURFACE ( )  B_SPLINE_SURFACE ( 1, 2, ( 
 ( #18692, #22332, #32134, #42862, #29397, #25982, #29168, #11622, #4993, #25533, #42638, #39439, #903, #21435, #35317, #28734, #32794, #11407, #32360, #38979, #28511, #4089, #18471, #11182, #8427, #18011, #35775, #8200, #42416, #22109, #35999, #675, #1568, #32580, #15490, #1350, #43082, #43307, #25757, #39663, #36227, #31910, #7747, #21658, #12529, #16173, #8873, #20046, #33465, #5217, #30522, #19583, #36449, #44223, #19135, #33701, #40797, #2243, #9101, #23002, #22771, #26431, #33018, #30078, #12304, #33248, #36670, #40109, #5441, #2473, #37118, #26203, #12984, #16398, #23469, #2021, #30296, #36895, #1792, #19361, #40337, #15946, #22549, #43992, #44444, #13211, #43763, #9552, #26879, #5664, #29847, #12753, #26654, #37355, #29620, #6127, #40568, #5891, #15718, #9328, #23235, #33929, #19813, #2699, #43535, #16627, #39886, #8649, #24142, #31407, #20719, #35028, #23700, #27110, #6811, #34158, #3811, #24361, #38247, #34811, #10457, #17302, #21154, #14090, #17509, #13656, #31632, #3596, #3160, #174, #7027, #28008, #24581, #34598, #10679, #41915, #38034, #17082, #38465, #7239, #13436, #20498, #3383, #31193, #45113, #23926, #17734, #37589, #6361, #13871, #400, #41033, #9788, #27781, #20272, #41694, #30974, #20939, #10018, #2929, #16858 ),
 ( #30750, #44673, #34379, #27339, #41260, #27563, #37807, #6582, #44898, #41478, #10235, #32309, #24800, #18636, #39153, #8150, #38919, #38691, #22054, #14767, #18852, #21376, #35259, #14316, #32744, #4719, #21603, #43028, #35721, #28901, #28679, #7457, #42138, #32526, #25704, #845, #11344, #21827, #42583, #4035, #11572, #11123, #28232, #1075, #10900, #17957, #35947, #1299, #35490, #31857, #625, #22279, #28453, #7688, #42811, #15211, #14987, #14537, #25479, #25024, #11796, #42362, #39610, #29116, #4263, #18182, #32077, #7917, #39385, #25256, #4494, #8372, #18415, #36172, #4938, #43485, #30018, #33642, #15666, #12932, #12702, #16117, #29567, #1518, #40741, #40286, #6066, #15437, #12254, #33192, #19079, #5611, #5393, #2189, #9049, #22950, #23413, #5163, #26148, #43704, #19312, #37300, #36842, #12024, #22497, #37064, #25926, #15894, #43936, #16343, #40051, #19534, #8598, #8818, #12477, #23186, #26375, #5837, #33410, #9498, #43258, #29345, #26602, #36391, #19986, #40515, #9278, #19761, #2418, #30246, #39835, #44170, #26830, #1968, #32965, #1742, #22719, #36618, #29793, #7580, #31969, #28123, #18074, #24916, #296, #23874, #11015, #21495, #20220, #27288, #10792, #14209, #24689, #30699, #25148, #30469, #44389, #7355, #31526, #37529, #35380 ) ),
 .UNSPECIFIED., .F., .F., .T. ) 
 B_SPLINE_SURFACE_WITH_KNOTS ( ( 2, 2 ),
 ( 3, 2, 2, 2, 2, 2, 2, 2, 2, 2, 2, 2, 2, 2, 2, 2, 2, 2, 2, 2, 2, 2, 2, 2, 2, 2, 2, 2, 2, 2, 2, 2, 2, 2, 2, 2, 2, 2, 2, 2, 2, 2, 2, 2, 2, 2, 2, 2, 2, 2, 2, 2, 2, 2, 2, 2, 2, 2, 2, 2, 2, 2, 2, 2, 2, 2, 2, 2, 2, 2, 2, 2, 2, 2, 2, 2, 2, 2, 2, 2, 3 ),
 ( 0.000000000000000000, 1.000000000000000000 ),
 ( 0.000000000000000000, 0.01250000000000000069, 0.02500000000000000139, 0.03749999999999999861, 0.05000000000000000278, 0.06250000000000000000, 0.07499999999999999722, 0.08749999999999999445, 0.1000000000000000056, 0.1125000000000000028, 0.1250000000000000000, 0.1375000000000000111, 0.1499999999999999944, 0.1625000000000000056, 0.1749999999999999889, 0.1875000000000000000, 0.2000000000000000111, 0.2124999999999999944, 0.2250000000000000056, 0.2374999999999999889, 0.2500000000000000000, 0.2625000000000000111, 0.2750000000000000222, 0.2874999999999999778, 0.2999999999999999889, 0.3125000000000000000, 0.3250000000000000111, 0.3375000000000000222, 0.3499999999999999778, 0.3624999999999999889, 0.3750000000000000000, 0.3875000000000000111, 0.4000000000000000222, 0.4124999999999999778, 0.4249999999999999889, 0.4375000000000000000, 0.4500000000000000111, 0.4625000000000000222, 0.4749999999999999778, 0.4874999999999999889, 0.5000000000000000000, 0.5124999999999999556, 0.5250000000000000222, 0.5374999999999999778, 0.5500000000000000444, 0.5625000000000000000, 0.5749999999999999556, 0.5875000000000000222, 0.5999999999999999778, 0.6125000000000000444, 0.6250000000000000000, 0.6374999999999999556, 0.6500000000000000222, 0.6624999999999999778, 0.6750000000000000444, 0.6875000000000000000, 0.6999999999999999556, 0.7125000000000000222, 0.7249999999999999778, 0.7375000000000000444, 0.7500000000000000000, 0.7624999999999999556, 0.7750000000000000222, 0.7874999999999999778, 0.8000000000000000444, 0.8125000000000000000, 0.8249999999999999556, 0.8375000000000000222, 0.8499999999999999778, 0.8625000000000000444, 0.8750000000000000000, 0.8874999999999999556, 0.9000000000000000222, 0.9124999999999999778, 0.9250000000000000444, 0.9375000000000000000, 0.9499999999999999556, 0.9625000000000000222, 0.9749999999999999778, 0.9875000000000000444, 1.000000000000000000 ),
 .UNSPECIFIED. ) 
 GEOMETRIC_REPRESENTATION_ITEM ( )  RATIONAL_B_SPLINE_SURFACE ( (
 ( 1.000000000000000000, 0.9238795325112869605, 1.000000000000000000, 0.9238795325112869605, 1.000000000000000000, 0.9238795325112869605, 1.000000000000000000, 0.9238795325112869605, 1.000000000000000000, 0.9238795325112869605, 1.000000000000000000, 0.9238795325112869605, 1.000000000000000000, 0.9238795325112869605, 1.000000000000000000, 0.9238795325112869605, 1.000000000000000000, 0.9238795325112869605, 1.000000000000000000, 0.9238795325112869605, 1.000000000000000000, 0.9238795325112869605, 1.000000000000000000, 0.9238795325112869605, 1.000000000000000000, 0.9238795325112869605, 1.000000000000000000, 0.9238795325112869605, 1.000000000000000000, 0.9238795325112869605, 1.000000000000000000, 0.9238795325112869605, 1.000000000000000000, 0.9238795325112869605, 1.000000000000000000, 0.9238795325112869605, 1.000000000000000000, 0.9238795325112869605, 1.000000000000000000, 0.9238795325112869605, 1.000000000000000000, 0.9238795325112869605, 1.000000000000000000, 0.9238795325112869605, 1.000000000000000000, 0.9238795325112869605, 1.000000000000000000, 0.9238795325112869605, 1.000000000000000000, 0.9238795325112869605, 1.000000000000000000, 0.9238795325112869605, 1.000000000000000000, 0.9238795325112869605, 1.000000000000000000, 0.9238795325112869605, 1.000000000000000000, 0.9238795325112869605, 1.000000000000000000, 0.9238795325112869605, 1.000000000000000000, 0.9238795325112869605, 1.000000000000000000, 0.9238795325112869605, 1.000000000000000000, 0.9238795325112869605, 1.000000000000000000, 0.9238795325112869605, 1.000000000000000000, 0.9238795325112869605, 1.000000000000000000, 0.9238795325112869605, 1.000000000000000000, 0.9238795325112869605, 1.000000000000000000, 0.9238795325112869605, 1.000000000000000000, 0.9238795325112869605, 1.000000000000000000, 0.9238795325112869605, 1.000000000000000000, 0.9238795325112869605, 1.000000000000000000, 0.9238795325112869605, 1.000000000000000000, 0.9238795325112869605, 1.000000000000000000, 0.9238795325112869605, 1.000000000000000000, 0.9238795325112869605, 1.000000000000000000, 0.9238795325112869605, 1.000000000000000000, 0.9238795325112869605, 1.000000000000000000, 0.9238795325112869605, 1.000000000000000000, 0.9238795325112869605, 1.000000000000000000, 0.9238795325112869605, 1.000000000000000000, 0.9238795325112869605, 1.000000000000000000, 0.9238795325112869605, 1.000000000000000000, 0.9238795325112869605, 1.000000000000000000, 0.9238795325112869605, 1.000000000000000000, 0.9238795325112869605, 1.000000000000000000, 0.9238795325112869605, 1.000000000000000000, 0.9238795325112869605, 1.000000000000000000, 0.9238795325112869605, 1.000000000000000000, 0.9238795325112869605, 1.000000000000000000, 0.9238795325112869605, 1.000000000000000000, 0.9238795325112869605, 1.000000000000000000, 0.9238795325112869605, 1.000000000000000000, 0.9238795325112869605, 1.000000000000000000, 0.9238795325112869605, 1.000000000000000000, 0.9238795325112869605, 1.000000000000000000, 0.9238795325112869605, 1.000000000000000000, 0.9238795325112869605, 1.000000000000000000, 0.9238795325112869605, 1.000000000000000000, 0.9238795325112869605, 1.000000000000000000, 0.9238795325112869605, 1.000000000000000000, 0.9238795325112869605, 1.000000000000000000, 0.9238795325112869605, 1.000000000000000000, 0.9238795325112869605, 1.000000000000000000, 0.9238795325112869605, 1.000000000000000000, 0.9238795325112869605, 1.000000000000000000, 0.9238795325112869605, 1.000000000000000000, 0.9238795325112869605, 1.000000000000000000, 0.9238795325112869605, 1.000000000000000000, 0.9238795325112869605, 1.000000000000000000, 0.9238795325112869605, 1.000000000000000000),
 ( 1.000000000000000000, 0.9238795325112869605, 1.000000000000000000, 0.9238795325112869605, 1.000000000000000000, 0.9238795325112869605, 1.000000000000000000, 0.9238795325112869605, 1.000000000000000000, 0.9238795325112869605, 1.000000000000000000, 0.9238795325112869605, 1.000000000000000000, 0.9238795325112869605, 1.000000000000000000, 0.9238795325112869605, 1.000000000000000000, 0.9238795325112869605, 1.000000000000000000, 0.9238795325112869605, 1.000000000000000000, 0.9238795325112869605, 1.000000000000000000, 0.9238795325112869605, 1.000000000000000000, 0.9238795325112869605, 1.000000000000000000, 0.9238795325112869605, 1.000000000000000000, 0.9238795325112869605, 1.000000000000000000, 0.9238795325112869605, 1.000000000000000000, 0.9238795325112869605, 1.000000000000000000, 0.9238795325112869605, 1.000000000000000000, 0.9238795325112869605, 1.000000000000000000, 0.9238795325112869605, 1.000000000000000000, 0.9238795325112869605, 1.000000000000000000, 0.9238795325112869605, 1.000000000000000000, 0.9238795325112869605, 1.000000000000000000, 0.9238795325112869605, 1.000000000000000000, 0.9238795325112869605, 1.000000000000000000, 0.9238795325112869605, 1.000000000000000000, 0.9238795325112869605, 1.000000000000000000, 0.9238795325112869605, 1.000000000000000000, 0.9238795325112869605, 1.000000000000000000, 0.9238795325112869605, 1.000000000000000000, 0.9238795325112869605, 1.000000000000000000, 0.9238795325112869605, 1.000000000000000000, 0.9238795325112869605, 1.000000000000000000, 0.9238795325112869605, 1.000000000000000000, 0.9238795325112869605, 1.000000000000000000, 0.9238795325112869605, 1.000000000000000000, 0.9238795325112869605, 1.000000000000000000, 0.9238795325112869605, 1.000000000000000000, 0.9238795325112869605, 1.000000000000000000, 0.9238795325112869605, 1.000000000000000000, 0.9238795325112869605, 1.000000000000000000, 0.9238795325112869605, 1.000000000000000000, 0.9238795325112869605, 1.000000000000000000, 0.9238795325112869605, 1.000000000000000000, 0.9238795325112869605, 1.000000000000000000, 0.9238795325112869605, 1.000000000000000000, 0.9238795325112869605, 1.000000000000000000, 0.9238795325112869605, 1.000000000000000000, 0.9238795325112869605, 1.000000000000000000, 0.9238795325112869605, 1.000000000000000000, 0.9238795325112869605, 1.000000000000000000, 0.9238795325112869605, 1.000000000000000000, 0.9238795325112869605, 1.000000000000000000, 0.9238795325112869605, 1.000000000000000000, 0.9238795325112869605, 1.000000000000000000, 0.9238795325112869605, 1.000000000000000000, 0.9238795325112869605, 1.000000000000000000, 0.9238795325112869605, 1.000000000000000000, 0.9238795325112869605, 1.000000000000000000, 0.9238795325112869605, 1.000000000000000000, 0.9238795325112869605, 1.000000000000000000, 0.9238795325112869605, 1.000000000000000000, 0.9238795325112869605, 1.000000000000000000, 0.9238795325112869605, 1.000000000000000000, 0.9238795325112869605, 1.000000000000000000, 0.9238795325112869605, 1.000000000000000000, 0.9238795325112869605, 1.000000000000000000, 0.9238795325112869605, 1.000000000000000000, 0.9238795325112869605, 1.000000000000000000, 0.9238795325112869605, 1.000000000000000000, 0.9238795325112869605, 1.000000000000000000, 0.9238795325112869605, 1.000000000000000000, 0.9238795325112869605, 1.000000000000000000, 0.9238795325112869605, 1.000000000000000000, 0.9238795325112869605, 1.000000000000000000, 0.9238795325112869605, 1.000000000000000000, 0.9238795325112869605, 1.000000000000000000, 0.9238795325112869605, 1.000000000000000000, 0.9238795325112869605, 1.000000000000000000, 0.9238795325112869605, 1.000000000000000000) ) ) 
 REPRESENTATION_ITEM ( '' )  SURFACE ( )  );
#35468=CARTESIAN_POINT ( 'NONE',  ( 111.1770983795247787, -0.7896495226426338832, -9.318865927141430916 ) ) ;
#35471=CARTESIAN_POINT ( 'NONE',  ( 116.2471765045247594, -2.791137627527887410, -8.388885654883788234 ) ) ;
#35472=CARTESIAN_POINT ( 'NONE',  ( 109.2294423643528347, -4.911049476578604356, -7.814831654473923805 ) ) ;
#35474=VECTOR ( 'NONE', #17699, 1000.000000000000000 ) ;
#35475=CARTESIAN_POINT ( 'NONE',  ( 113.1912390045248031, 0.8980012041604421569, -15.77991374673208469 ) ) ;
#35476=DIRECTION ( 'NONE',  ( 1.000000000000000000, 1.671245155169139691E-16, 0.000000000000000000 ) ) ;
#35479=CARTESIAN_POINT ( 'NONE',  ( 110.5520202545248054, -10.62599879583958717, -15.77991374673208469 ) ) ;
#35490=CARTESIAN_POINT ( 'NONE',  ( 113.2606921295247702, 0.8980012041604618078, -13.39321520033831447 ) ) ;
#35500=CARTESIAN_POINT ( 'NONE',  ( 115.9693640045247776, -10.62599879583958717, -11.00651665394454604 ) ) ;
#35519=CARTESIAN_POINT ( 'NONE',  ( 114.5803015045248117, -6.936859964151250502, -18.39754474579286025 ) ) ;
#35520=CARTESIAN_POINT ( 'NONE',  ( 69.69189222814998175, -41.76310523276723785, -6.393215200338315363 ) ) ;
#35524=VERTEX_POINT ( 'NONE', #10425 ) ;
#35531=CARTESIAN_POINT ( 'NONE',  ( 110.6214733795247867, -1.325403438956436419, -9.854619843455211026 ) ) ;
#35539=B_SPLINE_CURVE_WITH_KNOTS ( 'NONE', 3,
 ( #29485, #11496, #25401, #11944, #39531, #36312, #39299, #42949, #39748, #5082, #19229, #12395, #43398, #22643, #8069, #26295, #33110, #4861, #8968, #40202, #19448 ),
 .UNSPECIFIED., .F., .F.,
 ( 4, 2, 2, 1, 1, 2, 2, 2, 1, 2, 2, 4 ),
 ( 0.000000000000000000, 0.2500000000000362488, 0.3750000000000469624, 0.4375000000000521250, 0.4687500000000549005, 0.4843750000000563438, 0.5000000000000577316, 0.6250000000000136557, 0.6875000000000022204, 0.7187499999999964473, 0.7499999999999905631, 1.000000000000000000 ),
 .UNSPECIFIED. ) ;
#35547=DIRECTION ( 'NONE',  ( -1.000000000000000000, 0.000000000000000000, 0.000000000000000000 ) ) ;
#35553=CARTESIAN_POINT ( 'NONE',  ( 111.3160046295247838, -4.863998795839541422, -18.39754474579285315 ) ) ;
#35563=AXIS2_PLACEMENT_3D ( 'NONE', #34148, #30286, #13426 ) ;
#35576=CARTESIAN_POINT ( 'NONE',  ( 115.6220983795247861, -8.402594152722688392, -16.93181055722141792 ) ) ;
#35577=CARTESIAN_POINT ( 'NONE',  ( 114.3719421295247827, -9.868328341294093420, -13.39321520033831447 ) ) ;
#35580=VERTEX_POINT ( 'NONE', #17268 ) ;
#35583=CARTESIAN_POINT ( 'NONE',  ( 108.3989733795248753, -8.938348069036489818, -17.46756447353520159 ) ) ;
#35584=CARTESIAN_POINT ( 'NONE',  ( 61.69189222814998175, -40.21211973637273474, -6.893215200338315363 ) ) ;
#35586=EDGE_CURVE ( 'NONE', #29714, #9856, #11088, .T. ) ;
#35588=CARTESIAN_POINT ( 'NONE',  ( 109.2294647402427472, -0.3627424684288433343, -15.75041896508675521 ) ) ;
#35589=DIRECTION ( 'NONE',  ( -1.000000000000000000, 0.000000000000000000, 0.000000000000000000 ) ) ;
#35591=CARTESIAN_POINT ( 'NONE',  ( 115.9693640045247776, -10.62599879583958717, -11.00651665394454604 ) ) ;
#35592=CARTESIAN_POINT ( 'NONE',  ( 110.4131140045248287, 0.1403307496149616695, -15.46607636864997204 ) ) ;
#35598=UNCERTAINTY_MEASURE_WITH_UNIT (LENGTH_MEASURE( 1.000000000000000082E-05 ), #33697, 'distance_accuracy_value', 'NONE');
#35610=CARTESIAN_POINT ( 'NONE',  ( 107.2877233795247776, -1.325403438956436419, -9.854619843455211026 ) ) ;
#35611=CARTESIAN_POINT ( 'NONE',  ( 69.17459910784975818, -26.47815602666253909, -5.893215200338315363 ) ) ;
#35613=VERTEX_POINT ( 'NONE', #17477 ) ;
#35614=ORIENTED_EDGE ( 'NONE', *, *, #8956, .T. ) ;
#35624=CARTESIAN_POINT ( 'NONE',  ( 109.7185827545247889, -2.477300249445798297, -19.15521520033831138 ) ) ;
#35632=CARTESIAN_POINT ( 'NONE',  ( 85.61003441325739516, -27.00049153487613651, -8.010338156994905034 ) ) ;
#35633=CARTESIAN_POINT ( 'NONE',  ( 116.5944421295247793, -0.02276961308034231024, -12.14321520033831625 ) ) ;
#35640=CARTESIAN_POINT ( 'NONE',  ( 113.6079577545248043, -7.250697342233347165, -7.631215200338321125 ) ) ;
#35645=DIRECTION ( 'NONE',  ( 0.000000000000000000, 0.000000000000000000, -1.000000000000000000 ) ) ;
#35647=CARTESIAN_POINT ( 'NONE',  ( 107.6349890045248401, -9.868328341294098749, -11.32035403202665869 ) ) ;
#35649=CARTESIAN_POINT ( 'NONE',  ( 115.7610046295247912, -4.863998795839590272, -7.631215200338315796 ) ) ;
#35650=CARTESIAN_POINT ( 'NONE',  ( 109.2294894120781805, -5.138589313339342546, -18.58794946807955384 ) ) ;
#35653=CARTESIAN_POINT ( 'NONE',  ( 116.8028015045247940, -6.936859964151250502, -18.39754474579286025 ) ) ;
#35654=CARTESIAN_POINT ( 'NONE',  ( 114.5108483795247878, -8.402594152722688392, -16.93181055722141792 ) ) ;
#35656=DIRECTION ( 'NONE',  ( -0.6383198453882292789, -0.7697712484781092934, 0.000000000000000000 ) ) ;
#35672=CARTESIAN_POINT ( 'NONE',  ( 109.7880358795247986, -0.7896495226426338832, -17.46756447353520159 ) ) ;
#35674=CARTESIAN_POINT ( 'NONE',  ( 111.8021765045248372, -2.791137627527939813, -8.388885654883777576 ) ) ;
#35677=CARTESIAN_POINT ( 'NONE',  ( 79.79010115959992788, 5.106172230548961188, -4.893215200338314474 ) ) ;
#35682=CARTESIAN_POINT ( 'NONE',  ( 109.8574890045247940, -9.868328341294098749, -11.32035403202665869 ) ) ;
#35684=LINE ( 'NONE', #14277, #39152 ) ;
#35691=CARTESIAN_POINT ( 'NONE',  ( 90.67797751089673852, -17.83979763915464289, -21.89321520033831447 ) ) ;
#35693=CARTESIAN_POINT ( 'NONE',  ( 114.7886608795247696, -1.325403438956436419, -16.93181055722141792 ) ) ;
#35697=CARTESIAN_POINT ( 'NONE',  ( 108.6767858795247861, -0.7896495226426338832, -17.46756447353520159 ) ) ;
#35700=CARTESIAN_POINT ( 'NONE',  ( 115.8048964071292914, 0.2518737723193609224, -14.64321520033831447 ) ) ;
#35702=CARTESIAN_POINT ( 'NONE',  ( 109.2294487058530024, -3.686508270684544009, -7.993684625048021353 ) ) ;
#35704=CARTESIAN_POINT ( 'NONE',  ( 116.2471765045247594, -7.250697342233347165, -19.15521520033831138 ) ) ;
#35705=LINE ( 'NONE', #32510, #13154 ) ;
#35708=CARTESIAN_POINT ( 'NONE',  ( 111.8021765045248372, -7.250697342233347165, -19.15521520033831138 ) ) ;
#35713=TOROIDAL_SURFACE ( 'NONE', #43742, 1.500000000000000000, 0.5000000000000000000 ) ;
#35721=CARTESIAN_POINT ( 'NONE',  ( 114.6497546295247929, -4.863998795839590272, -7.631215200338315796 ) ) ;
#35728=ORIENTED_EDGE ( 'NONE', *, *, #29196, .T. ) ;
#35732=CARTESIAN_POINT ( 'NONE',  ( 84.87879901378997261, -30.44422003934618814, -7.893215200338315363 ) ) ;
#35736=( BOUNDED_CURVE ( )  B_SPLINE_CURVE ( 2, ( #24292, #27488, #38179, #45040, #6956, #20861, #34741, #33851, #25180, #39078, #17662, #7848, #3963, #7614, #327, #11502, #24949 ),
 .UNSPECIFIED., .F., .T. ) 
 B_SPLINE_CURVE_WITH_KNOTS ( ( 3, 2, 2, 2, 2, 2, 2, 2, 3 ),
 ( 0.3040431156034944515, 0.3125000000000000000, 0.3250000000000000111, 0.3375000000000000222, 0.3499999999999999778, 0.3624999999999999889, 0.3750000000000000000, 0.3875000000000000111, 0.3959568843965060037 ),
 .UNSPECIFIED. ) 
 CURVE ( )  GEOMETRIC_REPRESENTATION_ITEM ( )  RATIONAL_B_SPLINE_CURVE ( ( 0.9666851417651740608, 0.9485006404992000206, 1.000000000000000000, 0.9238795325112869605, 1.000000000000000000, 0.9238795325112869605, 1.000000000000000000, 0.9238795325112869605, 1.000000000000000000, 0.9238795325112869605, 1.000000000000000000, 0.9238795325112869605, 1.000000000000000000, 0.9238795325112869605, 1.000000000000000000, 0.9485006404991980222, 0.9666851417651760592 ) ) 
 REPRESENTATION_ITEM ( '' )  );
#35738=CARTESIAN_POINT ( 'NONE',  ( 83.82415148905927538, -46.76310523276723785, -23.89321520033831803 ) ) ;
#35747=DIRECTION ( 'NONE',  ( 0.000000000000000000, 0.000000000000000000, 1.000000000000000000 ) ) ;
#35749=EDGE_LOOP ( 'NONE', ( #4615, #32428, #44027, #42573 ) ) ;
#35751=CARTESIAN_POINT ( 'NONE',  ( 111.5938171295247940, 0.1403307496149613920, -13.39321520033831447 ) ) ;
#35763=CARTESIAN_POINT ( 'NONE',  ( 105.6208483795248299, -8.402594152722688392, -16.93181055722141792 ) ) ;
#35767=AXIS2_PLACEMENT_3D ( 'NONE', #41070, #13908, #3194 ) ;
#35775=CARTESIAN_POINT ( 'NONE',  ( 115.3442858795247759, -8.402594152722688392, -9.854619843455216355 ) ) ;
#35777=EDGE_CURVE ( 'NONE', #21643, #28223, #37455, .T. ) ;
#35780=ORIENTED_EDGE ( 'NONE', *, *, #40922, .F. ) ;
#35787=DIRECTION ( 'NONE',  ( 0.000000000000000000, 0.000000000000000000, -1.000000000000000000 ) ) ;
#35791=CARTESIAN_POINT ( 'NONE',  ( 78.69189222814998175, -49.76310523276715969, -40.89321520033831092 ) ) ;
#35795=CARTESIAN_POINT ( 'NONE',  ( 116.7089049431057788, -7.157548453469082972, -17.96581380690969709 ) ) ;
#35799=VERTEX_POINT ( 'NONE', #16080 ) ;
#35803=CARTESIAN_POINT ( 'NONE',  ( 105.6208483795248299, -0.7896495226426338832, -9.318865927141430916 ) ) ;
#35804=CARTESIAN_POINT ( 'NONE',  ( 112.3578015045248861, -6.936859964151250502, -18.39754474579286025 ) ) ;
#35807=ORIENTED_EDGE ( 'NONE', *, *, #32097, .F. ) ;
#35810=DIRECTION ( 'NONE',  ( -1.000000000000000000, 0.000000000000000000, 0.000000000000000000 ) ) ;
#35816=CARTESIAN_POINT ( 'NONE',  ( 111.6632702545248605, 0.1403307496149616695, -11.32035403202665336 ) ) ;
#35817=ORIENTED_EDGE ( 'NONE', *, *, #18655, .T. ) ;
#35825=ORIENTED_EDGE ( 'NONE', *, *, #36601, .F. ) ;
#35833=CARTESIAN_POINT ( 'NONE',  ( 106.3848327545248651, -6.936859964151250502, -8.388885654883777576 ) ) ;
#35835=VERTEX_POINT ( 'NONE', #1934 ) ;
#35845=CARTESIAN_POINT ( 'NONE',  ( 112.5661608795247872, -8.938348069036489818, -9.318865927141430916 ) ) ;
#35849=CARTESIAN_POINT ( 'NONE',  ( 143.3676850761856940, -71.37806158163373027, -41.02281774838946404 ) ) ;
#35850=VERTEX_POINT ( 'NONE', #29985 ) ;
#35855=CARTESIAN_POINT ( 'NONE',  ( 116.0388171295248014, -10.62599879583958540, -13.39321520033831447 ) ) ;
#35860=CARTESIAN_POINT ( 'NONE',  ( 113.3301452545248083, 0.8980012041604421569, -11.00651665394454071 ) ) ;
#35866=CARTESIAN_POINT ( 'NONE',  ( 107.8433483795247838, -8.402594152722688392, -16.93181055722141792 ) ) ;
#35871=CARTESIAN_POINT ( 'NONE',  ( 109.2294421713136359, -9.862771980732020438, -10.64487995292914668 ) ) ;
#35873=CARTESIAN_POINT ( 'NONE',  ( 112.0799890045248475, -9.868328341294098749, -11.32035403202665869 ) ) ;
#35874=CARTESIAN_POINT ( 'NONE',  ( 114.2330358795247776, -8.402594152722688392, -9.854619843455216355 ) ) ;
#35877=DIRECTION ( 'NONE',  ( 0.000000000000000000, 0.9284778069183722282, 0.3713878862591645791 ) ) ;
#35878=EDGE_CURVE ( 'NONE', #14664, #37700, #15348, .T. ) ;
#35889=EDGE_CURVE ( 'NONE', #18915, #17900, #22940, .T. ) ;
#35890=CIRCLE ( 'NONE', #13375, 4.500000000000003553 ) ;
#35894=CARTESIAN_POINT ( 'NONE',  ( 110.7603796295247918, -4.863998795839590272, -19.15521520033831493 ) ) ;
#35900=CARTESIAN_POINT ( 'NONE',  ( 112.2883483795247770, -8.402594152722688392, -16.93181055722141792 ) ) ;
#35907=CARTESIAN_POINT ( 'NONE',  ( 112.3807811052981691, 0.4930828106259610433, -12.14321520033829849 ) ) ;
#35908=CARTESIAN_POINT ( 'NONE',  ( 111.3160046295247838, -4.863998795839590272, -18.39754474579285315 ) ) ;
#35919=CARTESIAN_POINT ( 'NONE',  ( 114.9970202545248412, 0.1403307496149616695, -11.32035403202665336 ) ) ;
#35924=CARTESIAN_POINT ( 'NONE',  ( 86.25676480896552789, -26.61243077327098661, -8.441090345486626845 ) ) ;
#35925=CARTESIAN_POINT ( 'NONE',  ( 106.5237390045248418, 0.8980012041604421569, -15.77991374673208469 ) ) ;
#35931=CARTESIAN_POINT ( 'NONE',  ( 116.4555358795247884, -0.7896495226426338832, -17.46756447353520159 ) ) ;
#35932=DIRECTION ( 'NONE',  ( -0.2588190451025191297, 0.9659258262890686453, 0.000000000000000000 ) ) ;
#35933=CARTESIAN_POINT ( 'NONE',  ( 116.3166296295247832, -4.863998795839590272, -19.15521520033831493 ) ) ;
#35936=DIRECTION ( 'NONE',  ( -1.000000000000000000, 0.000000000000000000, 0.000000000000000000 ) ) ;
#35941=EDGE_CURVE ( 'NONE', #30697, #20261, #27253, .T. ) ;
#35947=CARTESIAN_POINT ( 'NONE',  ( 113.3995983795247895, -0.7896495226426338832, -9.318865927141430916 ) ) ;
#35961=ADVANCED_FACE ( 'NONE', ( #10150 ), #17574, .T. ) ;
#35975=CARTESIAN_POINT ( 'NONE',  ( 115.3442858795247759, -8.402594152722688392, -9.854619843455216355 ) ) ;
#35979=CARTESIAN_POINT ( 'NONE',  ( 115.8304577545247582, -2.791137627527939813, -18.39754474579286025 ) ) ;
#35980=ORIENTED_EDGE ( 'NONE', *, *, #5532, .T. ) ;
#35984=LINE ( 'NONE', #886, #8609 ) ;
#35986=CARTESIAN_POINT ( 'NONE',  ( 106.8015515045248378, -6.936859964151250502, -18.39754474579286025 ) ) ;
#35999=CARTESIAN_POINT ( 'NONE',  ( 115.0664733795247798, -1.325403438956436419, -9.854619843455211026 ) ) ;
#36003=( BOUNDED_CURVE ( )  B_SPLINE_CURVE ( 3, ( #32130, #35084, #35312, #4765 ),
 .UNSPECIFIED., .F., .T. ) 
 B_SPLINE_CURVE_WITH_KNOTS ( ( 4, 4 ),
 ( 1.570796326794899889, 3.141592653589795336 ),
 .UNSPECIFIED. ) 
 CURVE ( )  GEOMETRIC_REPRESENTATION_ITEM ( )  RATIONAL_B_SPLINE_CURVE ( ( 1.000000000000000000, 0.8047378541243659367, 0.8047378541243659367, 1.000000000000000000 ) ) 
 REPRESENTATION_ITEM ( '' )  );
#36010=ORIENTED_EDGE ( 'NONE', *, *, #3646, .T. ) ;
#36017=VECTOR ( 'NONE', #19774, 1000.000000000000114 ) ;
#36019=CARTESIAN_POINT ( 'NONE',  ( 86.84453910206313765, -17.83168818462593919, -19.39321520033831447 ) ) ;
#36020=DIRECTION ( 'NONE',  ( 0.000000000000000000, 0.000000000000000000, 1.000000000000000000 ) ) ;
#36023=CARTESIAN_POINT ( 'NONE',  ( 116.6756230178623639, -8.487090413082341911, -16.95583224994113891 ) ) ;
#36029=CARTESIAN_POINT ( 'NONE',  ( 114.8581140045248361, -10.62599879583958717, -11.00651665394454604 ) ) ;
#36030=CARTESIAN_POINT ( 'NONE',  ( 109.0935046295247872, -4.863998795839590272, -18.39754474579285315 ) ) ;
#36031=CARTESIAN_POINT ( 'NONE',  ( 110.0658483795247804, -8.402594152722688392, -16.93181055722141792 ) ) ;
#36034=VERTEX_POINT ( 'NONE', #15113 ) ;
#36036=CARTESIAN_POINT ( 'NONE',  ( 108.7462390045248242, 0.8980012041604421569, -15.77991374673208469 ) ) ;
#36042=CARTESIAN_POINT ( 'NONE',  ( 110.3436608795247764, -8.938348069036489818, -9.318865927141430916 ) ) ;
#36043=CARTESIAN_POINT ( 'NONE',  ( 110.6909265045248247, -2.791137627527939813, -8.388885654883777576 ) ) ;
#36044=AXIS2_PLACEMENT_3D ( 'NONE', #27853, #16698, #41763 ) ;
#36051=PRODUCT_DEFINITION_CONTEXT ( 'detailed design', #11383, 'design' ) ;
#36054=ORIENTED_EDGE ( 'NONE', *, *, #27569, .F. ) ;
#36061=CARTESIAN_POINT ( 'NONE',  ( 107.1488171295247867, 0.1403307496149613920, -13.39321520033831447 ) ) ;
#36063=EDGE_LOOP ( 'NONE', ( #30864, #34077, #34439, #5206 ) ) ;
#36072=CARTESIAN_POINT ( 'NONE',  ( 71.77086717554882966, -26.54201219542348511, -4.893215200338314474 ) ) ;
#36074=CARTESIAN_POINT ( 'NONE',  ( 110.3436608795247764, -8.938348069036489818, -9.318865927141430916 ) ) ;
#36080=ORIENTED_EDGE ( 'NONE', *, *, #3335, .F. ) ;
#36084=CARTESIAN_POINT ( 'NONE',  ( 67.69189222814998175, -42.70034233532976486, -10.06214201013430909 ) ) ;
#36086=CARTESIAN_POINT ( 'NONE',  ( 114.1635827545248389, -2.477300249445798297, -19.15521520033831138 ) ) ;
#36091=CARTESIAN_POINT ( 'NONE',  ( 109.2324108795247923, -8.938348069036489818, -9.318865927141430916 ) ) ;
#36095=CARTESIAN_POINT ( 'NONE',  ( 117.1405054202893155, -11.23569791401464713, -5.537001952796093640 ) ) ;
#36096=CARTESIAN_POINT ( 'NONE',  ( 105.8292077545248446, -2.791137627527939813, -18.39754474579286025 ) ) ;
#36099=CARTESIAN_POINT ( 'NONE',  ( 109.2294691412240297, -9.956217823165619762, -15.41276842522689350 ) ) ;
#36102=CARTESIAN_POINT ( 'NONE',  ( 114.0941296295247867, -4.863998795839590272, -8.388885654883775800 ) ) ;
#36103=CARTESIAN_POINT ( 'NONE',  ( 114.9970202545248412, 0.1403307496149616695, -11.32035403202665336 ) ) ;
#36108=ORIENTED_EDGE ( 'NONE', *, *, #7185, .T. ) ;
#36114=ORIENTED_EDGE ( 'NONE', *, *, #33249, .F. ) ;
#36116=CIRCLE ( 'NONE', #1907, 2.999999999999998224 ) ;
#36121=ADVANCED_FACE ( 'NONE', ( #18307 ), #25155, .T. ) ;
#36122=CARTESIAN_POINT ( 'NONE',  ( 115.7610046295247912, -4.863998795839590272, -18.39754474579285315 ) ) ;
#36128=CARTESIAN_POINT ( 'NONE',  ( 117.0143358795247792, -1.328464889906837199, -16.92874910627105223 ) ) ;
#36129=CARTESIAN_POINT ( 'NONE',  ( 110.8298327545248299, -6.936859964151250502, -8.388885654883777576 ) ) ;
#36141=CARTESIAN_POINT ( 'NONE',  ( 108.8156921295247912, -9.868328341294093420, -13.39321520033831447 ) ) ;
#36147=CARTESIAN_POINT ( 'NONE',  ( 106.8710046295248759, -4.863998795839590272, -7.631215200338315796 ) ) ;
#36153=CARTESIAN_POINT ( 'NONE',  ( 116.3860827545247787, -2.477300249445798297, -19.15521520033831138 ) ) ;
#36158=CARTESIAN_POINT ( 'NONE',  ( 106.8710046295248759, -4.863998795839590272, -7.631215200338315796 ) ) ;
#36161=EDGE_CURVE ( 'NONE', #13861, #6063, #22619, .T. ) ;
#36172=CARTESIAN_POINT ( 'NONE',  ( 111.5243640045248412, -10.62599879583958717, -11.00651665394454604 ) ) ;
#36174=CARTESIAN_POINT ( 'NONE',  ( 110.8992858795247827, -0.7896495226426338832, -17.46756447353518382 ) ) ;
#36184=CARTESIAN_POINT ( 'NONE',  ( 115.4328884760651874, 0.6362173239733635022, -12.14321520033831625 ) ) ;
#36186=CYLINDRICAL_SURFACE ( 'NONE', #23707, 1.000000000000000888 ) ;
#36187=CARTESIAN_POINT ( 'NONE',  ( 64.59495755916755400, -36.13370383219653803, -5.723731037142725242 ) ) ;
#36191=DIRECTION ( 'NONE',  ( 0.000000000000000000, 0.3713878862591638574, -0.9284778069183724503 ) ) ;
#36200=CARTESIAN_POINT ( 'NONE',  ( 116.8722546295247895, -4.863998795839590272, -18.39754474579285315 ) ) ;
#36204=CARTESIAN_POINT ( 'NONE',  ( 113.1912390045248031, 0.8980012041604421569, -15.77991374673208469 ) ) ;
#36205=CARTESIAN_POINT ( 'NONE',  ( 112.7050671295247923, 0.1403307496149613920, -13.39321520033831447 ) ) ;
#36217=CARTESIAN_POINT ( 'NONE',  ( 109.8574890045248509, -9.868328341294098749, -11.32035403202665869 ) ) ;
#36225=DIRECTION ( 'NONE',  ( -1.000000000000000000, 0.000000000000000000, 0.000000000000000000 ) ) ;
#36227=CARTESIAN_POINT ( 'NONE',  ( 114.3719421295247827, -9.868328341294093420, -13.39321520033831447 ) ) ;
#36231=ORIENTED_EDGE ( 'NONE', *, *, #31486, .T. ) ;
#36234=CARTESIAN_POINT ( 'NONE',  ( 111.1770983795247787, -8.402594152722633325, -16.93181055722145345 ) ) ;
#36239=CARTESIAN_POINT ( 'NONE',  ( 110.1353015045248185, -6.936859964151197211, -18.39754474579288512 ) ) ;
#36240=CARTESIAN_POINT ( 'NONE',  ( 114.9740004229301888, 0.1075849324168598464, -14.64321520033831447 ) ) ;
#36249=DIRECTION ( 'NONE',  ( -0.3445294493088598697, -0.9387755102040815647, 0.000000000000000000 ) ) ;
#36255=CARTESIAN_POINT ( 'NONE',  ( 116.4555358795247884, -0.7896495226426338832, -17.46756447353520159 ) ) ;
#36256=CARTESIAN_POINT ( 'NONE',  ( 108.3989733795248753, -1.325403438956436419, -9.854619843455211026 ) ) ;
#36257=CARTESIAN_POINT ( 'NONE',  ( 111.0381921295247878, -9.868328341294093420, -13.39321520033831447 ) ) ;
#36261=VERTEX_POINT ( 'NONE', #19207 ) ;
#36262=CARTESIAN_POINT ( 'NONE',  ( 106.7320983795247855, -0.7896495226426338832, -9.318865927141430916 ) ) ;
#36265=CARTESIAN_POINT ( 'NONE',  ( 109.2295757755578762, -0.1086748408276279887, -15.25738775639926992 ) ) ;
#36268=CARTESIAN_POINT ( 'NONE',  ( 109.6491296295247793, -4.863998795839590272, -19.15521520033831493 ) ) ;
#36269=CARTESIAN_POINT ( 'NONE',  ( 112.3578015045248861, -6.936859964151250502, -18.39754474579286025 ) ) ;
#36271=CARTESIAN_POINT ( 'NONE',  ( 110.9518144685027750, 0.6938714319018670640, -14.64321520033828072 ) ) ;
#36276=( BOUNDED_CURVE ( )  B_SPLINE_CURVE ( 3, ( #8408, #25960, #879, #4749 ),
 .UNSPECIFIED., .F., .T. ) 
 B_SPLINE_CURVE_WITH_KNOTS ( ( 4, 4 ),
 ( 3.141592653589785122, 4.712388980384700332 ),
 .UNSPECIFIED. ) 
 CURVE ( )  GEOMETRIC_REPRESENTATION_ITEM ( )  RATIONAL_B_SPLINE_CURVE ( ( 1.000000000000000000, 0.8047378541243619399, 0.8047378541243619399, 1.000000000000000000 ) ) 
 REPRESENTATION_ITEM ( '' )  );
#36281=CARTESIAN_POINT ( 'NONE',  ( 113.5348452706805915, 0.3193521225029610777, -14.64321520033833401 ) ) ;
#36287=CARTESIAN_POINT ( 'NONE',  ( 116.1082702545247827, -10.62599879583958717, -15.77991374673208469 ) ) ;
#36296=CARTESIAN_POINT ( 'NONE',  ( 71.62231439647737830, -24.74987456741813929, -4.893215200338314474 ) ) ;
#36297=CARTESIAN_POINT ( 'NONE',  ( 110.4131140045248287, -10.62599879583958717, -11.00651665394454604 ) ) ;
#36303=EDGE_LOOP ( 'NONE', ( #36735, #3905, #18038, #12446, #7850 ) ) ;
#36306=CARTESIAN_POINT ( 'NONE',  ( 112.5661608795247872, -8.938348069036489818, -9.318865927141430916 ) ) ;
#36307=CARTESIAN_POINT ( 'NONE',  ( 115.9693640045247776, 0.1403307496149616695, -15.46607636864997204 ) ) ;
#36308=CARTESIAN_POINT ( 'NONE',  ( 110.6214733795247867, -8.938348069036489818, -17.46756447353520159 ) ) ;
#36312=CARTESIAN_POINT ( 'NONE',  ( 62.62167863469137075, -37.39737710839052198, -5.203302251594248418 ) ) ;
#36313=CARTESIAN_POINT ( 'NONE',  ( 107.0793640045248196, -10.62599879583958717, -11.00651665394454604 ) ) ;
#36317=CARTESIAN_POINT ( 'NONE',  ( 117.2221267808402985, -10.92304153767783959, -5.282372476044864484 ) ) ;
#36319=FACE_OUTER_BOUND ( 'NONE', #34920, .T. ) ;
#36320=CARTESIAN_POINT ( 'NONE',  ( 109.2294471768124424, -10.42840437825952549, -12.68791898119246042 ) ) ;
#36323=CARTESIAN_POINT ( 'NONE',  ( 111.1770983795247787, -8.402594152722688392, -16.93181055722141792 ) ) ;
#36324=CARTESIAN_POINT ( 'NONE',  ( 115.9693640045247776, 0.1403307496149616695, -15.46607636864997204 ) ) ;
#36326=DIRECTION ( 'NONE',  ( 0.000000000000000000, -0.3713878862591642460, 0.9284778069183722282 ) ) ;
#36327=CARTESIAN_POINT ( 'NONE',  ( 68.95535311261431843, -26.02754444259658584, -5.893215200338315363 ) ) ;
#36340=CARTESIAN_POINT ( 'NONE',  ( 105.8986608795248401, -8.938348069036489818, -9.318865927141430916 ) ) ;
#36343=CARTESIAN_POINT ( 'NONE',  ( 113.4690515045247992, -6.936859964151250502, -18.39754474579286025 ) ) ;
#36345=CARTESIAN_POINT ( 'NONE',  ( 70.19189222814998175, -58.73420832284057269, -33.46539274499136241 ) ) ;
#36352=CARTESIAN_POINT ( 'NONE',  ( 116.5944421295247793, -9.868328341294093420, -13.39321520033831447 ) ) ;
#36353=CARTESIAN_POINT ( 'NONE',  ( 109.5796765045248122, -2.791137627527939813, -8.388885654883777576 ) ) ;
#36356=CARTESIAN_POINT ( 'NONE',  ( 107.2294421295247844, -9.051693226400931991, -21.89321520033831447 ) ) ;
#36364=CARTESIAN_POINT ( 'NONE',  ( 107.9128015045248219, -6.936859964151250502, -18.39754474579286025 ) ) ;
#36370=CARTESIAN_POINT ( 'NONE',  ( 107.3571765045248299, -7.250697342233347165, -19.15521520033831138 ) ) ;
#36374=CARTESIAN_POINT ( 'NONE',  ( 78.69189222814998175, -64.41823023953079996, -19.25521411788948711 ) ) ;
#36375=CARTESIAN_POINT ( 'NONE',  ( 113.8163171295247764, -10.62599879583958540, -13.39321520033831447 ) ) ;
#36380=CARTESIAN_POINT ( 'NONE',  ( 106.3153796295248412, -4.863998795839590272, -19.15521520033831493 ) ) ;
#36382=DIRECTION ( 'NONE',  ( -8.728168432587710164E-16, -1.000000000000000000, 0.000000000000000000 ) ) ;
#36384=CARTESIAN_POINT ( 'NONE',  ( 116.0861162244890892, -0.02276961308034231024, -12.14321520033833934 ) ) ;
#36391=CARTESIAN_POINT ( 'NONE',  ( 108.0517077545248696, -7.250697342233347165, -7.631215200338321125 ) ) ;
#36392=VECTOR ( 'NONE', #9770, 1000.000000000000000 ) ;
#36396=ORIENTED_EDGE ( 'NONE', *, *, #18655, .F. ) ;
#36402=CARTESIAN_POINT ( 'NONE',  ( 115.1614878519202847, 0.2518737723193609224, -12.14321520033831625 ) ) ;
#36404=CARTESIAN_POINT ( 'NONE',  ( 61.69189222814998175, -49.76310523276723785, -7.393215200338315363 ) ) ;
#36419=CARTESIAN_POINT ( 'NONE',  ( 115.4831921295247952, -9.868328341294093420, -13.39321520033831447 ) ) ;
#36424=CARTESIAN_POINT ( 'NONE',  ( 115.2748327545248657, -2.477300249445798297, -19.15521520033831138 ) ) ;
#36425=CARTESIAN_POINT ( 'NONE',  ( 109.6491296295247793, -4.863998795839590272, -8.388885654883775800 ) ) ;
#36430=CARTESIAN_POINT ( 'NONE',  ( 116.4555358795247884, -8.402594152722688392, -9.854619843455216355 ) ) ;
#36432=VECTOR ( 'NONE', #31364, 1000.000000000000227 ) ;
#36437=CARTESIAN_POINT ( 'NONE',  ( 108.1906140045248463, 0.1403307496149616695, -15.46607636864997204 ) ) ;
#36448=EDGE_CURVE ( 'NONE', #20559, #7488, #27180, .T. ) ;
#36449=CARTESIAN_POINT ( 'NONE',  ( 113.5385046295247804, -4.863998795839590272, -18.39754474579285315 ) ) ;
#36464=EDGE_CURVE ( 'NONE', #26462, #4322, #16406, .T. ) ;
#36465=CARTESIAN_POINT ( 'NONE',  ( 69.69189222814998175, -41.76310523276723785, -19.39321520033831447 ) ) ;
#36474=CARTESIAN_POINT ( 'NONE',  ( 116.6823128682102748, -8.240270276191195009, -17.20524534304492192 ) ) ;
#36480=CARTESIAN_POINT ( 'NONE',  ( 114.4099712410415748, 0.7607806665037644134, -12.14321520033829316 ) ) ;
#36481=CARTESIAN_POINT ( 'NONE',  ( 109.9269421295247753, 0.8980012041604618078, -13.39321520033831447 ) ) ;
#36482=CARTESIAN_POINT ( 'NONE',  ( 111.5243640045248412, 0.1403307496149616695, -15.46607636864997204 ) ) ;
#36483=CARTESIAN_POINT ( 'NONE',  ( 109.9963952545248134, -9.868328341294098749, -15.46607636864997204 ) ) ;
#36493=CARTESIAN_POINT ( 'NONE',  ( 111.5243640045248412, -10.62599879583958717, -11.00651665394454604 ) ) ;
#36508=ORIENTED_EDGE ( 'NONE', *, *, #11402, .T. ) ;
#36509=DIRECTION ( 'NONE',  ( -1.000000000000000000, 0.000000000000000000, 0.000000000000000000 ) ) ;
#36511=CARTESIAN_POINT ( 'NONE',  ( 115.6220983795247861, -0.7896495226426338832, -9.318865927141430916 ) ) ;
#36513=ADVANCED_FACE ( 'NONE', ( #13940 ), #37880, .F. ) ;
#36522=CARTESIAN_POINT ( 'NONE',  ( 62.73714355202354653, -64.74057374251856345, -45.90754283741456732 ) ) ;
#36523=CARTESIAN_POINT ( 'NONE',  ( 108.1906140045248463, -10.62599879583958717, -11.00651665394454604 ) ) ;
#36530=EDGE_LOOP ( 'NONE', ( #14394, #34914, #6116, #13177 ) ) ;
#36533=CARTESIAN_POINT ( 'NONE',  ( 112.2883483795247770, -0.7896495226426338832, -9.318865927141430916 ) ) ;
#36535=CARTESIAN_POINT ( 'NONE',  ( 112.1494421295248003, 0.8980012041604618078, -13.39321520033831447 ) ) ;
#36537=ORIENTED_EDGE ( 'NONE', *, *, #17908, .F. ) ;
#36540=CARTESIAN_POINT ( 'NONE',  ( 107.2877233795247776, -8.938348069036489818, -17.46756447353520159 ) ) ;
#36547=CARTESIAN_POINT ( 'NONE',  ( 109.2295002756012963, -10.42642047080344270, -13.52344292549696014 ) ) ;
#36549=CARTESIAN_POINT ( 'NONE',  ( 110.4131140045248287, 0.1403307496149616695, -15.46607636864997204 ) ) ;
#36550=CARTESIAN_POINT ( 'NONE',  ( 114.4413952545248350, -9.868328341294098749, -15.46607636864997204 ) ) ;
#36553=CARTESIAN_POINT ( 'NONE',  ( 69.87170781386352303, -25.28162009068048732, -5.721420406450495655 ) ) ;
#36556=ORIENTED_EDGE ( 'NONE', *, *, #24435, .F. ) ;
#36558=VECTOR ( 'NONE', #26960, 1000.000000000000000 ) ;
#36568=CARTESIAN_POINT ( 'NONE',  ( 106.5237390045248418, 0.8980012041604421569, -15.77991374673208469 ) ) ;
#36571=CARTESIAN_POINT ( 'NONE',  ( 109.0935046295247872, -4.863998795839590272, -18.39754474579285315 ) ) ;
#36581=CARTESIAN_POINT ( 'NONE',  ( 112.3578015045248861, -6.936859964151250502, -18.39754474579286025 ) ) ;
#36593=CARTESIAN_POINT ( 'NONE',  ( 109.5102233795247884, -1.325403438956436419, -9.854619843455211026 ) ) ;
#36597=CARTESIAN_POINT ( 'NONE',  ( 110.2047546295247855, -4.863998795839590272, -7.631215200338315796 ) ) ;
#36600=FACE_OUTER_BOUND ( 'NONE', #2005, .T. ) ;
#36601=EDGE_CURVE ( 'NONE', #21089, #31466, #39220, .T. ) ;
#36602=CARTESIAN_POINT ( 'NONE',  ( 112.5661608795247872, -8.938348069036489818, -9.318865927141430916 ) ) ;
#36604=CARTESIAN_POINT ( 'NONE',  ( 116.5249890045247980, 0.8980012041604421569, -15.77991374673208469 ) ) ;
#36607=CARTESIAN_POINT ( 'NONE',  ( 105.8292077545248446, -7.250697342233347165, -7.631215200338321125 ) ) ;
#36618=CARTESIAN_POINT ( 'NONE',  ( 107.0793640045248196, -10.62599879583958717, -11.00651665394454604 ) ) ;
#36621=CARTESIAN_POINT ( 'NONE',  ( 116.7836398906078017, -3.487082921028213711, -18.39717223183647477 ) ) ;
#36626=CARTESIAN_POINT ( 'NONE',  ( 113.6774108795247997, -1.325403438956436419, -16.93181055722138595 ) ) ;
#36629=EDGE_CURVE ( 'NONE', #11127, #26421, #43613, .T. ) ;
#36642=ORIENTED_EDGE ( 'NONE', *, *, #34210, .T. ) ;
#36645=CARTESIAN_POINT ( 'NONE',  ( 113.2606921295247702, -9.868328341294093420, -13.39321520033831447 ) ) ;
#36649=CARTESIAN_POINT ( 'NONE',  ( 114.3719421295247827, 0.8980012041604618078, -13.39321520033831447 ) ) ;
#36650=CARTESIAN_POINT ( 'NONE',  ( 109.5102233795247884, -1.325403438956436419, -9.854619843455211026 ) ) ;
#36652=VECTOR ( 'NONE', #6363, 1000.000000000000000 ) ;
#36654=CARTESIAN_POINT ( 'NONE',  ( 112.6356140045247827, 0.1403307496149616695, -15.46607636864997204 ) ) ;
#36660=CARTESIAN_POINT ( 'NONE',  ( 106.3153796295248412, -4.863998795839590272, -8.388885654883775800 ) ) ;
#36661=ORIENTED_EDGE ( 'NONE', *, *, #33534, .T. ) ;
#36670=CARTESIAN_POINT ( 'NONE',  ( 112.5661608795247872, -1.325403438956436419, -16.93181055722141792 ) ) ;
#36673=VERTEX_POINT ( 'NONE', #32147 ) ;
#36678=ORIENTED_EDGE ( 'NONE', *, *, #20834, .T. ) ;
#36680=PLANE ( 'NONE',  #42753 ) ;
#36696=VERTEX_POINT ( 'NONE', #11419 ) ;
#36699=CARTESIAN_POINT ( 'NONE',  ( 110.6909265045248247, -7.250697342233347165, -19.15521520033831138 ) ) ;
#36700=CARTESIAN_POINT ( 'NONE',  ( 108.2600671295247992, 0.1403307496149613920, -13.39321520033831447 ) ) ;
#36701=CARTESIAN_POINT ( 'NONE',  ( 110.4131140045248287, 0.1403307496149616695, -15.46607636864997204 ) ) ;
#36710=CARTESIAN_POINT ( 'NONE',  ( 108.4684265045247997, -7.250697342233347165, -19.15521520033831138 ) ) ;
#36713=DIRECTION ( 'NONE',  ( 0.000000000000000000, 0.000000000000000000, -1.000000000000000000 ) ) ;
#36733=CARTESIAN_POINT ( 'NONE',  ( 114.4413952545248350, 0.8980012041604421569, -11.00651665394454071 ) ) ;
#36735=ORIENTED_EDGE ( 'NONE', *, *, #23687, .T. ) ;
#36736=VERTEX_POINT ( 'NONE', #12091 ) ;
#36741=CARTESIAN_POINT ( 'NONE',  ( 61.80825783966907494, -65.83929257108415811, -43.67008539085770025 ) ) ;
#36754=CARTESIAN_POINT ( 'NONE',  ( 112.6356140045247827, -10.62599879583958717, -11.00651665394454604 ) ) ;
#36755=CARTESIAN_POINT ( 'NONE',  ( 112.7050671295247923, 0.1403307496149613920, -13.39321520033831447 ) ) ;
#36756=CARTESIAN_POINT ( 'NONE',  ( 113.2606921295247702, 0.8980012041604618078, -13.39321520033831447 ) ) ;
#36761=CARTESIAN_POINT ( 'NONE',  ( 107.1488171295247867, -10.62599879583958540, -13.39321520033831447 ) ) ;
#36769=CARTESIAN_POINT ( 'NONE',  ( 109.2294844673402423, -10.43718104171506944, -13.11406945123205858 ) ) ;
#36771=CARTESIAN_POINT ( 'NONE',  ( 113.3301452545248083, -9.868328341294098749, -15.46607636864997204 ) ) ;
#36772=CARTESIAN_POINT ( 'NONE',  ( 113.1217858795247935, -8.402594152722688392, -9.854619843455216355 ) ) ;
#36774=FACE_OUTER_BOUND ( 'NONE', #19635, .T. ) ;
#36775=CARTESIAN_POINT ( 'NONE',  ( 71.24792571258848284, -26.61500810931513428, -5.214987668974215396 ) ) ;
#36778=ORIENTED_EDGE ( 'NONE', *, *, #3317, .T. ) ;
#36779=EDGE_CURVE ( 'NONE', #32851, #29903, #22221, .T. ) ;
#36792=CARTESIAN_POINT ( 'NONE',  ( 105.6903015045248253, -2.477300249445798297, -7.631215200338321125 ) ) ;
#36795=CARTESIAN_POINT ( 'NONE',  ( 108.6073327545248048, -6.936859964151250502, -8.388885654883777576 ) ) ;
#36801=VERTEX_POINT ( 'NONE', #26668 ) ;
#36802=CARTESIAN_POINT ( 'NONE',  ( 116.2471765045247594, -2.791137627527939813, -8.388885654883777576 ) ) ;
#36803=CARTESIAN_POINT ( 'NONE',  ( 107.7044421295247929, -9.868328341294093420, -13.39321520033831447 ) ) ;
#36814=CARTESIAN_POINT ( 'NONE',  ( 110.2742077545248094, -2.791137627527939813, -18.39754474579286025 ) ) ;
#36818=CARTESIAN_POINT ( 'NONE',  ( 74.69189222814998175, -41.76310523276723785, -20.39321520033831447 ) ) ;
#36819=CARTESIAN_POINT ( 'NONE',  ( 115.2748327545248657, -6.936859964151250502, -8.388885654883777576 ) ) ;
#36822=DIRECTION ( 'NONE',  ( -2.439015257082815255E-15, 1.000000000000000000, 0.000000000000000000 ) ) ;
#36823=CARTESIAN_POINT ( 'NONE',  ( 111.1076452545248259, 0.8980012041604421569, -11.00651665394454071 ) ) ;
#36825=CARTESIAN_POINT ( 'NONE',  ( 116.1082702545247827, -10.62599879583958717, -15.77991374673208469 ) ) ;
#36828=CARTESIAN_POINT ( 'NONE',  ( 108.1906140045248463, -10.62599879583958717, -11.00651665394454604 ) ) ;
#36831=ORIENTED_EDGE ( 'NONE', *, *, #10025, .F. ) ;
#36832=CARTESIAN_POINT ( 'NONE',  ( 116.1351496632429416, -0.3638222789105182153, -10.82232390540186984 ) ) ;
#36842=CARTESIAN_POINT ( 'NONE',  ( 109.5102233795247884, -8.938348069036489818, -17.46756447353520159 ) ) ;
#36844=CARTESIAN_POINT ( 'NONE',  ( 110.5520202545248196, -10.62599879583953388, -15.77991374673210601 ) ) ;
#36848=DIRECTION ( 'NONE',  ( -8.728168432587710164E-16, -1.000000000000000000, 0.000000000000000000 ) ) ;
#36866=CARTESIAN_POINT ( 'NONE',  ( 114.3719421295247827, -9.868328341294093420, -13.39321520033831447 ) ) ;
#36870=CARTESIAN_POINT ( 'NONE',  ( 106.1764733795248219, -1.325403438956436419, -9.854619843455211026 ) ) ;
#36871=CARTESIAN_POINT ( 'NONE',  ( 109.2324108795247923, -1.325403438956436419, -16.93181055722141792 ) ) ;
#36877=CARTESIAN_POINT ( 'NONE',  ( 113.9552233795247815, -1.325403438956436419, -9.854619843455211026 ) ) ;
#36884=CARTESIAN_POINT ( 'NONE',  ( 105.0652233795248378, -1.325403438956436419, -9.854619843455211026 ) ) ;
#36885=VECTOR ( 'NONE', #43569, 1000.000000000000114 ) ;
#36889=EDGE_CURVE ( 'NONE', #31933, #30574, #31649, .T. ) ;
#36892=CARTESIAN_POINT ( 'NONE',  ( 71.36400868967236022, -24.42718413923373788, -4.893215200338314474 ) ) ;
#36895=CARTESIAN_POINT ( 'NONE',  ( 111.8021765045248372, -2.791137627527939813, -8.388885654883777576 ) ) ;
#36904=AXIS2_PLACEMENT_3D ( 'NONE', #42262, #7592, #11027 ) ;
#36906=DIRECTION ( 'NONE',  ( 1.000000000000000000, 0.000000000000000000, 0.000000000000000000 ) ) ;
#36922=CARTESIAN_POINT ( 'NONE',  ( 112.0799890045248475, 0.8980012041604421569, -15.77991374673208469 ) ) ;
#36923=CARTESIAN_POINT ( 'NONE',  ( 111.2465515045248168, -6.936859964151250502, -18.39754474579286025 ) ) ;
#36924=CARTESIAN_POINT ( 'NONE',  ( 108.6767858795247861, -8.402594152722688392, -9.854619843455216355 ) ) ;
#36925=CARTESIAN_POINT ( 'NONE',  ( 109.2309317933750634, -8.902407557854933984, -9.282925415959930149 ) ) ;
#36928=DIRECTION ( 'NONE',  ( 0.000000000000000000, 0.000000000000000000, -1.000000000000000000 ) ) ;
#36933=CARTESIAN_POINT ( 'NONE',  ( 107.1488171295248861, 0.1403307496149613920, -13.39321520033831447 ) ) ;
#36935=CARTESIAN_POINT ( 'NONE',  ( 115.2053796295247849, -4.863998795839590272, -8.388885654883775800 ) ) ;
#36938=CARTESIAN_POINT ( 'NONE',  ( 61.76986277844709861, -39.32091226840162079, -6.340220811149025693 ) ) ;
#36941=VECTOR ( 'NONE', #12215, 1000.000000000000000 ) ;
#36953=CARTESIAN_POINT ( 'NONE',  ( 114.5108483795247878, -0.7896495226426338832, -9.318865927141430916 ) ) ;
#36962=CARTESIAN_POINT ( 'NONE',  ( 107.2877233795247776, -8.938348069036489818, -17.46756447353520159 ) ) ;
#36969=EDGE_CURVE ( 'NONE', #42684, #529, #21325, .T. ) ;
#36970=EDGE_CURVE ( 'NONE', #23478, #44558, #19148, .T. ) ;
#36975=CARTESIAN_POINT ( 'NONE',  ( 114.0246765045248196, -7.250697342233347165, -19.15521520033831138 ) ) ;
#36976=CARTESIAN_POINT ( 'NONE',  ( 113.4690515045247992, -6.936859964151250502, -18.39754474579286025 ) ) ;
#36977=CARTESIAN_POINT ( 'NONE',  ( 109.7185827545247889, -2.477300249445798297, -19.15521520033831138 ) ) ;
#36992=CARTESIAN_POINT ( 'NONE',  ( 116.2471765045247594, -7.250697342233347165, -19.15521520033831138 ) ) ;
#36993=CARTESIAN_POINT ( 'NONE',  ( 111.8021765045248372, -2.791137627527939813, -8.388885654883777576 ) ) ;
#36996=CARTESIAN_POINT ( 'NONE',  ( 68.97125867122092302, -25.93985065944693957, -5.893215200338315363 ) ) ;
#37011=( BOUNDED_CURVE ( )  B_SPLINE_CURVE ( 2, ( #17940, #38449, #38899, #32059, #30786, #25236, #42345, #35471, #4246, #25462, #8133 ),
 .UNSPECIFIED., .F., .T. ) 
 B_SPLINE_CURVE_WITH_KNOTS ( ( 3, 2, 2, 2, 2, 3 ),
 ( 0.04958152047947080032, 0.05000000000000000278, 0.06250000000000000000, 0.07499999999999999722, 0.08749999999999999445, 0.09595688439650540413 ),
 .UNSPECIFIED. ) 
 CURVE ( )  GEOMETRIC_REPRESENTATION_ITEM ( )  RATIONAL_B_SPLINE_CURVE ( ( 0.9950738546682840191, 0.9974516114610290085, 1.000000000000000000, 0.9238795325112869605, 1.000000000000000000, 0.9238795325112869605, 1.000000000000000000, 0.9238795325112869605, 1.000000000000000000, 0.9485006404992000206, 0.9666851417651740608 ) ) 
 REPRESENTATION_ITEM ( '' )  );
#37013=CARTESIAN_POINT ( 'NONE',  ( 107.2182702545248105, -10.62599879583958717, -15.77991374673208469 ) ) ;
#37018=DIRECTION ( 'NONE',  ( 0.000000000000000000, 1.000000000000000000, 0.000000000000000000 ) ) ;
#37019=CARTESIAN_POINT ( 'NONE',  ( 110.0658483795247804, -8.402594152722688392, -16.93181055722141792 ) ) ;
#37039=CARTESIAN_POINT ( 'NONE',  ( 109.9269421295247753, -9.868328341294093420, -13.39321520033831447 ) ) ;
#37043=CARTESIAN_POINT ( 'NONE',  ( 112.7745202545247878, 0.1403307496149616695, -11.32035403202665336 ) ) ;
#37045=CARTESIAN_POINT ( 'NONE',  ( 70.36267391504962632, -5.685877709920933221, -7.393215200338315363 ) ) ;
#37047=CARTESIAN_POINT ( 'NONE',  ( 109.9269421295247753, 0.8980012041604618078, -13.39321520033831447 ) ) ;
#37049=CARTESIAN_POINT ( 'NONE',  ( 115.1359265045248605, -7.250697342233347165, -19.15521520033831138 ) ) ;
#37055=VERTEX_POINT ( 'NONE', #30310 ) ;
#37061=ORIENTED_EDGE ( 'NONE', *, *, #40924, .F. ) ;
#37064=CARTESIAN_POINT ( 'NONE',  ( 109.3018640045248304, -10.62599879583958717, -11.00651665394454604 ) ) ;
#37066=CARTESIAN_POINT ( 'NONE',  ( 116.8240514920784818, -1.666881267585053283, -17.53180210756796598 ) ) ;
#37068=ORIENTED_EDGE ( 'NONE', *, *, #35889, .T. ) ;
#37069=VECTOR ( 'NONE', #17435, 1000.000000000000227 ) ;
#37074=DIRECTION ( 'NONE',  ( -1.000000000000000000, 1.091021054073464066E-15, 0.000000000000000000 ) ) ;
#37077=CARTESIAN_POINT ( 'NONE',  ( 108.4684265045248424, -2.791137627527939813, -8.388885654883777576 ) ) ;
#37088=CARTESIAN_POINT ( 'NONE',  ( 116.3860827545247787, -6.936859964151250502, -8.388885654883777576 ) ) ;
#37092=CARTESIAN_POINT ( 'NONE',  ( 114.7192077545248594, -7.250697342233347165, -7.631215200338321125 ) ) ;
#37093=CARTESIAN_POINT ( 'NONE',  ( 108.8851452545248151, -9.868328341294098749, -15.46607636864997204 ) ) ;
#37094=CARTESIAN_POINT ( 'NONE',  ( 83.46578503091454593, -32.14527012763957714, -23.68292775665955574 ) ) ;
#37098=DIRECTION ( 'NONE',  ( 0.000000000000000000, 1.000000000000000000, 1.195183497228115774E-16 ) ) ;
#37099=CARTESIAN_POINT ( 'NONE',  ( 111.8021765045248372, -2.791137627527939813, -8.388885654883777576 ) ) ;
#37100=ORIENTED_EDGE ( 'NONE', *, *, #35889, .F. ) ;
#37109=ORIENTED_EDGE ( 'NONE', *, *, #13941, .T. ) ;
#37118=CARTESIAN_POINT ( 'NONE',  ( 112.2883483795247770, -8.402594152722688392, -16.93181055722141792 ) ) ;
#37129=CARTESIAN_POINT ( 'NONE',  ( 63.69189222814998175, -69.76310523276724496, -16.89321520033831447 ) ) ;
#37131=CARTESIAN_POINT ( 'NONE',  ( 77.83157470812513168, -57.29119719338378047, -1.256939079640419843 ) ) ;
#37147=CARTESIAN_POINT ( 'NONE',  ( 113.6079577545248043, -7.250697342233347165, -7.631215200338321125 ) ) ;
#37149=CARTESIAN_POINT ( 'NONE',  ( 87.44708369096655076, -22.59602017601539359, -8.393215200338321580 ) ) ;
#37150=CARTESIAN_POINT ( 'NONE',  ( 64.34483944462449756, -36.50333010661785238, -5.615903718745205886 ) ) ;
#37153=CARTESIAN_POINT ( 'NONE',  ( 61.76986277844709861, -39.32091226840162079, -7.393215200338315363 ) ) ;
#37156=CARTESIAN_POINT ( 'NONE',  ( 105.0652233795248378, -1.325403438956436419, -9.854619843455211026 ) ) ;
#37158=CARTESIAN_POINT ( 'NONE',  ( 114.8581140045248361, 0.1403307496149616695, -15.46607636864997204 ) ) ;
#37161=CARTESIAN_POINT ( 'NONE',  ( 110.5290004229301815, 0.1075849324168598464, -14.64321520033829671 ) ) ;
#37180=CARTESIAN_POINT ( 'NONE',  ( 113.0523327545247838, -2.477300249445798297, -19.15521520033831138 ) ) ;
#37189=CARTESIAN_POINT ( 'NONE',  ( 106.3153796295248412, -4.863998795839590272, -19.15521520033831493 ) ) ;
#37194=( BOUNDED_SURFACE ( )  B_SPLINE_SURFACE ( 1, 2, ( 
 ( #1107, #29379, #15025, #28935, #43291, #12061, #25962, #39868, #42843, #8633, #36430, #15243, #5198, #29151, #11603, #19117, #8183, #25514, #22092, #35979, #9085, #33908, #19795, #9768, #22987, #12287, #37335, #33679, #2909, #5427, #16839, #26185, #19344, #40093, #40551, #41014, #44205, #2455, #2679, #27092, #26637, #20026, #12735, #23679, #30058, #16153, #36877, #23450, #16610, #33231, #40777, #30279, #16377, #30732, #6106, #13191, #19567, #8853, #2224, #37569, #22754, #2004, #5873, #30503, #44424, #36654, #12966, #9311, #15930, #26862, #6338, #20254, #43971, #34140, #29828, #43744, #23220, #37099, #12513, #26411, #9534, #40321, #5647, #33445, #28217, #30957, #35244, #17719, #10662, #17943, #31175, #38452, #37790, #4021, #27547, #10884, #17285, #45096, #7013, #34361, #14298, #34582, #42124, #24567, #38019, #24782, #38232, #14076, #44655, #31617, #7223, #38673, #7440, #3143, #13418, #44881, #17492, #21136, #13637, #21361, #3365, #35011, #3793, #27322, #41238, #9998, #23907, #386, #10218, #6564, #20481, #31390, #6795, #17064, #41459, #24126, #20704, #13853, #27767, #41681, #24347, #10442, #20923, #34797, #3579, #160, #27994, #41899, #830, #14750, #32292, #11329, #18836, #42797, #8355, #14972, #39594, #15422, #1502, #1056, #4479 ),
 ( #28884, #31842, #35931, #36153, #22259, #35704, #4922, #32728, #4249, #21810, #18399, #29327, #43241, #11558, #8136, #5146, #18166, #25465, #39369, #22037, #32063, #28662, #42567, #4698, #25687, #12006, #25909, #611, #18618, #39814, #25239, #8581, #32509, #1284, #22481, #15195, #21587, #29100, #43011, #14522, #36375, #11780, #28435, #42348, #11106, #25008, #38902, #39138, #7673, #35475, #7903, #26359, #29551, #5377, #27039, #12458, #19063, #32947, #36602, #43916, #44150, #12915, #26584, #40956, #40722, #12685, #33622, #33172, #1949, #19516, #43682, #6045, #30000, #9480, #2167, #26811, #2625, #33856, #33393, #36823, #40034, #19294, #16327, #12233, #37510, #16095, #8799, #40497, #9258, #23168, #19968, #40266, #22704, #23392, #15875, #1724, #37047, #15646, #29772, #16558, #30453, #9033, #5818, #19738, #2398, #22930, #5592, #30228, #44373, #37278, #13135, #9711, #23623, #43467, #26129, #14246, #44601, #23857, #13806, #13364, #9943, #17668, #34312, #17012, #41632, #3527, #3085, #3307, #6961, #27717, #17231, #34958, #37742, #42072, #24513, #17445, #24727, #37967, #113, #27269, #10830, #30903, #31564, #24074, #6743, #10388, #41182, #21081, #41412, #3746, #31339, #44825, #333, #45045, #20868, #6283, #38398, #14026, #28162, #20204, #6513 ) ),
 .UNSPECIFIED., .F., .F., .T. ) 
 B_SPLINE_SURFACE_WITH_KNOTS ( ( 2, 2 ),
 ( 3, 2, 2, 2, 2, 2, 2, 2, 2, 2, 2, 2, 2, 2, 2, 2, 2, 2, 2, 2, 2, 2, 2, 2, 2, 2, 2, 2, 2, 2, 2, 2, 2, 2, 2, 2, 2, 2, 2, 2, 2, 2, 2, 2, 2, 2, 2, 2, 2, 2, 2, 2, 2, 2, 2, 2, 2, 2, 2, 2, 2, 2, 2, 2, 2, 2, 2, 2, 2, 2, 2, 2, 2, 2, 2, 2, 2, 2, 2, 2, 3 ),
 ( 0.000000000000000000, 1.000000000000000000 ),
 ( 0.000000000000000000, 0.01250000000000000069, 0.02500000000000000139, 0.03749999999999999861, 0.05000000000000000278, 0.06250000000000000000, 0.07499999999999999722, 0.08749999999999999445, 0.1000000000000000056, 0.1125000000000000028, 0.1250000000000000000, 0.1375000000000000111, 0.1499999999999999944, 0.1625000000000000056, 0.1749999999999999889, 0.1875000000000000000, 0.2000000000000000111, 0.2124999999999999944, 0.2250000000000000056, 0.2374999999999999889, 0.2500000000000000000, 0.2625000000000000111, 0.2750000000000000222, 0.2874999999999999778, 0.2999999999999999889, 0.3125000000000000000, 0.3250000000000000111, 0.3375000000000000222, 0.3499999999999999778, 0.3624999999999999889, 0.3750000000000000000, 0.3875000000000000111, 0.4000000000000000222, 0.4124999999999999778, 0.4249999999999999889, 0.4375000000000000000, 0.4500000000000000111, 0.4625000000000000222, 0.4749999999999999778, 0.4874999999999999889, 0.5000000000000000000, 0.5124999999999999556, 0.5250000000000000222, 0.5374999999999999778, 0.5500000000000000444, 0.5625000000000000000, 0.5749999999999999556, 0.5875000000000000222, 0.5999999999999999778, 0.6125000000000000444, 0.6250000000000000000, 0.6374999999999999556, 0.6500000000000000222, 0.6624999999999999778, 0.6750000000000000444, 0.6875000000000000000, 0.6999999999999999556, 0.7125000000000000222, 0.7249999999999999778, 0.7375000000000000444, 0.7500000000000000000, 0.7624999999999999556, 0.7750000000000000222, 0.7874999999999999778, 0.8000000000000000444, 0.8125000000000000000, 0.8249999999999999556, 0.8375000000000000222, 0.8499999999999999778, 0.8625000000000000444, 0.8750000000000000000, 0.8874999999999999556, 0.9000000000000000222, 0.9124999999999999778, 0.9250000000000000444, 0.9375000000000000000, 0.9499999999999999556, 0.9625000000000000222, 0.9749999999999999778, 0.9875000000000000444, 1.000000000000000000 ),
 .UNSPECIFIED. ) 
 GEOMETRIC_REPRESENTATION_ITEM ( )  RATIONAL_B_SPLINE_SURFACE ( (
 ( 1.000000000000000000, 0.9238795325112869605, 1.000000000000000000, 0.9238795325112869605, 1.000000000000000000, 0.9238795325112869605, 1.000000000000000000, 0.9238795325112869605, 1.000000000000000000, 0.9238795325112869605, 1.000000000000000000, 0.9238795325112869605, 1.000000000000000000, 0.9238795325112869605, 1.000000000000000000, 0.9238795325112869605, 1.000000000000000000, 0.9238795325112869605, 1.000000000000000000, 0.9238795325112869605, 1.000000000000000000, 0.9238795325112869605, 1.000000000000000000, 0.9238795325112869605, 1.000000000000000000, 0.9238795325112869605, 1.000000000000000000, 0.9238795325112869605, 1.000000000000000000, 0.9238795325112869605, 1.000000000000000000, 0.9238795325112869605, 1.000000000000000000, 0.9238795325112869605, 1.000000000000000000, 0.9238795325112869605, 1.000000000000000000, 0.9238795325112869605, 1.000000000000000000, 0.9238795325112869605, 1.000000000000000000, 0.9238795325112869605, 1.000000000000000000, 0.9238795325112869605, 1.000000000000000000, 0.9238795325112869605, 1.000000000000000000, 0.9238795325112869605, 1.000000000000000000, 0.9238795325112869605, 1.000000000000000000, 0.9238795325112869605, 1.000000000000000000, 0.9238795325112869605, 1.000000000000000000, 0.9238795325112869605, 1.000000000000000000, 0.9238795325112869605, 1.000000000000000000, 0.9238795325112869605, 1.000000000000000000, 0.9238795325112869605, 1.000000000000000000, 0.9238795325112869605, 1.000000000000000000, 0.9238795325112869605, 1.000000000000000000, 0.9238795325112869605, 1.000000000000000000, 0.9238795325112869605, 1.000000000000000000, 0.9238795325112869605, 1.000000000000000000, 0.9238795325112869605, 1.000000000000000000, 0.9238795325112869605, 1.000000000000000000, 0.9238795325112869605, 1.000000000000000000, 0.9238795325112869605, 1.000000000000000000, 0.9238795325112869605, 1.000000000000000000, 0.9238795325112869605, 1.000000000000000000, 0.9238795325112869605, 1.000000000000000000, 0.9238795325112869605, 1.000000000000000000, 0.9238795325112869605, 1.000000000000000000, 0.9238795325112869605, 1.000000000000000000, 0.9238795325112869605, 1.000000000000000000, 0.9238795325112869605, 1.000000000000000000, 0.9238795325112869605, 1.000000000000000000, 0.9238795325112869605, 1.000000000000000000, 0.9238795325112869605, 1.000000000000000000, 0.9238795325112869605, 1.000000000000000000, 0.9238795325112869605, 1.000000000000000000, 0.9238795325112869605, 1.000000000000000000, 0.9238795325112869605, 1.000000000000000000, 0.9238795325112869605, 1.000000000000000000, 0.9238795325112869605, 1.000000000000000000, 0.9238795325112869605, 1.000000000000000000, 0.9238795325112869605, 1.000000000000000000, 0.9238795325112869605, 1.000000000000000000, 0.9238795325112869605, 1.000000000000000000, 0.9238795325112869605, 1.000000000000000000, 0.9238795325112869605, 1.000000000000000000, 0.9238795325112869605, 1.000000000000000000, 0.9238795325112869605, 1.000000000000000000, 0.9238795325112869605, 1.000000000000000000, 0.9238795325112869605, 1.000000000000000000, 0.9238795325112869605, 1.000000000000000000, 0.9238795325112869605, 1.000000000000000000, 0.9238795325112869605, 1.000000000000000000, 0.9238795325112869605, 1.000000000000000000, 0.9238795325112869605, 1.000000000000000000, 0.9238795325112869605, 1.000000000000000000, 0.9238795325112869605, 1.000000000000000000, 0.9238795325112869605, 1.000000000000000000, 0.9238795325112869605, 1.000000000000000000, 0.9238795325112869605, 1.000000000000000000, 0.9238795325112869605, 1.000000000000000000, 0.9238795325112869605, 1.000000000000000000, 0.9238795325112869605, 1.000000000000000000),
 ( 1.000000000000000000, 0.9238795325112869605, 1.000000000000000000, 0.9238795325112869605, 1.000000000000000000, 0.9238795325112869605, 1.000000000000000000, 0.9238795325112869605, 1.000000000000000000, 0.9238795325112869605, 1.000000000000000000, 0.9238795325112869605, 1.000000000000000000, 0.9238795325112869605, 1.000000000000000000, 0.9238795325112869605, 1.000000000000000000, 0.9238795325112869605, 1.000000000000000000, 0.9238795325112869605, 1.000000000000000000, 0.9238795325112869605, 1.000000000000000000, 0.9238795325112869605, 1.000000000000000000, 0.9238795325112869605, 1.000000000000000000, 0.9238795325112869605, 1.000000000000000000, 0.9238795325112869605, 1.000000000000000000, 0.9238795325112869605, 1.000000000000000000, 0.9238795325112869605, 1.000000000000000000, 0.9238795325112869605, 1.000000000000000000, 0.9238795325112869605, 1.000000000000000000, 0.9238795325112869605, 1.000000000000000000, 0.9238795325112869605, 1.000000000000000000, 0.9238795325112869605, 1.000000000000000000, 0.9238795325112869605, 1.000000000000000000, 0.9238795325112869605, 1.000000000000000000, 0.9238795325112869605, 1.000000000000000000, 0.9238795325112869605, 1.000000000000000000, 0.9238795325112869605, 1.000000000000000000, 0.9238795325112869605, 1.000000000000000000, 0.9238795325112869605, 1.000000000000000000, 0.9238795325112869605, 1.000000000000000000, 0.9238795325112869605, 1.000000000000000000, 0.9238795325112869605, 1.000000000000000000, 0.9238795325112869605, 1.000000000000000000, 0.9238795325112869605, 1.000000000000000000, 0.9238795325112869605, 1.000000000000000000, 0.9238795325112869605, 1.000000000000000000, 0.9238795325112869605, 1.000000000000000000, 0.9238795325112869605, 1.000000000000000000, 0.9238795325112869605, 1.000000000000000000, 0.9238795325112869605, 1.000000000000000000, 0.9238795325112869605, 1.000000000000000000, 0.9238795325112869605, 1.000000000000000000, 0.9238795325112869605, 1.000000000000000000, 0.9238795325112869605, 1.000000000000000000, 0.9238795325112869605, 1.000000000000000000, 0.9238795325112869605, 1.000000000000000000, 0.9238795325112869605, 1.000000000000000000, 0.9238795325112869605, 1.000000000000000000, 0.9238795325112869605, 1.000000000000000000, 0.9238795325112869605, 1.000000000000000000, 0.9238795325112869605, 1.000000000000000000, 0.9238795325112869605, 1.000000000000000000, 0.9238795325112869605, 1.000000000000000000, 0.9238795325112869605, 1.000000000000000000, 0.9238795325112869605, 1.000000000000000000, 0.9238795325112869605, 1.000000000000000000, 0.9238795325112869605, 1.000000000000000000, 0.9238795325112869605, 1.000000000000000000, 0.9238795325112869605, 1.000000000000000000, 0.9238795325112869605, 1.000000000000000000, 0.9238795325112869605, 1.000000000000000000, 0.9238795325112869605, 1.000000000000000000, 0.9238795325112869605, 1.000000000000000000, 0.9238795325112869605, 1.000000000000000000, 0.9238795325112869605, 1.000000000000000000, 0.9238795325112869605, 1.000000000000000000, 0.9238795325112869605, 1.000000000000000000, 0.9238795325112869605, 1.000000000000000000, 0.9238795325112869605, 1.000000000000000000, 0.9238795325112869605, 1.000000000000000000, 0.9238795325112869605, 1.000000000000000000, 0.9238795325112869605, 1.000000000000000000, 0.9238795325112869605, 1.000000000000000000, 0.9238795325112869605, 1.000000000000000000, 0.9238795325112869605, 1.000000000000000000, 0.9238795325112869605, 1.000000000000000000, 0.9238795325112869605, 1.000000000000000000, 0.9238795325112869605, 1.000000000000000000, 0.9238795325112869605, 1.000000000000000000, 0.9238795325112869605, 1.000000000000000000) ) ) 
 REPRESENTATION_ITEM ( '' )  SURFACE ( )  );
#37197=EDGE_LOOP ( 'NONE', ( #31865, #41686, #28117, #8733, #1218 ) ) ;
#37201=CARTESIAN_POINT ( 'NONE',  ( 111.7327233795247849, -8.938348069036489818, -17.46756447353520159 ) ) ;
#37203=CARTESIAN_POINT ( 'NONE',  ( 114.3719421295247827, -9.868328341294093420, -13.39321520033831447 ) ) ;
#37204=CARTESIAN_POINT ( 'NONE',  ( 113.6774108795247997, -8.938348069036489818, -9.318865927141430916 ) ) ;
#37211=CARTESIAN_POINT ( 'NONE',  ( 105.7294421295247844, -9.051693226400931991, -21.39321520033831447 ) ) ;
#37216=LINE ( 'NONE', #5755, #43890 ) ;
#37218=ORIENTED_EDGE ( 'NONE', *, *, #7431, .T. ) ;
#37219=CARTESIAN_POINT ( 'NONE',  ( 90.41915846579418314, -16.87387181286558757, -4.893215200338314474 ) ) ;
#37222=CARTESIAN_POINT ( 'NONE',  ( 108.3989733795247759, -1.325403438956436419, -9.854619843455211026 ) ) ;
#37223=CARTESIAN_POINT ( 'NONE',  ( 111.0381921295247878, -9.868328341294093420, -13.39321520033831447 ) ) ;
#37225=CARTESIAN_POINT ( 'NONE',  ( 69.23661232544138500, -26.06570555932018962, -5.871568482255425714 ) ) ;
#37231=AXIS2_PLACEMENT_3D ( 'NONE', #29522, #12660, #12202 ) ;
#37242=CARTESIAN_POINT ( 'NONE',  ( 108.9545983795247821, -0.7896495226426338832, -9.318865927141430916 ) ) ;
#37246=CARTESIAN_POINT ( 'NONE',  ( 111.2465515045248168, -6.936859964151250502, -18.39754474579286025 ) ) ;
#37247=DIRECTION ( 'NONE',  ( -1.000000000000000000, 0.000000000000000000, 0.000000000000000000 ) ) ;
#37252=FACE_OUTER_BOUND ( 'NONE', #42721, .T. ) ;
#37259=CARTESIAN_POINT ( 'NONE',  ( 70.32328378357757970, -26.37807398378523160, -5.615903685620933672 ) ) ;
#37264=CARTESIAN_POINT ( 'NONE',  ( 114.5104504682427802, 0.5115630086001619059, -14.64321520033831447 ) ) ;
#37267=CARTESIAN_POINT ( 'NONE',  ( 107.2877233795247776, -1.325403438956436419, -9.854619843455211026 ) ) ;
#37268=EDGE_CURVE ( 'NONE', #14703, #30187, #2798, .T. ) ;
#37273=CARTESIAN_POINT ( 'NONE',  ( 113.6079577545248043, -2.791137627527939813, -18.39754474579286025 ) ) ;
#37278=CARTESIAN_POINT ( 'NONE',  ( 109.0240515045248202, -2.477300249445798297, -7.631215200338321125 ) ) ;
#37280=CARTESIAN_POINT ( 'NONE',  ( 114.1635827545248389, -2.477300249445798297, -19.15521520033831138 ) ) ;
#37283=CARTESIAN_POINT ( 'NONE',  ( 115.4451630180080883, 0.7607806665037644134, -14.64321520033834467 ) ) ;
#37299=VECTOR ( 'NONE', #44991, 1000.000000000000000 ) ;
#37300=CARTESIAN_POINT ( 'NONE',  ( 109.5796765045248122, -7.250697342233347165, -19.15521520033831138 ) ) ;
#37302=CARTESIAN_POINT ( 'NONE',  ( 109.3018640045248304, 0.1403307496149616695, -15.46607636864997204 ) ) ;
#37305=CARTESIAN_POINT ( 'NONE',  ( 116.4555358795247884, -0.7896495226426338832, -17.46756447353520159 ) ) ;
#37306=ORIENTED_EDGE ( 'NONE', *, *, #9789, .F. ) ;
#37307=CARTESIAN_POINT ( 'NONE',  ( 78.69189222814998175, -69.76310523276724496, -16.89321520033831447 ) ) ;
#37311=CARTESIAN_POINT ( 'NONE',  ( 116.7696035360916227, 2.027398920889790457, -5.931029822836547005 ) ) ;
#37313=CARTESIAN_POINT ( 'NONE',  ( 106.3153796295248412, -4.863998795839590272, -8.388885654883775800 ) ) ;
#37316=CARTESIAN_POINT ( 'NONE',  ( 115.7145311052981782, 0.4930828106259610433, -12.14321520033831625 ) ) ;
#37320=EDGE_LOOP ( 'NONE', ( #6207, #32212, #9402, #25247 ) ) ;
#37328=CARTESIAN_POINT ( 'NONE',  ( 110.6909265045248247, -7.250697342233347165, -19.15521520033831138 ) ) ;
#37330=CARTESIAN_POINT ( 'NONE',  ( 61.76986277844709861, -39.32091226840162079, -21.89321520033831447 ) ) ;
#37334=LINE ( 'NONE', #33678, #19700 ) ;
#37335=CARTESIAN_POINT ( 'NONE',  ( 115.3442858795247759, -8.402594152722688392, -9.854619843455216355 ) ) ;
#37336=ORIENTED_EDGE ( 'NONE', *, *, #8638, .F. ) ;
#37337=LINE ( 'NONE', #27094, #36392 ) ;
#37339=CARTESIAN_POINT ( 'NONE',  ( 79.39832680986421565, 5.045790854648893209, -6.299625027019903456 ) ) ;
#37355=CARTESIAN_POINT ( 'NONE',  ( 110.6909265045248247, -2.791137627527939813, -8.388885654883777576 ) ) ;
#37358=ORIENTED_EDGE ( 'NONE', *, *, #1650, .T. ) ;
#37364=ORIENTED_EDGE ( 'NONE', *, *, #9273, .T. ) ;
#37365=CIRCLE ( 'NONE', #14072, 5.000000000000000888 ) ;
#37374=FACE_OUTER_BOUND ( 'NONE', #8228, .T. ) ;
#37386=CARTESIAN_POINT ( 'NONE',  ( 112.0105358795247810, -0.7896495226426338832, -17.46756447353520159 ) ) ;
#37396=ADVANCED_FACE ( 'NONE', ( #10692 ), #28244, .F. ) ;
#37399=CARTESIAN_POINT ( 'NONE',  ( 114.7192077545248594, -2.791137627527939813, -18.39754474579286025 ) ) ;
#37417=ORIENTED_EDGE ( 'NONE', *, *, #40060, .F. ) ;
#37421=CARTESIAN_POINT ( 'NONE',  ( 110.6909265045248247, -7.250697342233347165, -19.15521520033831138 ) ) ;
#37428=CARTESIAN_POINT ( 'NONE',  ( 69.69189222814998175, -41.76310523276723785, -23.89321520033831803 ) ) ;
#37438=CARTESIAN_POINT ( 'NONE',  ( 116.5944421295247793, -4.863998795839590272, -13.39321520033831447 ) ) ;
#37440=CARTESIAN_POINT ( 'NONE',  ( 109.1629577545248395, -7.250697342233347165, -7.631215200338321125 ) ) ;
#37441=CARTESIAN_POINT ( 'NONE',  ( 111.5938171295247940, 0.1403307496149613920, -13.39321520033831447 ) ) ;
#37442=CARTESIAN_POINT ( 'NONE',  ( 106.3848327545248651, -2.477300249445798297, -19.15521520033831138 ) ) ;
#37448=CARTESIAN_POINT ( 'NONE',  ( 84.39081516114413262, -30.32262605124143562, -12.39321520033834645 ) ) ;
#37451=CARTESIAN_POINT ( 'NONE',  ( 83.86216108596053687, -32.76310523276723785, -23.89321520033831803 ) ) ;
#37455=CIRCLE ( 'NONE', #27289, 0.4999999999999981681 ) ;
#37460=CARTESIAN_POINT ( 'NONE',  ( 107.9128015045248219, -6.936859964151250502, -18.39754474579286025 ) ) ;
#37461=CARTESIAN_POINT ( 'NONE',  ( 110.3436608795247764, -1.325403438956436419, -16.93181055722141792 ) ) ;
#37471=EDGE_CURVE ( 'NONE', #14403, #40384, #39302, .T. ) ;
#37474=DIRECTION ( 'NONE',  ( -2.439015257082815255E-15, 1.000000000000000000, 0.000000000000000000 ) ) ;
#37481=VERTEX_POINT ( 'NONE', #36404 ) ;
#37482=CARTESIAN_POINT ( 'NONE',  ( 116.5564130180080866, 0.7607806665037644134, -14.64321520033833401 ) ) ;
#37484=CARTESIAN_POINT ( 'NONE',  ( 108.7462390045248242, -9.868328341294098749, -11.32035403202665869 ) ) ;
#37493=CARTESIAN_POINT ( 'NONE',  ( 116.3631031537514815, 0.4930828106259610433, -14.64321520033831447 ) ) ;
#37494=CARTESIAN_POINT ( 'NONE',  ( 112.7745202545247736, -10.62599879583958540, -15.77991374673208469 ) ) ;
#37496=CARTESIAN_POINT ( 'NONE',  ( 68.68839935636916039, -25.95913848132418522, -5.893215200338315363 ) ) ;
#37501=DIRECTION ( 'NONE',  ( 0.3445294493088594256, 0.9387755102040817867, 0.000000000000000000 ) ) ;
#37502=CARTESIAN_POINT ( 'NONE',  ( 106.0375671295248310, 0.1403307496149613920, -13.39321520033831447 ) ) ;
#37506=CARTESIAN_POINT ( 'NONE',  ( 115.6220983795247861, -8.402594152722688392, -16.93181055722141792 ) ) ;
#37510=CARTESIAN_POINT ( 'NONE',  ( 110.7603796295247918, -4.863998795839590272, -19.15521520033831493 ) ) ;
#37511=DIRECTION ( 'NONE',  ( 0.000000000000000000, 0.000000000000000000, -1.000000000000000000 ) ) ;
#37512=CARTESIAN_POINT ( 'NONE',  ( 113.2606921295247702, 0.8980012041604618078, -13.39321520033831447 ) ) ;
#37528=CIRCLE ( 'NONE', #17871, 8.000000000000000000 ) ;
#37529=CARTESIAN_POINT ( 'NONE',  ( 105.5513952545248060, 0.8980012041604421569, -11.00651665394454071 ) ) ;
#37530=CARTESIAN_POINT ( 'NONE',  ( 108.8851452545248151, -9.868328341294098749, -15.46607636864997204 ) ) ;
#37533=CARTESIAN_POINT ( 'NONE',  ( 114.0246765045248196, -7.250697342233347165, -19.15521520033831138 ) ) ;
#37534=ORIENTED_EDGE ( 'NONE', *, *, #41046, .T. ) ;
#37535=DIRECTION ( 'NONE',  ( -0.9659258262890689783, -0.2588190451025185190, 0.000000000000000000 ) ) ;
#37540=VECTOR ( 'NONE', #33853, 1000.000000000000114 ) ;
#37542=CARTESIAN_POINT ( 'NONE',  ( 106.2459265045248173, -2.791137627527939813, -8.388885654883777576 ) ) ;
#37562=CARTESIAN_POINT ( 'NONE',  ( 111.3160046295247838, -4.863998795839590272, -7.631215200338315796 ) ) ;
#37563=CARTESIAN_POINT ( 'NONE',  ( 69.69189222814998175, -41.76310523276723785, -47.71602681600972318 ) ) ;
#37569=CARTESIAN_POINT ( 'NONE',  ( 113.0523327545247838, -6.936859964151250502, -8.388885654883777576 ) ) ;
#37570=EDGE_LOOP ( 'NONE', ( #25034, #11910, #39746, #41250 ) ) ;
#37571=CARTESIAN_POINT ( 'NONE',  ( 109.2294422423184272, -0.4618089760604071059, -15.91181704383022932 ) ) ;
#37589=CARTESIAN_POINT ( 'NONE',  ( 106.9404577545248145, -2.791137627527939813, -18.39754474579286025 ) ) ;
#37591=DIRECTION ( 'NONE',  ( 0.000000000000000000, -1.000000000000000000, 0.000000000000000000 ) ) ;
#37594=ADVANCED_FACE ( 'NONE', ( #15452 ), #36186, .F. ) ;
#37595=CIRCLE ( 'NONE', #39052, 1.000000000000000888 ) ;
#37601=DIRECTION ( 'NONE',  ( -1.000000000000000000, 0.000000000000000000, 0.000000000000000000 ) ) ;
#37603=CARTESIAN_POINT ( 'NONE',  ( 78.63502652544006821, -59.11697439676735399, 0.04365315361115504333 ) ) ;
#37605=FACE_OUTER_BOUND ( 'NONE', #21504, .T. ) ;
#37618=CARTESIAN_POINT ( 'NONE',  ( 109.6491296295247793, -4.863998795839590272, -19.15521520033831493 ) ) ;
#37620=CARTESIAN_POINT ( 'NONE',  ( 105.6208483795248299, -8.402594152722688392, -16.93181055722141792 ) ) ;
#37621=CARTESIAN_POINT ( 'NONE',  ( 106.1764733795248219, -1.325403438956436419, -9.854619843455211026 ) ) ;
#37622=CARTESIAN_POINT ( 'NONE',  ( 109.7880358795247986, -0.7896495226426338832, -17.46756447353518382 ) ) ;
#37626=FACE_OUTER_BOUND ( 'NONE', #12337, .T. ) ;
#37631=CARTESIAN_POINT ( 'NONE',  ( 107.3571765045248299, -7.250697342233347165, -19.15521520033831138 ) ) ;
#37633=ORIENTED_EDGE ( 'NONE', *, *, #28346, .F. ) ;
#37643=DIRECTION ( 'NONE',  ( 0.3445294493088594256, 0.9387755102040817867, 2.035644895278904423E-16 ) ) ;
#37651=CARTESIAN_POINT ( 'NONE',  ( 110.4825671295247815, -10.62599879583958540, -13.39321520033831447 ) ) ;
#37664=LINE ( 'NONE', #16703, #30260 ) ;
#37673=CARTESIAN_POINT ( 'NONE',  ( 107.1488171295247867, -10.62599879583958540, -13.39321520033831447 ) ) ;
#37674=CARTESIAN_POINT ( 'NONE',  ( 112.7745202545247878, 0.1403307496149616695, -11.32035403202665336 ) ) ;
#37675=CARTESIAN_POINT ( 'NONE',  ( 108.5378796295247810, -4.863998795839590272, -19.15521520033831493 ) ) ;
#37681=FACE_OUTER_BOUND ( 'NONE', #28966, .T. ) ;
#37683=EDGE_CURVE ( 'NONE', #816, #29699, #21285, .T. ) ;
#37689=CARTESIAN_POINT ( 'NONE',  ( 107.3571765045248299, -7.250697342233347165, -19.15521520033831138 ) ) ;
#37694=CARTESIAN_POINT ( 'NONE',  ( 109.3018640045248304, 0.1403307496149616695, -15.46607636864997204 ) ) ;
#37695=CARTESIAN_POINT ( 'NONE',  ( 107.1488171295248861, 0.1403307496149613920, -13.39321520033831447 ) ) ;
#37697=CARTESIAN_POINT ( 'NONE',  ( 68.68839935636917460, -25.95913848132418522, -5.893215200338315363 ) ) ;
#37700=VERTEX_POINT ( 'NONE', #20899 ) ;
#37706=VERTEX_POINT ( 'NONE', #360 ) ;
#37717=CARTESIAN_POINT ( 'NONE',  ( 115.8999108795247821, -8.938348069036489818, -9.318865927141430916 ) ) ;
#37723=CARTESIAN_POINT ( 'NONE',  ( 77.77634386988368931, 3.254514819260763581, -12.14321520033831625 ) ) ;
#37725=CARTESIAN_POINT ( 'NONE',  ( 112.6356140045247827, -10.62599879583958540, -11.00651665394455492 ) ) ;
#37728=DIRECTION ( 'NONE',  ( -0.3445294493088594256, -0.9387755102040817867, 0.000000000000000000 ) ) ;
#37729=EDGE_CURVE ( 'NONE', #1801, #21278, #33890, .T. ) ;
#37734=CARTESIAN_POINT ( 'NONE',  ( 114.0941296295247867, -4.863998795839590272, -19.15521520033831493 ) ) ;
#37737=CARTESIAN_POINT ( 'NONE',  ( 63.27883505452616930, -30.76310523276723785, -21.89321520033831447 ) ) ;
#37738=CARTESIAN_POINT ( 'NONE',  ( 113.9552233795247815, -1.325403438956436419, -9.854619843455211026 ) ) ;
#37742=CARTESIAN_POINT ( 'NONE',  ( 107.4266296295248821, -4.863998795839590272, -19.15521520033831493 ) ) ;
#37745=CARTESIAN_POINT ( 'NONE',  ( 113.8857702545248003, -10.62599879583958717, -15.77991374673208469 ) ) ;
#37748=CARTESIAN_POINT ( 'NONE',  ( 114.9275671295247889, -10.62599879583958540, -13.39321520033831625 ) ) ;
#37759=( BOUNDED_CURVE ( )  B_SPLINE_CURVE ( 2, ( #37942, #27692, #2600, #6489, #34503, #3504, #34064, #6716, #6020, #19943, #10364, #3282, #17421, #17204, #27243, #31097, #2830 ),
 .UNSPECIFIED., .F., .F. ) 
 B_SPLINE_CURVE_WITH_KNOTS ( ( 3, 2, 2, 2, 2, 2, 2, 2, 3 ),
 ( 0.004043115603494570193, 0.01250000000000000069, 0.02500000000000000139, 0.03750000000000000555, 0.05000000000000000278, 0.06250000000000000000, 0.07499999999999999722, 0.08749999999999999445, 0.09595688439650570944 ),
 .UNSPECIFIED. ) 
 CURVE ( )  GEOMETRIC_REPRESENTATION_ITEM ( )  RATIONAL_B_SPLINE_CURVE ( ( 0.9666851417651740608, 0.9485006404992000206, 1.000000000000000000, 0.9238795325112869605, 1.000000000000000000, 0.9238795325112869605, 1.000000000000000000, 0.9238795325112869605, 1.000000000000000000, 0.9238795325112869605, 1.000000000000000000, 0.9238795325112869605, 1.000000000000000000, 0.9238795325112869605, 1.000000000000000000, 0.9485006404991980222, 0.9666851417651760592 ) ) 
 REPRESENTATION_ITEM ( '' )  );
#37763=CARTESIAN_POINT ( 'NONE',  ( 112.6356140045247827, -10.62599879583958717, -11.00651665394454604 ) ) ;
#37767=CARTESIAN_POINT ( 'NONE',  ( 79.79010115959992788, 5.106172230548961188, -6.893215200338315363 ) ) ;
#37768=CARTESIAN_POINT ( 'NONE',  ( 116.5856851890968642, 2.159773802720716951, -6.182123076206457846 ) ) ;
#37770=CARTESIAN_POINT ( 'NONE',  ( 105.2041296295248287, -4.863998795839590272, -8.388885654883775800 ) ) ;
#37777=ORIENTED_EDGE ( 'NONE', *, *, #33649, .F. ) ;
#37783=CARTESIAN_POINT ( 'NONE',  ( 110.4825671295247815, -10.62599879583958540, -13.39321520033831447 ) ) ;
#37784=CARTESIAN_POINT ( 'NONE',  ( 105.8986608795248401, -1.325403438956436419, -16.93181055722141792 ) ) ;
#37785=CARTESIAN_POINT ( 'NONE',  ( 115.6220983795247861, -0.7896495226426338832, -9.318865927141430916 ) ) ;
#37790=CARTESIAN_POINT ( 'NONE',  ( 110.7603796295247918, -4.863998795839590272, -8.388885654883775800 ) ) ;
#37802=( NAMED_UNIT ( * ) SI_UNIT ( $, .STERADIAN. ) SOLID_ANGLE_UNIT ( ) );
#37804=AXIS2_PLACEMENT_3D ( 'NONE', #24715, #31997, #760 ) ;
#37807=CARTESIAN_POINT ( 'NONE',  ( 116.1777233795247781, -8.938348069036489818, -17.46756447353520159 ) ) ;
#37809=CARTESIAN_POINT ( 'NONE',  ( 69.90440230179062553, -25.79449873085293987, -5.893215200338315363 ) ) ;
#37824=CARTESIAN_POINT ( 'NONE',  ( 109.2294421295247844, 0.8460904216231607267, -14.64321520033831447 ) ) ;
#37834=CARTESIAN_POINT ( 'NONE',  ( 106.6626452545248611, 0.8980012041604421569, -11.00651665394454071 ) ) ;
#37836=CYLINDRICAL_SURFACE ( 'NONE', #24085, 5.000000000000004441 ) ;
#37840=ORIENTED_EDGE ( 'NONE', *, *, #15053, .T. ) ;
#37841=VECTOR ( 'NONE', #22183, 1000.000000000000114 ) ;
#37848=CARTESIAN_POINT ( 'NONE',  ( 106.0375671295248310, -10.62599879583958540, -13.39321520033831447 ) ) ;
#37851=FACE_OUTER_BOUND ( 'NONE', #38964, .T. ) ;
#37855=CARTESIAN_POINT ( 'NONE',  ( 70.19189222814998175, -75.31442247550839397, -37.94335727672635983 ) ) ;
#37860=ORIENTED_EDGE ( 'NONE', *, *, #15081, .F. ) ;
#37862=DIRECTION ( 'NONE',  ( 0.000000000000000000, 0.000000000000000000, -1.000000000000000000 ) ) ;
#37872=CARTESIAN_POINT ( 'NONE',  ( 107.0793640045248196, -10.62599879583958717, -11.00651665394454604 ) ) ;
#37876=AXIS2_PLACEMENT_3D ( 'NONE', #15423, #29328, #1725 ) ;
#37879=APPLICATION_CONTEXT ( 'automotive_design' ) ;
#37880=PLANE ( 'NONE',  #36044 ) ;
#37893=CARTESIAN_POINT ( 'NONE',  ( 107.2182702545248105, -10.62599879583958717, -15.77991374673208469 ) ) ;
#37894=CARTESIAN_POINT ( 'NONE',  ( 108.5378796295247810, -4.863998795839590272, -8.388885654883775800 ) ) ;
#37895=CARTESIAN_POINT ( 'NONE',  ( 109.0935046295247872, -4.863998795839590272, -7.631215200338315796 ) ) ;
#37901=CARTESIAN_POINT ( 'NONE',  ( 112.2883483795247770, -0.7896495226426338832, -9.318865927141430916 ) ) ;
#37908=CARTESIAN_POINT ( 'NONE',  ( 115.6915515045247531, -6.936859964151250502, -18.39754474579286025 ) ) ;
#37914=CARTESIAN_POINT ( 'NONE',  ( 108.1211608795247798, -1.325403438956436419, -16.93181055722141792 ) ) ;
#37915=CARTESIAN_POINT ( 'NONE',  ( 105.6903015045248253, -6.936859964151250502, -18.39754474579286025 ) ) ;
#37916=VECTOR ( 'NONE', #15873, 1000.000000000000000 ) ;
#37930=ADVANCED_FACE ( 'NONE', ( #22453 ), #11532, .F. ) ;
#37940=CARTESIAN_POINT ( 'NONE',  ( 115.6915515045247531, -2.477300249445798297, -7.631215200338321125 ) ) ;
#37942=CARTESIAN_POINT ( 'NONE',  ( 115.9947331777918862, -0.01829820670803256055, -14.64321520033831447 ) ) ;
#37947=EDGE_LOOP ( 'NONE', ( #25515, #4345, #23974, #2937 ) ) ;
#37952=CARTESIAN_POINT ( 'NONE',  ( 65.34289968162609341, -37.75951406093616214, -4.893215200338314474 ) ) ;
#37958=CARTESIAN_POINT ( 'NONE',  ( 107.4266296295248821, -4.863998795839590272, -8.388885654883775800 ) ) ;
#37962=CARTESIAN_POINT ( 'NONE',  ( 110.4131140045248287, 0.1403307496149616695, -15.46607636864997204 ) ) ;
#37964=CARTESIAN_POINT ( 'NONE',  ( 62.92618109310924268, -32.76310523276723785, -23.89321520033831803 ) ) ;
#37967=CARTESIAN_POINT ( 'NONE',  ( 107.0793640045248196, -10.62599879583958717, -11.00651665394454604 ) ) ;
#37969=CARTESIAN_POINT ( 'NONE',  ( 108.5378796295247810, -4.863998795839590272, -19.15521520033831493 ) ) ;
#37972=CARTESIAN_POINT ( 'NONE',  ( 111.9181031537514741, 0.4930828106259610433, -14.64321520033831447 ) ) ;
#37975=EDGE_CURVE ( 'NONE', #2531, #23514, #42984, .T. ) ;
#37985=ADVANCED_FACE ( 'NONE', ( #8329 ), #4451, .F. ) ;
#37987=CARTESIAN_POINT ( 'NONE',  ( 116.8583982284553144, -0.4292963591166082393, -16.22917518106288881 ) ) ;
#37988=CARTESIAN_POINT ( 'NONE',  ( 113.9552233795247815, -8.938348069036489818, -17.46756447353520159 ) ) ;
#37989=ORIENTED_EDGE ( 'NONE', *, *, #6249, .T. ) ;
#37992=CARTESIAN_POINT ( 'NONE',  ( 116.1777233795247781, -1.325403438956436419, -9.854619843455211026 ) ) ;
#37995=CARTESIAN_POINT ( 'NONE',  ( 117.0736591576486774, 1.652729585752748198, -5.467741361931248711 ) ) ;
#37997=CARTESIAN_POINT ( 'NONE',  ( 107.7044421295247929, -9.868328341294093420, -13.39321520033831447 ) ) ;
#38006=EDGE_LOOP ( 'NONE', ( #7516, #14013, #12521, #6428 ) ) ;
#38009=CARTESIAN_POINT ( 'NONE',  ( 117.0806140045248185, 0.1403307496149616695, -15.46607636864997204 ) ) ;
#38012=CARTESIAN_POINT ( 'NONE',  ( 111.3854577545248645, -7.250697342233347165, -7.631215200338321125 ) ) ;
#38013=CARTESIAN_POINT ( 'NONE',  ( 105.4819421295248247, -9.868328341294093420, -13.39321520033831447 ) ) ;
#38014=CARTESIAN_POINT ( 'NONE',  ( 82.84471951188260164, -31.80328994127697939, -23.17386122141205718 ) ) ;
#38017=DIRECTION ( 'NONE',  ( 0.000000000000000000, 0.000000000000000000, -1.000000000000000000 ) ) ;
#38019=CARTESIAN_POINT ( 'NONE',  ( 109.9269421295247753, -9.868328341294093420, -13.39321520033831447 ) ) ;
#38028=VECTOR ( 'NONE', #20474, 1000.000000000000114 ) ;
#38034=CARTESIAN_POINT ( 'NONE',  ( 107.7044421295247929, -9.868328341294093420, -13.39321520033831447 ) ) ;
#38044=CARTESIAN_POINT ( 'NONE',  ( 114.3024890045248156, 0.8980012041604421569, -15.77991374673208469 ) ) ;
#38048=CARTESIAN_POINT ( 'NONE',  ( 78.02189457680029250, -57.61239323309698790, -1.007362850241582786 ) ) ;
#38050=CARTESIAN_POINT ( 'NONE',  ( 66.06194382436763135, -14.97931106434683635, -21.89321520033831447 ) ) ;
#38061=CARTESIAN_POINT ( 'NONE',  ( 109.5796765045248122, -7.250697342233347165, -19.15521520033831138 ) ) ;
#38062=CARTESIAN_POINT ( 'NONE',  ( 105.7597546295248350, -4.863998795839590272, -18.39754474579285315 ) ) ;
#38064=DIRECTION ( 'NONE',  ( 1.000000000000000000, 0.000000000000000000, 0.000000000000000000 ) ) ;
#38072=CARTESIAN_POINT ( 'NONE',  ( 111.6632702545248605, 0.1403307496149616695, -11.32035403202665336 ) ) ;
#38075=FACE_OUTER_BOUND ( 'NONE', #2234, .T. ) ;
#38084=AXIS2_PLACEMENT_3D ( 'NONE', #23277, #9144, #16217 ) ;
#38085=CARTESIAN_POINT ( 'NONE',  ( 116.5945891742730822, -9.863394354262339903, -13.30644683333167855 ) ) ;
#38093=CARTESIAN_POINT ( 'NONE',  ( 106.7320983795247855, -0.7896495226426338832, -9.318865927141430916 ) ) ;
#38101=DIRECTION ( 'NONE',  ( 0.000000000000000000, -0.7142857142857143016, 0.6998542122237653151 ) ) ;
#38111=EDGE_CURVE ( 'NONE', #32144, #18453, #37664, .T. ) ;
#38113=CARTESIAN_POINT ( 'NONE',  ( 107.6349890045248401, 0.8980012041604421569, -15.77991374673208469 ) ) ;
#38115=CARTESIAN_POINT ( 'NONE',  ( 108.8851452545248151, -9.868328341294098749, -15.46607636864997204 ) ) ;
#38116=CARTESIAN_POINT ( 'NONE',  ( 106.1764733795248219, -8.938348069036489818, -17.46756447353520159 ) ) ;
#38122=CARTESIAN_POINT ( 'NONE',  ( 109.4407702545248355, -10.62599879583958717, -15.77991374673208469 ) ) ;
#38123=PLANE ( 'NONE',  #27074 ) ;
#38131=CARTESIAN_POINT ( 'NONE',  ( 106.5931921295248372, 0.8980012041604618078, -13.39321520033831447 ) ) ;
#38137=CARTESIAN_POINT ( 'NONE',  ( 113.8857702545248003, -10.62599879583958717, -15.77991374673208469 ) ) ;
#38138=CARTESIAN_POINT ( 'NONE',  ( 108.3989733795248753, -1.325403438956436419, -9.854619843455211026 ) ) ;
#38142=ORIENTED_EDGE ( 'NONE', *, *, #19698, .F. ) ;
#38144=CYLINDRICAL_SURFACE ( 'NONE', #16417, 1.299999999999995604 ) ;
#38159=CARTESIAN_POINT ( 'NONE',  ( 107.0793640045248196, 0.1403307496149616695, -15.46607636864997204 ) ) ;
#38173=CARTESIAN_POINT ( 'NONE',  ( 116.0388171295248014, -10.62599879583958540, -13.39321520033831447 ) ) ;
#38179=CARTESIAN_POINT ( 'NONE',  ( 112.5661608795247872, -1.325403438956436419, -16.93181055722138595 ) ) ;
#38180=CARTESIAN_POINT ( 'NONE',  ( 111.4549108795247747, -1.325403438956436419, -16.93181055722141792 ) ) ;
#38182=CARTESIAN_POINT ( 'NONE',  ( 109.2294422726160974, -7.213534936028837663, -18.14492746615356822 ) ) ;
#38184=LINE ( 'NONE', #34746, #40789 ) ;
#38186=CARTESIAN_POINT ( 'NONE',  ( 110.1353015045248469, -2.477300249445798297, -7.631215200338321125 ) ) ;
#38202=CARTESIAN_POINT ( 'NONE',  ( 115.5526452545247622, 0.8980012041604421569, -11.00651665394454071 ) ) ;
#38203=ORIENTED_EDGE ( 'NONE', *, *, #22524, .F. ) ;
#38206=CARTESIAN_POINT ( 'NONE',  ( 112.7515004229301780, 0.1075849324168598464, -14.64321520033831447 ) ) ;
#38212=EDGE_CURVE ( 'NONE', #32422, #38815, #7666, .T. ) ;
#38213=DIRECTION ( 'NONE',  ( -0.1736481776669309696, -0.9848077530122079093, 0.000000000000000000 ) ) ;
#38214=CARTESIAN_POINT ( 'NONE',  ( 116.2471765045247594, -2.791137627527939813, -8.388885654883777576 ) ) ;
#38219=ORIENTED_EDGE ( 'NONE', *, *, #23071, .F. ) ;
#38225=CARTESIAN_POINT ( 'NONE',  ( 106.5237390045248418, -9.868328341294098749, -11.32035403202665869 ) ) ;
#38226=CARTESIAN_POINT ( 'NONE',  ( 114.7192077545248594, -7.250697342233347165, -7.631215200338321125 ) ) ;
#38230=CARTESIAN_POINT ( 'NONE',  ( 109.2294439017210550, -0.2843800758933193173, -10.66990552702273476 ) ) ;
#38232=CARTESIAN_POINT ( 'NONE',  ( 109.7880358795247986, -8.402594152722688392, -9.854619843455216355 ) ) ;
#38234=CARTESIAN_POINT ( 'NONE',  ( 69.69189222814998175, -41.76310523276723785, -24.89321520033831447 ) ) ;
#38247=CARTESIAN_POINT ( 'NONE',  ( 108.9545983795247821, -8.402594152722688392, -16.93181055722141792 ) ) ;
#38249=CARTESIAN_POINT ( 'NONE',  ( 83.84865386347668448, -25.99489077589588604, -15.39321520033831625 ) ) ;
#38250=ORIENTED_EDGE ( 'NONE', *, *, #30606, .T. ) ;
#38256=CARTESIAN_POINT ( 'NONE',  ( 114.6497546295247929, -4.863998795839590272, -7.631215200338315796 ) ) ;
#38273=CARTESIAN_POINT ( 'NONE',  ( 108.9545983795247821, -0.7896495226426338832, -9.318865927141430916 ) ) ;
#38278=CIRCLE ( 'NONE', #43374, 1.000000000000000888 ) ;
#38286=CARTESIAN_POINT ( 'NONE',  ( 113.7468640045248236, 0.1403307496149616695, -15.46607636864997204 ) ) ;
#38289=ORIENTED_EDGE ( 'NONE', *, *, #28401, .F. ) ;
#38294=CARTESIAN_POINT ( 'NONE',  ( 80.19189222814998175, -66.20485342690169261, -45.06987807991851724 ) ) ;
#38298=VERTEX_POINT ( 'NONE', #4336 ) ;
#38300=CARTESIAN_POINT ( 'NONE',  ( 116.5987716749792895, -9.866677412677834269, -13.52174868289714027 ) ) ;
#38308=CARTESIAN_POINT ( 'NONE',  ( 109.0240515045248202, -2.477300249445798297, -7.631215200338321125 ) ) ;
#38311=VERTEX_POINT ( 'NONE', #11426 ) ;
#38318=CARTESIAN_POINT ( 'NONE',  ( 79.72353890764954087, 4.236894767232761261, -12.14321520033831625 ) ) ;
#38326=ORIENTED_EDGE ( 'NONE', *, *, #4937, .F. ) ;
#38327=AXIS2_PLACEMENT_3D ( 'NONE', #16409, #27351, #44685 ) ;
#38329=CARTESIAN_POINT ( 'NONE',  ( 115.1359265045248605, -2.791137627527939813, -8.388885654883777576 ) ) ;
#38330=CARTESIAN_POINT ( 'NONE',  ( 110.6909265045248247, -2.791137627527939813, -8.388885654883777576 ) ) ;
#38331=CARTESIAN_POINT ( 'NONE',  ( 105.8986608795248401, -8.938348069036489818, -9.318865927141430916 ) ) ;
#38336=CARTESIAN_POINT ( 'NONE',  ( 113.6774108795247997, -8.938348069036489818, -9.318865927141430916 ) ) ;
#38337=CARTESIAN_POINT ( 'NONE',  ( 61.76986277844709861, -39.32091226840162079, -6.340220811149025693 ) ) ;
#38339=FACE_OUTER_BOUND ( 'NONE', #8039, .T. ) ;
#38342=CARTESIAN_POINT ( 'NONE',  ( 113.6079577545248043, -7.250697342233347165, -7.631215200338321125 ) ) ;
#38343=CARTESIAN_POINT ( 'NONE',  ( 115.2748327545248657, -6.936859964151250502, -8.388885654883777576 ) ) ;
#38345=CARTESIAN_POINT ( 'NONE',  ( 116.2659068881580708, -12.01880880694303855, -20.89321520033831447 ) ) ;
#38348=VECTOR ( 'NONE', #37474, 1000.000000000000000 ) ;
#38349=CARTESIAN_POINT ( 'NONE',  ( 113.6774108795247997, -8.938348069036489818, -9.318865927141430916 ) ) ;
#38350=CARTESIAN_POINT ( 'NONE',  ( 108.4684265045248424, -2.791137627527939813, -8.388885654883777576 ) ) ;
#38354=VERTEX_POINT ( 'NONE', #14840 ) ;
#38362=CARTESIAN_POINT ( 'NONE',  ( 108.7462390045248242, -9.868328341294098749, -11.32035403202665869 ) ) ;
#38372=CARTESIAN_POINT ( 'NONE',  ( 106.2459265045248173, -2.791137627527939813, -8.388885654883777576 ) ) ;
#38374=CARTESIAN_POINT ( 'NONE',  ( 117.2294421295248128, -10.91793254776207611, -21.88709314391948269 ) ) ;
#38378=ORIENTED_EDGE ( 'NONE', *, *, #24471, .T. ) ;
#38384=EDGE_LOOP ( 'NONE', ( #13512, #10176, #1115, #11062, #31360, #32676, #36678 ) ) ;
#38387=CARTESIAN_POINT ( 'NONE',  ( 109.9963952545248134, 0.8980012041604421569, -11.00651665394454071 ) ) ;
#38392=PLANE ( 'NONE',  #31510 ) ;
#38393=CARTESIAN_POINT ( 'NONE',  ( 110.6214733795247867, -1.325403438956436419, -9.854619843455211026 ) ) ;
#38396=CARTESIAN_POINT ( 'NONE',  ( 109.2294421683802312, -8.290612149491295213, -17.51551637747833468 ) ) ;
#38398=CARTESIAN_POINT ( 'NONE',  ( 105.7597546295248350, -4.863998795839590272, -7.631215200338315796 ) ) ;
#38399=CARTESIAN_POINT ( 'NONE',  ( 115.5526452545247622, -9.868328341294098749, -15.46607636864997204 ) ) ;
#38400=CARTESIAN_POINT ( 'NONE',  ( 110.8298327545248299, -2.477300249445798297, -19.15521520033831138 ) ) ;
#38404=( BOUNDED_CURVE ( )  B_SPLINE_CURVE ( 3, ( #15673, #18645, #39393, #29577 ),
 .UNSPECIFIED., .F., .F. ) 
 B_SPLINE_CURVE_WITH_KNOTS ( ( 4, 4 ),
 ( 0.000000000000000000, 3.141592653589795336 ),
 .UNSPECIFIED. ) 
 CURVE ( )  GEOMETRIC_REPRESENTATION_ITEM ( )  RATIONAL_B_SPLINE_CURVE ( ( 1.000000000000000000, 0.3333333333333335369, 0.3333333333333335369, 1.000000000000000000 ) ) 
 REPRESENTATION_ITEM ( '' )  );
#38405=ADVANCED_FACE ( 'NONE', ( #8221 ), #10752, .F. ) ;
#38413=AXIS2_PLACEMENT_3D ( 'NONE', #24476, #10358, #30648 ) ;
#38420=CARTESIAN_POINT ( 'NONE',  ( 115.6220983795247861, -0.7896495226426338832, -9.318865927141430916 ) ) ;
#38430=CARTESIAN_POINT ( 'NONE',  ( 104.9263171295248327, 0.1403307496149613920, -13.39321520033831447 ) ) ;
#38432=CARTESIAN_POINT ( 'NONE',  ( 116.5944421295247793, -9.868328341294093420, -13.39321520033831447 ) ) ;
#38439=ORIENTED_EDGE ( 'NONE', *, *, #9005, .T. ) ;
#38442=CARTESIAN_POINT ( 'NONE',  ( 114.8581140045248361, 0.1403307496149616695, -15.46607636864997204 ) ) ;
#38445=CARTESIAN_POINT ( 'NONE',  ( 86.09796674931440918, -26.99705449037680438, -8.518632518551283894 ) ) ;
#38446=CARTESIAN_POINT ( 'NONE',  ( 112.0799890045248475, 0.8980012041604421569, -15.77991374673208469 ) ) ;
#38449=CARTESIAN_POINT ( 'NONE',  ( 116.5965958012052539, -9.868328341294104078, -13.45749254416749174 ) ) ;
#38452=CARTESIAN_POINT ( 'NONE',  ( 110.8298327545248299, -6.936859964151250502, -8.388885654883777576 ) ) ;
#38456=CARTESIAN_POINT ( 'NONE',  ( 110.6214733795247867, -8.938348069036489818, -17.46756447353520159 ) ) ;
#38465=CARTESIAN_POINT ( 'NONE',  ( 107.5655358795247736, -8.402594152722688392, -9.854619843455216355 ) ) ;
#38473=CARTESIAN_POINT ( 'NONE',  ( 107.2182702545248105, 0.1403307496149616695, -11.32035403202665336 ) ) ;
#38478=DIRECTION ( 'NONE',  ( 0.000000000000000000, 0.000000000000000000, -1.000000000000000000 ) ) ;
#38479=ADVANCED_FACE ( 'NONE', ( #21453, #15062 ), #921, .F. ) ;
#38489=ORIENTED_EDGE ( 'NONE', *, *, #10952, .T. ) ;
#38491=CARTESIAN_POINT ( 'NONE',  ( 106.5237390045248418, 0.8980012041604421569, -15.77991374673208469 ) ) ;
#38493=CARTESIAN_POINT ( 'NONE',  ( 114.2330358795247776, -8.402594152722736354, -9.854619843455244776 ) ) ;
#38502=CARTESIAN_POINT ( 'NONE',  ( 111.1076452545248259, -9.868328341294098749, -15.46607636864997204 ) ) ;
#38512=DIRECTION ( 'NONE',  ( -2.439015257082815255E-15, 1.000000000000000000, 0.000000000000000000 ) ) ;
#38522=CARTESIAN_POINT ( 'NONE',  ( 105.8986608795248401, -8.938348069036489818, -9.318865927141430916 ) ) ;
#38531=CARTESIAN_POINT ( 'NONE',  ( 87.44708369096657918, -21.99489077589588604, -4.893215200338314474 ) ) ;
#38542=ORIENTED_EDGE ( 'NONE', *, *, #98, .T. ) ;
#38544=CARTESIAN_POINT ( 'NONE',  ( 112.8439733795247832, -1.325403438956436419, -9.854619843455211026 ) ) ;
#38545=CARTESIAN_POINT ( 'NONE',  ( 107.5655358795247736, -8.402594152722688392, -9.854619843455216355 ) ) ;
#38546=CARTESIAN_POINT ( 'NONE',  ( 112.0799890045248475, -9.868328341294098749, -11.32035403202665869 ) ) ;
#38552=CARTESIAN_POINT ( 'NONE',  ( 113.1217858795247935, -0.7896495226426338832, -17.46756447353520159 ) ) ;
#38553=CARTESIAN_POINT ( 'NONE',  ( 78.69189222814998175, -46.76310523276723785, -6.893215200338315363 ) ) ;
#38558=CARTESIAN_POINT ( 'NONE',  ( 112.6356140045247827, -10.62599879583958717, -11.00651665394454604 ) ) ;
#38559=CARTESIAN_POINT ( 'NONE',  ( 114.5108483795247878, -8.402594152722688392, -16.93181055722141792 ) ) ;
#38564=CIRCLE ( 'NONE', #18917, 5.132259260909280307 ) ;
#38565=CARTESIAN_POINT ( 'NONE',  ( 115.5526452545247622, 0.8980012041604421569, -11.00651665394454071 ) ) ;
#38566=CARTESIAN_POINT ( 'NONE',  ( 104.9957702545248566, 0.1403307496149616695, -11.32035403202665336 ) ) ;
#38575=VERTEX_POINT ( 'NONE', #38999 ) ;
#38579=CARTESIAN_POINT ( 'NONE',  ( 109.9963952545248134, -9.868328341294098749, -15.46607636864997204 ) ) ;
#38580=ORIENTED_EDGE ( 'NONE', *, *, #17301, .F. ) ;
#38585=EDGE_LOOP ( 'NONE', ( #10786, #29664 ) ) ;
#38588=CARTESIAN_POINT ( 'NONE',  ( 106.1070202545248407, 0.1403307496149616695, -11.32035403202665336 ) ) ;
#38590=B_SPLINE_CURVE_WITH_KNOTS ( 'NONE', 3,
 ( #44474, #23268, #43797, #41291, #9588, #34188, #40833, #9821, #37150, #40371, #16890, #30331, #20528, #19614, #33498, #15977, #34408, #2277 ),
 .UNSPECIFIED., .F., .F.,
 ( 4, 2, 2, 1, 1, 1, 1, 2, 2, 2, 4 ),
 ( 0.000000000000000000, 0.2500000000001928457, 0.3750000000002891021, 0.4375000000003371747, 0.4687500000003585465, 0.4843750000003703149, 0.4921875000003760325, 0.4960937500003751999, 0.5000000000003742562, 0.7500000000001871836, 1.000000000000000000 ),
 .UNSPECIFIED. ) ;
#38595=VERTEX_POINT ( 'NONE', #35108 ) ;
#38597=CARTESIAN_POINT ( 'NONE',  ( 116.2471765045247594, -7.250697342233347165, -19.15521520033831138 ) ) ;
#38598=CARTESIAN_POINT ( 'NONE',  ( 84.82510614249602554, -29.13926788429013470, -9.862835514873660614 ) ) ;
#38604=CARTESIAN_POINT ( 'NONE',  ( 109.6527889883689824, 0.3193521225029610777, -12.14321520033828072 ) ) ;
#38605=CARTESIAN_POINT ( 'NONE',  ( 109.6491296295247793, -4.863998795839590272, -19.15521520033831493 ) ) ;
#38610=CARTESIAN_POINT ( 'NONE',  ( 107.9128015045248219, -6.936859964151250502, -18.39754474579286025 ) ) ;
#38613=CARTESIAN_POINT ( 'NONE',  ( 109.2296097124207250, -8.834719573337491028, -17.03747813294903324 ) ) ;
#38616=CARTESIAN_POINT ( 'NONE',  ( 116.7333483795247844, -8.402594152722688392, -16.93181055722141792 ) ) ;
#38617=CARTESIAN_POINT ( 'NONE',  ( 108.8851452545248151, 0.8980012041604421569, -11.00651665394454071 ) ) ;
#38618=CARTESIAN_POINT ( 'NONE',  ( 70.36267391504958368, -5.685877709920885259, -21.89321520033831447 ) ) ;
#38624=ORIENTED_EDGE ( 'NONE', *, *, #42337, .T. ) ;
#38635=CARTESIAN_POINT ( 'NONE',  ( 110.4131140045248287, -10.62599879583958717, -11.00651665394454604 ) ) ;
#38647=CARTESIAN_POINT ( 'NONE',  ( 116.8722546295247895, -4.863998795839590272, -18.39754474579285315 ) ) ;
#38660=CARTESIAN_POINT ( 'NONE',  ( 114.3024890045248156, -9.868328341294098749, -11.32035403202665869 ) ) ;
#38662=( BOUNDED_CURVE ( )  B_SPLINE_CURVE ( 3, ( #34575, #2904, #14069, #30726 ),
 .UNSPECIFIED., .F., .T. ) 
 B_SPLINE_CURVE_WITH_KNOTS ( ( 4, 4 ),
 ( 0.2801472849774039875, 0.7487301044471339484 ),
 .UNSPECIFIED. ) 
 CURVE ( )  GEOMETRIC_REPRESENTATION_ITEM ( )  RATIONAL_B_SPLINE_CURVE ( ( 1.000000000000000000, 0.9817860582945869830, 0.9817860582945869830, 1.000000000000000000 ) ) 
 REPRESENTATION_ITEM ( '' )  );
#38665=CARTESIAN_POINT ( 'NONE',  ( 86.28794317325427699, -26.53699186446346658, -8.429793386229720298 ) ) ;
#38666=CARTESIAN_POINT ( 'NONE',  ( 111.6632702545248605, -10.62599879583958717, -15.77991374673208469 ) ) ;
#38671=CARTESIAN_POINT ( 'NONE',  ( 109.2294421335984111, -7.460416756848673003, -8.322835172996224884 ) ) ;
#38673=CARTESIAN_POINT ( 'NONE',  ( 109.4407702545248355, 0.1403307496149616695, -11.32035403202665336 ) ) ;
#38676=FACE_OUTER_BOUND ( 'NONE', #37947, .T. ) ;
#38679=CARTESIAN_POINT ( 'NONE',  ( 109.5796765045248122, -7.250697342233347165, -19.15521520033831138 ) ) ;
#38682=EDGE_CURVE ( 'NONE', #30525, #38595, #39011, .T. ) ;
#38691=CARTESIAN_POINT ( 'NONE',  ( 115.4137390045248566, 0.8980012041604421569, -15.77991374673208469 ) ) ;
#38699=VERTEX_POINT ( 'NONE', #37824 ) ;
#38700=CARTESIAN_POINT ( 'NONE',  ( 107.0099108795247815, -1.325403438956436419, -16.93181055722141792 ) ) ;
#38709=ADVANCED_FACE ( 'NONE', ( #16420 ), #34616, .T. ) ;
#38717=ORIENTED_EDGE ( 'NONE', *, *, #7486, .T. ) ;
#38719=CARTESIAN_POINT ( 'NONE',  ( 114.9275671295247889, 0.1403307496149613920, -13.39321520033831447 ) ) ;
#38721=CARTESIAN_POINT ( 'NONE',  ( 87.44708369096657918, -25.99489077589588604, -15.39321520033831625 ) ) ;
#38731=CARTESIAN_POINT ( 'NONE',  ( 110.6909265045248247, -2.791137627527939813, -8.388885654883777576 ) ) ;
#38733=EDGE_LOOP ( 'NONE', ( #43596, #15481, #18573, #33075 ) ) ;
#38738=ADVANCED_FACE ( 'NONE', ( #6831, #34396, #27582 ), #20736, .T. ) ;
#38752=VERTEX_POINT ( 'NONE', #10036 ) ;
#38755=CARTESIAN_POINT ( 'NONE',  ( 107.4266296295248821, -4.863998795839590272, -19.15521520033831493 ) ) ;
#38759=CARTESIAN_POINT ( 'NONE',  ( 87.44708369096657918, -21.99489077589588604, -20.89321520033831447 ) ) ;
#38773=VERTEX_POINT ( 'NONE', #3177 ) ;
#38778=CARTESIAN_POINT ( 'NONE',  ( 112.5661608795247872, -1.325403438956436419, -16.93181055722141792 ) ) ;
#38779=CARTESIAN_POINT ( 'NONE',  ( 109.6491296295247793, -4.863998795839590272, -8.388885654883775800 ) ) ;
#38780=CARTESIAN_POINT ( 'NONE',  ( 111.7327233795247849, -1.325403438956436419, -9.854619843455211026 ) ) ;
#38785=CARTESIAN_POINT ( 'NONE',  ( 110.5520202545248054, -10.62599879583958717, -15.77991374673208469 ) ) ;
#38789=CARTESIAN_POINT ( 'NONE',  ( 79.33697550240769658, 5.018751399745532638, -6.205043556752605660 ) ) ;
#38791=CARTESIAN_POINT ( 'NONE',  ( 114.3719421295247827, 0.8980012041604618078, -13.39321520033831447 ) ) ;
#38792=CARTESIAN_POINT ( 'NONE',  ( 111.3854577545248645, -2.791137627527939813, -18.39754474579286025 ) ) ;
#38794=DIRECTION ( 'NONE',  ( 0.000000000000000000, 0.000000000000000000, 1.000000000000000000 ) ) ;
#38808=CARTESIAN_POINT ( 'NONE',  ( 113.4872481608379786, 0.3867979994853637526, -14.64321520033833401 ) ) ;
#38812=DIRECTION ( 'NONE',  ( 0.000000000000000000, 1.000000000000000000, 0.000000000000000000 ) ) ;
#38813=CARTESIAN_POINT ( 'NONE',  ( 112.3578015045248861, -6.936859964151250502, -18.39754474579286025 ) ) ;
#38815=VERTEX_POINT ( 'NONE', #41498 ) ;
#38818=CARTESIAN_POINT ( 'NONE',  ( 69.69189222814998175, -41.76310523276723785, -24.39321520033831447 ) ) ;
#38821=AXIS2_PLACEMENT_3D ( 'NONE', #23513, #9597, #5707 ) ;
#38822=CARTESIAN_POINT ( 'NONE',  ( 74.19189222814998175, -41.76310523276723785, -6.393215200338315363 ) ) ;
#38824=CARTESIAN_POINT ( 'NONE',  ( 113.2606921295247702, 0.8980012041604618078, -13.39321520033831447 ) ) ;
#38832=CARTESIAN_POINT ( 'NONE',  ( 115.2748327545248657, -2.477300249445798297, -19.15521520033831138 ) ) ;
#38834=CARTESIAN_POINT ( 'NONE',  ( 84.59925623653033711, -29.75466480065543706, -10.12692979306177143 ) ) ;
#38840=CARTESIAN_POINT ( 'NONE',  ( 113.3995983795247895, -0.7896495226426338832, -9.318865927141430916 ) ) ;
#38845=CARTESIAN_POINT ( 'NONE',  ( 111.5938171295247940, 0.1403307496149613920, -13.39321520033831447 ) ) ;
#38849=CARTESIAN_POINT ( 'NONE',  ( 109.2296393276947271, -6.249043720356506348, -18.46636368634833048 ) ) ;
#38854=CARTESIAN_POINT ( 'NONE',  ( 107.4266296295248821, -4.863998795839590272, -19.15521520033831493 ) ) ;
#38869=CYLINDRICAL_SURFACE ( 'NONE', #41315, 1.000000000000000888 ) ;
#38870=CARTESIAN_POINT ( 'NONE',  ( 110.2742077545248094, -7.250697342233347165, -7.631215200338321125 ) ) ;
#38872=CARTESIAN_POINT ( 'NONE',  ( 116.8928740015602870, 0.2848729546123598966, -14.64321520033831447 ) ) ;
#38873=CARTESIAN_POINT ( 'NONE',  ( 115.4137390045248566, -9.868328341294098749, -11.32035403202665869 ) ) ;
#38875=CARTESIAN_POINT ( 'NONE',  ( 117.1020249174801506, 1.596432964241469188, -5.416842142801578497 ) ) ;
#38879=CARTESIAN_POINT ( 'NONE',  ( 113.6079577545248043, -2.791137627527939813, -18.39754474579286025 ) ) ;
#38892=CARTESIAN_POINT ( 'NONE',  ( 114.2330358795247776, -8.402594152722688392, -9.854619843455216355 ) ) ;
#38895=CARTESIAN_POINT ( 'NONE',  ( 85.34837758929681684, -28.81250896213596135, -9.554009972945269880 ) ) ;
#38896=CARTESIAN_POINT ( 'NONE',  ( 112.9134265045247645, -7.250697342233347165, -19.15521520033831138 ) ) ;
#38899=CARTESIAN_POINT ( 'NONE',  ( 116.5944421295247793, -9.868328341294093420, -13.39321520033827007 ) ) ;
#38900=CARTESIAN_POINT ( 'NONE',  ( 109.2295733927577146, -1.759256525978093677, -8.933306666141186625 ) ) ;
#38902=CARTESIAN_POINT ( 'NONE',  ( 113.3995983795247895, -0.7896495226426338832, -9.318865927141430916 ) ) ;
#38903=LINE ( 'NONE', #25241, #40817 ) ;
#38906=CARTESIAN_POINT ( 'NONE',  ( 112.0799890045248475, 0.8980012041604421569, -15.77991374673208469 ) ) ;
#38910=AXIS2_PLACEMENT_3D ( 'NONE', #38818, #25383, #526 ) ;
#38919=CARTESIAN_POINT ( 'NONE',  ( 115.4831921295247952, 0.8980012041604618078, -13.39321520033831447 ) ) ;
#38927=CARTESIAN_POINT ( 'NONE',  ( 106.7320983795247855, -8.402594152722688392, -16.93181055722141792 ) ) ;
#38933=CARTESIAN_POINT ( 'NONE',  ( 64.40742206494232391, -35.25845966367313622, -5.871648730333305366 ) ) ;
#38934=( BOUNDED_SURFACE ( )  B_SPLINE_SURFACE ( 1, 2, ( 
 ( #13185, #20250, #16372, #30275, #44200, #40771, #16834, #6101, #30727, #2674, #44650, #16606, #41233, #23902, #37785, #6558, #20475, #30951, #34356, #17059, #44875, #13631, #27542, #14516, #31384, #605, #28428, #38226, #42341, #24560, #28210, #20917, #32056, #380, #17279, #42561, #31611, #3360, #11100, #31170, #25002, #7665, #14292, #34792, #14744, #20698, #45091, #823, #25233, #21581, #28655, #3575, #35238, #38896, #17487, #18160, #17937, #21354, #155, #6789, #11322, #42118, #34576, #13847, #14070, #38446, #24342, #10878, #10654, #7434, #24775, #38666, #27762, #10435, #27988, #3787, #7217, #4014, #35468, #41677, #31836, #4243, #7008, #21129, #41893, #35004, #17712, #29321, #15870, #12453, #15642, #1494, #36597, #43234, #29093, #12000, #22031, #39130, #21804, #32503, #19290, #1277, #18830, #11551, #14965, #7897, #15189, #42790, #39809, #39588, #15416, #4915, #25903, #18611, #35697, #5373, #32722, #43463, #8575, #32943, #43004, #18393, #1719, #8349, #43678, #1050, #28878, #4473, #32285, #29546, #11773, #22701, #22476, #36370, #22252, #25459, #39362, #12228, #33169, #25681, #36147, #5141, #19057, #26125, #1945, #35925, #8129, #40030, #4692, #8794, #29768, #34084, #33617, #26354, #12681, #34308, #40493, #19733, #9707, #44596, #13131 ),
 ( #22926, #40262, #6041, #33389, #3081, #23620, #37506, #23387, #30676, #19964, #17009, #36819, #9028, #33852, #2163, #30898, #6280, #20200, #2851, #16783, #16554, #20424, #13359, #27265, #12911, #44821, #41178, #2394, #9938, #23852, #37738, #6509, #2621, #5588, #19511, #37273, #16323, #16090, #29995, #26579, #30225, #30449, #44369, #27035, #23162, #43912, #9254, #37043, #40950, #5813, #44145, #26807, #40717, #9476, #21077, #20648, #34954, #3740, #6738, #24950, #7166, #11047, #7386, #24508, #38845, #21304, #38180, #35186, #3964, #45041, #17885, #31334, #17663, #27713, #7615, #31559, #24070, #4191, #38393, #10163, #31782, #37962, #555, #14465, #328, #41627, #21528, #3523, #18110, #34525, #14240, #31117, #6957, #10383, #13801, #24293, #28372, #10824, #20862, #42286, #35415, #32003, #34742, #13578, #41846, #3302, #17441, #14021, #108, #41407, #28157, #27489, #17227, #27936, #42067, #10606, #24722, #38610, #35866, #4639, #9141, #35647, #23046, #1226, #12570, #7849, #32675, #18561, #36933, #1443, #12794, #21754, #42737, #11721, #5704, #19621, #39537, #9365, #42513, #766, #25634, #4421, #23274, #43804, #26475, #33505, #29887, #36096, #40607, #2284, #16214, #32452, #5932, #30117, #21978, #44032, #40379, #26695, #37156, #8298, #19854 ) ),
 .UNSPECIFIED., .F., .F., .T. ) 
 B_SPLINE_SURFACE_WITH_KNOTS ( ( 2, 2 ),
 ( 3, 2, 2, 2, 2, 2, 2, 2, 2, 2, 2, 2, 2, 2, 2, 2, 2, 2, 2, 2, 2, 2, 2, 2, 2, 2, 2, 2, 2, 2, 2, 2, 2, 2, 2, 2, 2, 2, 2, 2, 2, 2, 2, 2, 2, 2, 2, 2, 2, 2, 2, 2, 2, 2, 2, 2, 2, 2, 2, 2, 2, 2, 2, 2, 2, 2, 2, 2, 2, 2, 2, 2, 2, 2, 2, 2, 2, 2, 2, 2, 3 ),
 ( 0.000000000000000000, 1.000000000000000000 ),
 ( 0.000000000000000000, 0.01250000000000000069, 0.02500000000000000139, 0.03749999999999999861, 0.05000000000000000278, 0.06250000000000000000, 0.07499999999999999722, 0.08749999999999999445, 0.1000000000000000056, 0.1125000000000000028, 0.1250000000000000000, 0.1375000000000000111, 0.1499999999999999944, 0.1625000000000000056, 0.1749999999999999889, 0.1875000000000000000, 0.2000000000000000111, 0.2124999999999999944, 0.2250000000000000056, 0.2374999999999999889, 0.2500000000000000000, 0.2625000000000000111, 0.2750000000000000222, 0.2874999999999999778, 0.2999999999999999889, 0.3125000000000000000, 0.3250000000000000111, 0.3375000000000000222, 0.3499999999999999778, 0.3624999999999999889, 0.3750000000000000000, 0.3875000000000000111, 0.4000000000000000222, 0.4124999999999999778, 0.4249999999999999889, 0.4375000000000000000, 0.4500000000000000111, 0.4625000000000000222, 0.4749999999999999778, 0.4874999999999999889, 0.5000000000000000000, 0.5124999999999999556, 0.5250000000000000222, 0.5374999999999999778, 0.5500000000000000444, 0.5625000000000000000, 0.5749999999999999556, 0.5875000000000000222, 0.5999999999999999778, 0.6125000000000000444, 0.6250000000000000000, 0.6374999999999999556, 0.6500000000000000222, 0.6624999999999999778, 0.6750000000000000444, 0.6875000000000000000, 0.6999999999999999556, 0.7125000000000000222, 0.7249999999999999778, 0.7375000000000000444, 0.7500000000000000000, 0.7624999999999999556, 0.7750000000000000222, 0.7874999999999999778, 0.8000000000000000444, 0.8125000000000000000, 0.8249999999999999556, 0.8375000000000000222, 0.8499999999999999778, 0.8625000000000000444, 0.8750000000000000000, 0.8874999999999999556, 0.9000000000000000222, 0.9124999999999999778, 0.9250000000000000444, 0.9375000000000000000, 0.9499999999999999556, 0.9625000000000000222, 0.9749999999999999778, 0.9875000000000000444, 1.000000000000000000 ),
 .UNSPECIFIED. ) 
 GEOMETRIC_REPRESENTATION_ITEM ( )  RATIONAL_B_SPLINE_SURFACE ( (
 ( 1.000000000000000000, 0.9238795325112869605, 1.000000000000000000, 0.9238795325112869605, 1.000000000000000000, 0.9238795325112869605, 1.000000000000000000, 0.9238795325112869605, 1.000000000000000000, 0.9238795325112869605, 1.000000000000000000, 0.9238795325112869605, 1.000000000000000000, 0.9238795325112869605, 1.000000000000000000, 0.9238795325112869605, 1.000000000000000000, 0.9238795325112869605, 1.000000000000000000, 0.9238795325112869605, 1.000000000000000000, 0.9238795325112869605, 1.000000000000000000, 0.9238795325112869605, 1.000000000000000000, 0.9238795325112869605, 1.000000000000000000, 0.9238795325112869605, 1.000000000000000000, 0.9238795325112869605, 1.000000000000000000, 0.9238795325112869605, 1.000000000000000000, 0.9238795325112869605, 1.000000000000000000, 0.9238795325112869605, 1.000000000000000000, 0.9238795325112869605, 1.000000000000000000, 0.9238795325112869605, 1.000000000000000000, 0.9238795325112869605, 1.000000000000000000, 0.9238795325112869605, 1.000000000000000000, 0.9238795325112869605, 1.000000000000000000, 0.9238795325112869605, 1.000000000000000000, 0.9238795325112869605, 1.000000000000000000, 0.9238795325112869605, 1.000000000000000000, 0.9238795325112869605, 1.000000000000000000, 0.9238795325112869605, 1.000000000000000000, 0.9238795325112869605, 1.000000000000000000, 0.9238795325112869605, 1.000000000000000000, 0.9238795325112869605, 1.000000000000000000, 0.9238795325112869605, 1.000000000000000000, 0.9238795325112869605, 1.000000000000000000, 0.9238795325112869605, 1.000000000000000000, 0.9238795325112869605, 1.000000000000000000, 0.9238795325112869605, 1.000000000000000000, 0.9238795325112869605, 1.000000000000000000, 0.9238795325112869605, 1.000000000000000000, 0.9238795325112869605, 1.000000000000000000, 0.9238795325112869605, 1.000000000000000000, 0.9238795325112869605, 1.000000000000000000, 0.9238795325112869605, 1.000000000000000000, 0.9238795325112869605, 1.000000000000000000, 0.9238795325112869605, 1.000000000000000000, 0.9238795325112869605, 1.000000000000000000, 0.9238795325112869605, 1.000000000000000000, 0.9238795325112869605, 1.000000000000000000, 0.9238795325112869605, 1.000000000000000000, 0.9238795325112869605, 1.000000000000000000, 0.9238795325112869605, 1.000000000000000000, 0.9238795325112869605, 1.000000000000000000, 0.9238795325112869605, 1.000000000000000000, 0.9238795325112869605, 1.000000000000000000, 0.9238795325112869605, 1.000000000000000000, 0.9238795325112869605, 1.000000000000000000, 0.9238795325112869605, 1.000000000000000000, 0.9238795325112869605, 1.000000000000000000, 0.9238795325112869605, 1.000000000000000000, 0.9238795325112869605, 1.000000000000000000, 0.9238795325112869605, 1.000000000000000000, 0.9238795325112869605, 1.000000000000000000, 0.9238795325112869605, 1.000000000000000000, 0.9238795325112869605, 1.000000000000000000, 0.9238795325112869605, 1.000000000000000000, 0.9238795325112869605, 1.000000000000000000, 0.9238795325112869605, 1.000000000000000000, 0.9238795325112869605, 1.000000000000000000, 0.9238795325112869605, 1.000000000000000000, 0.9238795325112869605, 1.000000000000000000, 0.9238795325112869605, 1.000000000000000000, 0.9238795325112869605, 1.000000000000000000, 0.9238795325112869605, 1.000000000000000000, 0.9238795325112869605, 1.000000000000000000, 0.9238795325112869605, 1.000000000000000000, 0.9238795325112869605, 1.000000000000000000, 0.9238795325112869605, 1.000000000000000000, 0.9238795325112869605, 1.000000000000000000, 0.9238795325112869605, 1.000000000000000000, 0.9238795325112869605, 1.000000000000000000, 0.9238795325112869605, 1.000000000000000000),
 ( 1.000000000000000000, 0.9238795325112869605, 1.000000000000000000, 0.9238795325112869605, 1.000000000000000000, 0.9238795325112869605, 1.000000000000000000, 0.9238795325112869605, 1.000000000000000000, 0.9238795325112869605, 1.000000000000000000, 0.9238795325112869605, 1.000000000000000000, 0.9238795325112869605, 1.000000000000000000, 0.9238795325112869605, 1.000000000000000000, 0.9238795325112869605, 1.000000000000000000, 0.9238795325112869605, 1.000000000000000000, 0.9238795325112869605, 1.000000000000000000, 0.9238795325112869605, 1.000000000000000000, 0.9238795325112869605, 1.000000000000000000, 0.9238795325112869605, 1.000000000000000000, 0.9238795325112869605, 1.000000000000000000, 0.9238795325112869605, 1.000000000000000000, 0.9238795325112869605, 1.000000000000000000, 0.9238795325112869605, 1.000000000000000000, 0.9238795325112869605, 1.000000000000000000, 0.9238795325112869605, 1.000000000000000000, 0.9238795325112869605, 1.000000000000000000, 0.9238795325112869605, 1.000000000000000000, 0.9238795325112869605, 1.000000000000000000, 0.9238795325112869605, 1.000000000000000000, 0.9238795325112869605, 1.000000000000000000, 0.9238795325112869605, 1.000000000000000000, 0.9238795325112869605, 1.000000000000000000, 0.9238795325112869605, 1.000000000000000000, 0.9238795325112869605, 1.000000000000000000, 0.9238795325112869605, 1.000000000000000000, 0.9238795325112869605, 1.000000000000000000, 0.9238795325112869605, 1.000000000000000000, 0.9238795325112869605, 1.000000000000000000, 0.9238795325112869605, 1.000000000000000000, 0.9238795325112869605, 1.000000000000000000, 0.9238795325112869605, 1.000000000000000000, 0.9238795325112869605, 1.000000000000000000, 0.9238795325112869605, 1.000000000000000000, 0.9238795325112869605, 1.000000000000000000, 0.9238795325112869605, 1.000000000000000000, 0.9238795325112869605, 1.000000000000000000, 0.9238795325112869605, 1.000000000000000000, 0.9238795325112869605, 1.000000000000000000, 0.9238795325112869605, 1.000000000000000000, 0.9238795325112869605, 1.000000000000000000, 0.9238795325112869605, 1.000000000000000000, 0.9238795325112869605, 1.000000000000000000, 0.9238795325112869605, 1.000000000000000000, 0.9238795325112869605, 1.000000000000000000, 0.9238795325112869605, 1.000000000000000000, 0.9238795325112869605, 1.000000000000000000, 0.9238795325112869605, 1.000000000000000000, 0.9238795325112869605, 1.000000000000000000, 0.9238795325112869605, 1.000000000000000000, 0.9238795325112869605, 1.000000000000000000, 0.9238795325112869605, 1.000000000000000000, 0.9238795325112869605, 1.000000000000000000, 0.9238795325112869605, 1.000000000000000000, 0.9238795325112869605, 1.000000000000000000, 0.9238795325112869605, 1.000000000000000000, 0.9238795325112869605, 1.000000000000000000, 0.9238795325112869605, 1.000000000000000000, 0.9238795325112869605, 1.000000000000000000, 0.9238795325112869605, 1.000000000000000000, 0.9238795325112869605, 1.000000000000000000, 0.9238795325112869605, 1.000000000000000000, 0.9238795325112869605, 1.000000000000000000, 0.9238795325112869605, 1.000000000000000000, 0.9238795325112869605, 1.000000000000000000, 0.9238795325112869605, 1.000000000000000000, 0.9238795325112869605, 1.000000000000000000, 0.9238795325112869605, 1.000000000000000000, 0.9238795325112869605, 1.000000000000000000, 0.9238795325112869605, 1.000000000000000000, 0.9238795325112869605, 1.000000000000000000, 0.9238795325112869605, 1.000000000000000000, 0.9238795325112869605, 1.000000000000000000, 0.9238795325112869605, 1.000000000000000000, 0.9238795325112869605, 1.000000000000000000, 0.9238795325112869605, 1.000000000000000000) ) ) 
 REPRESENTATION_ITEM ( '' )  SURFACE ( )  );
#38946=FACE_OUTER_BOUND ( 'NONE', #43361, .T. ) ;
#38947=AXIS2_PLACEMENT_3D ( 'NONE', #16764, #19948, #10369 ) ;
#38951=CARTESIAN_POINT ( 'NONE',  ( 112.5661608795247872, -1.325403438956436419, -16.93181055722141792 ) ) ;
#38954=CARTESIAN_POINT ( 'NONE',  ( 113.4437166496844895, 0.5600166689815611054, -12.14321520033829849 ) ) ;
#38962=CARTESIAN_POINT ( 'NONE',  ( 112.4967077545247633, -2.791137627527939813, -18.39754474579286025 ) ) ;
#38964=EDGE_LOOP ( 'NONE', ( #15289, #8741 ) ) ;
#38973=CARTESIAN_POINT ( 'NONE',  ( 63.69189222814998175, -64.02637234200076932, -46.77412892735921446 ) ) ;
#38977=EDGE_CURVE ( 'NONE', #22388, #44662, #1185, .T. ) ;
#38979=CARTESIAN_POINT ( 'NONE',  ( 115.8304577545247582, -2.791137627527939813, -18.39754474579286025 ) ) ;
#38982=ORIENTED_EDGE ( 'NONE', *, *, #29029, .T. ) ;
#38985=VECTOR ( 'NONE', #22614, 1000.000000000000114 ) ;
#38999=CARTESIAN_POINT ( 'NONE',  ( 64.69189222814998175, -41.76310523276723785, -6.393215200338315363 ) ) ;
#39003=CARTESIAN_POINT ( 'NONE',  ( 116.7565503026016813, -4.863998795840742240, -18.55532337341522364 ) ) ;
#39010=CARTESIAN_POINT ( 'NONE',  ( 115.5526452545247622, 0.8980012041604421569, -11.00651665394454071 ) ) ;
#39011=CIRCLE ( 'NONE', #7696, 0.5000000000000004441 ) ;
#39012=CARTESIAN_POINT ( 'NONE',  ( 114.4413952545248350, -9.868328341294098749, -15.46607636864997204 ) ) ;
#39013=CARTESIAN_POINT ( 'NONE',  ( 112.0105358795248804, -8.402594152722688392, -9.854619843455216355 ) ) ;
#39016=EDGE_LOOP ( 'NONE', ( #17905, #27079, #4947, #42085 ) ) ;
#39018=CARTESIAN_POINT ( 'NONE',  ( 109.1629577545248395, -7.250697342233347165, -7.631215200338321125 ) ) ;
#39019=FACE_BOUND ( 'NONE', #9841, .T. ) ;
#39024=CARTESIAN_POINT ( 'NONE',  ( 113.0523327545247838, -2.477300249445798297, -19.15521520033831138 ) ) ;
#39025=CARTESIAN_POINT ( 'NONE',  ( 109.8574890045248509, -9.868328341294098749, -11.32035403202665869 ) ) ;
#39030=VECTOR ( 'NONE', #35309, 1000.000000000000000 ) ;
#39038=CARTESIAN_POINT ( 'NONE',  ( 113.2226630180080775, 0.7607806665038616689, -14.64321520033831447 ) ) ;
#39041=CARTESIAN_POINT ( 'NONE',  ( 110.7164878519203768, 0.2518737723193609224, -12.14321520033831625 ) ) ;
#39044=CARTESIAN_POINT ( 'NONE',  ( 115.0664733795247798, -8.938348069036489818, -17.46756447353520159 ) ) ;
#39047=ORIENTED_EDGE ( 'NONE', *, *, #32802, .F. ) ;
#39052=AXIS2_PLACEMENT_3D ( 'NONE', #41823, #21733, #25386 ) ;
#39057=CARTESIAN_POINT ( 'NONE',  ( 111.8716296295247901, -4.863998795839590272, -19.15521520033831493 ) ) ;
#39064=VERTEX_POINT ( 'NONE', #43503 ) ;
#39067=CARTESIAN_POINT ( 'NONE',  ( 84.43379914120473018, -30.20550309442903725, -11.21534971632906519 ) ) ;
#39068=CARTESIAN_POINT ( 'NONE',  ( 116.3166296295247832, -4.863998795839590272, -19.15521520033831493 ) ) ;
#39071=ORIENTED_EDGE ( 'NONE', *, *, #34210, .F. ) ;
#39073=CARTESIAN_POINT ( 'NONE',  ( 109.5577383310706807, 0.1843591316377651834, -12.14321520033833757 ) ) ;
#39074=CARTESIAN_POINT ( 'NONE',  ( 113.8857702545248003, -10.62599879583958717, -15.77991374673208469 ) ) ;
#39078=CARTESIAN_POINT ( 'NONE',  ( 112.0799890045248759, -9.868328341294150263, -11.32035403202671020 ) ) ;
#39081=ORIENTED_EDGE ( 'NONE', *, *, #9432, .F. ) ;
#39083=CARTESIAN_POINT ( 'NONE',  ( 109.2294364582409116, -3.949221096940591202, -18.45898293540659907 ) ) ;
#39086=CARTESIAN_POINT ( 'NONE',  ( 115.3442858795247759, -8.402594152722688392, -9.854619843455216355 ) ) ;
#39087=CARTESIAN_POINT ( 'NONE',  ( 106.7320983795247855, -0.7896495226426338832, -9.318865927141430916 ) ) ;
#39090=DIRECTION ( 'NONE',  ( 0.000000000000000000, 0.000000000000000000, 1.000000000000000000 ) ) ;
#39103=CARTESIAN_POINT ( 'NONE',  ( 108.5378796295247810, -4.863998795839590272, -19.15521520033831493 ) ) ;
#39104=CARTESIAN_POINT ( 'NONE',  ( 70.36267391504958368, -5.685877709920885259, -4.893215200338314474 ) ) ;
#39107=CARTESIAN_POINT ( 'NONE',  ( 111.8716296295247901, -4.863998795839590272, -8.388885654883775800 ) ) ;
#39110=CARTESIAN_POINT ( 'NONE',  ( 117.2294421295247844, 1.035107641088057973, -5.059859068394715109 ) ) ;
#39114=CARTESIAN_POINT ( 'NONE',  ( 112.2188952545247531, -9.868328341294098749, -15.46607636864997204 ) ) ;
#39115=MECHANICAL_DESIGN_GEOMETRIC_PRESENTATION_REPRESENTATION('',(#18717),#23123);
#39126=CARTESIAN_POINT ( 'NONE',  ( 114.6497546295247929, -4.863998795839590272, -18.39754474579285315 ) ) ;
#39129=CARTESIAN_POINT ( 'NONE',  ( 86.22611448523406352, -26.68659777590136528, -8.453450719925958978 ) ) ;
#39130=CARTESIAN_POINT ( 'NONE',  ( 109.8574890045247940, 0.8980012041604421569, -15.77991374673208469 ) ) ;
#39134=CARTESIAN_POINT ( 'NONE',  ( 109.2294421266624767, -3.229083252145867444, -8.131417123785080747 ) ) ;
#39137=VECTOR ( 'NONE', #24496, 1000.000000000000000 ) ;
#39138=CARTESIAN_POINT ( 'NONE',  ( 113.3301452545248083, 0.8980012041604421569, -11.00651665394454071 ) ) ;
#39139=CARTESIAN_POINT ( 'NONE',  ( 69.69189222814998175, -41.76310523276723785, -24.39321520033831447 ) ) ;
#39140=CARTESIAN_POINT ( 'NONE',  ( 83.36558916507954109, -33.11616680504563703, -22.91154035974133407 ) ) ;
#39143=CARTESIAN_POINT ( 'NONE',  ( 109.7185827545247889, -2.477300249445798297, -19.15521520033831138 ) ) ;
#39152=VECTOR ( 'NONE', #4458, 1000.000000000000000 ) ;
#39153=CARTESIAN_POINT ( 'NONE',  ( 115.6220983795247861, -0.7896495226426338832, -9.318865927141430916 ) ) ;
#39156=CARTESIAN_POINT ( 'NONE',  ( 86.84453910206313765, -17.83168818462593919, -19.39321520033831447 ) ) ;
#39157=ORIENTED_EDGE ( 'NONE', *, *, #43495, .T. ) ;
#39163=VECTOR ( 'NONE', #24995, 1000.000000000000000 ) ;
#39166=CARTESIAN_POINT ( 'NONE',  ( 76.69189222814998175, -55.76602098829192755, -2.607500914624014232 ) ) ;
#39169=DIRECTION ( 'NONE',  ( -1.000000000000000000, 0.000000000000000000, 0.000000000000000000 ) ) ;
#39178=ORIENTED_EDGE ( 'NONE', *, *, #11621, .T. ) ;
#39180=CARTESIAN_POINT ( 'NONE',  ( 112.2188952545247531, -9.868328341294098749, -15.46607636864997204 ) ) ;
#39182=CARTESIAN_POINT ( 'NONE',  ( 114.3719421295247827, -9.868328341294093420, -13.39321520033836244 ) ) ;
#39190=CARTESIAN_POINT ( 'NONE',  ( 76.19189222814999596, -49.76310523276725206, -29.87698278062875445 ) ) ;
#39191=CARTESIAN_POINT ( 'NONE',  ( 107.3571765045248299, -2.791137627527939813, -8.388885654883777576 ) ) ;
#39202=DIRECTION ( 'NONE',  ( -1.000000000000000000, 0.000000000000000000, 0.000000000000000000 ) ) ;
#39205=ORIENTED_EDGE ( 'NONE', *, *, #26305, .F. ) ;
#39220=LINE ( 'NONE', #38531, #25833 ) ;
#39228=CARTESIAN_POINT ( 'NONE',  ( 116.6874845501451574, -8.042305857947342318, -17.38640671321973841 ) ) ;
#39235=EDGE_CURVE ( 'NONE', #10734, #35580, #22898, .T. ) ;
#39236=CARTESIAN_POINT ( 'NONE',  ( 115.6915515045247531, -2.477300249445798297, -7.631215200338321125 ) ) ;
#39237=CARTESIAN_POINT ( 'NONE',  ( 112.7745202545247878, 0.1403307496149616695, -11.32035403202665336 ) ) ;
#39238=CARTESIAN_POINT ( 'NONE',  ( 114.9275671295247889, 0.1403307496149613920, -13.39321520033831447 ) ) ;
#39246=CARTESIAN_POINT ( 'NONE',  ( 109.2295375745178490, -0.2444348417507766491, -15.53743370689154091 ) ) ;
#39247=CARTESIAN_POINT ( 'NONE',  ( 87.44708369096657918, -29.99489077589588959, -12.39321520033834645 ) ) ;
#39250=CARTESIAN_POINT ( 'NONE',  ( 114.3024890045248156, 0.8980012041604421569, -15.77991374673208469 ) ) ;
#39251=CARTESIAN_POINT ( 'NONE',  ( 109.4407702545248355, 0.1403307496149616695, -11.32035403202665336 ) ) ;
#39256=CARTESIAN_POINT ( 'NONE',  ( 70.19189222814998175, -41.58126682492877535, -29.83537093841426469 ) ) ;
#39257=EDGE_CURVE ( 'NONE', #38752, #38575, #23035, .T. ) ;
#39262=ORIENTED_EDGE ( 'NONE', *, *, #9786, .F. ) ;
#39273=CARTESIAN_POINT ( 'NONE',  ( 106.1070202545248407, 0.1403307496149616695, -11.32035403202665336 ) ) ;
#39276=ORIENTED_EDGE ( 'NONE', *, *, #15956, .F. ) ;
#39283=CARTESIAN_POINT ( 'NONE',  ( 65.19189222814998175, -41.76310523276723785, -20.39321520033831447 ) ) ;
#39284=CARTESIAN_POINT ( 'NONE',  ( 113.3301452545248083, 0.8980012041604421569, -11.00651665394454071 ) ) ;
#39285=CARTESIAN_POINT ( 'NONE',  ( 117.1280733121688371, -11.26650585198349752, -21.76132083932495220 ) ) ;
#39292=CARTESIAN_POINT ( 'NONE',  ( 116.5944421295247793, 0.8980012041604618078, -13.39321520033831447 ) ) ;
#39294=CARTESIAN_POINT ( 'NONE',  ( 114.9970202545248412, -10.62599879583958717, -15.77991374673208469 ) ) ;
#39299=CARTESIAN_POINT ( 'NONE',  ( 62.66011239371932362, -37.43768621791543438, -5.179380419204645314 ) ) ;
#39300=CARTESIAN_POINT ( 'NONE',  ( 111.3160046295247838, -4.863998795839590272, -7.631215200338315796 ) ) ;
#39302=B_SPLINE_CURVE_WITH_KNOTS ( 'NONE', 3,
 ( #28468, #42375, #11136, #25039, #21616, #4277 ),
 .UNSPECIFIED., .F., .F.,
 ( 4, 2, 4 ),
 ( 0.000000000000000000, 0.5000000000000000000, 1.000000000000000000 ),
 .UNSPECIFIED. ) ;
#39310=CARTESIAN_POINT ( 'NONE',  ( 109.2294423771211314, -10.02588119094734154, -11.04280315885711516 ) ) ;
#39314=CARTESIAN_POINT ( 'NONE',  ( 116.0388171295248014, 0.1403307496149613920, -13.39321520033831447 ) ) ;
#39318=DIRECTION ( 'NONE',  ( 0.000000000000000000, 0.000000000000000000, 1.000000000000000000 ) ) ;
#39333=CARTESIAN_POINT ( 'NONE',  ( 109.3018640045248304, -10.62599879583958717, -11.00651665394454604 ) ) ;
#39336=CARTESIAN_POINT ( 'NONE',  ( 115.2053796295247849, -4.863998795839590272, -8.388885654883775800 ) ) ;
#39345=CARTESIAN_POINT ( 'NONE',  ( 110.5520202545248054, 0.1403307496149616695, -11.32035403202665336 ) ) ;
#39356=CARTESIAN_POINT ( 'NONE',  ( 114.1635827545248389, -6.936859964151250502, -8.388885654883777576 ) ) ;
#39361=CARTESIAN_POINT ( 'NONE',  ( 85.26085842212216903, -29.02448141952688232, -9.765951594476932840 ) ) ;
#39362=CARTESIAN_POINT ( 'NONE',  ( 107.1488171295247867, -10.62599879583958540, -13.39321520033831447 ) ) ;
#39365=CARTESIAN_POINT ( 'NONE',  ( 115.8523959279789892, 0.1843591316377651834, -14.64321520033831447 ) ) ;
#39367=DIRECTION ( 'NONE',  ( 0.000000000000000000, 0.000000000000000000, -1.000000000000000000 ) ) ;
#39369=CARTESIAN_POINT ( 'NONE',  ( 115.3442858795247759, -0.7896495226426338832, -17.46756447353520159 ) ) ;
#39370=CARTESIAN_POINT ( 'NONE',  ( 117.0302221353151424, 1.731593677198245418, -21.24358807290060369 ) ) ;
#39371=CARTESIAN_POINT ( 'NONE',  ( 116.5944421295247793, 0.8980012041604618078, -13.39321520033831447 ) ) ;
#39374=CARTESIAN_POINT ( 'NONE',  ( 112.9134265045247645, -7.250697342233347165, -19.15521520033831138 ) ) ;
#39377=CARTESIAN_POINT ( 'NONE',  ( 112.5186459279789801, 0.1843591316377651834, -14.64321520033832691 ) ) ;
#39385=CARTESIAN_POINT ( 'NONE',  ( 111.8716296295247901, -4.863998795839590272, -19.15521520033831493 ) ) ;
#39393=CARTESIAN_POINT ( 'NONE',  ( 60.19189222814998175, -75.31442247550837976, -37.94335727672635272 ) ) ;
#39399=CARTESIAN_POINT ( 'NONE',  ( 64.43740640915127926, -35.20632691772231482, -5.871463680831255694 ) ) ;
#39404=CARTESIAN_POINT ( 'NONE',  ( 117.2294421295247844, 0.6306099254434621715, -14.64321520033831447 ) ) ;
#39410=CARTESIAN_POINT ( 'NONE',  ( 63.69189222814998175, -40.21211973637273474, -6.893215200338315363 ) ) ;
#39412=ORIENTED_EDGE ( 'NONE', *, *, #4384, .T. ) ;
#39414=CARTESIAN_POINT ( 'NONE',  ( 114.7886608795247696, -1.325403438956436419, -16.93181055722141792 ) ) ;
#39415=LINE ( 'NONE', #18883, #11737 ) ;
#39424=CARTESIAN_POINT ( 'NONE',  ( 108.3295202545248657, 0.1403307496149616695, -11.32035403202665336 ) ) ;
#39432=B_SPLINE_CURVE_WITH_KNOTS ( 'NONE', 3,
 ( #42097, #17261, #31815, #11081, #10861, #24983, #14054, #805, #24756, #35222 ),
 .UNSPECIFIED., .F., .F.,
 ( 4, 3, 3, 4 ),
 ( 0.000000000000000000, 0.0002476486447139030302, 0.0004952972925464440039, 0.0009604418836934600166 ),
 .UNSPECIFIED. ) ;
#39436=CARTESIAN_POINT ( 'NONE',  ( 63.06909581425561129, -64.46843347564573889, -46.33544452488994381 ) ) ;
#39439=CARTESIAN_POINT ( 'NONE',  ( 116.3860827545247787, -6.936859964151250502, -8.388885654883777576 ) ) ;
#39460=CARTESIAN_POINT ( 'NONE',  ( 116.6728924761787880, -8.584822191178330897, -16.85008389185930966 ) ) ;
#39464=EDGE_LOOP ( 'NONE', ( #20942, #40182, #30367, #31086, #8430, #37860 ) ) ;
#39467=CARTESIAN_POINT ( 'NONE',  ( 110.3436608795247764, -1.325403438956436419, -16.93181055722141792 ) ) ;
#39468=CARTESIAN_POINT ( 'NONE',  ( 114.5803015045248117, -6.936859964151250502, -18.39754474579286025 ) ) ;
#39471=ORIENTED_EDGE ( 'NONE', *, *, #17680, .T. ) ;
#39473=CARTESIAN_POINT ( 'NONE',  ( 108.6073327545248048, -2.477300249445798297, -19.15521520033831138 ) ) ;
#39476=CARTESIAN_POINT ( 'NONE',  ( 109.2295988934735504, -0.1244266206082473986, -15.29196534783836370 ) ) ;
#39479=CARTESIAN_POINT ( 'NONE',  ( 110.5520202545248054, -10.62599879583958717, -15.77991374673208469 ) ) ;
#39480=CARTESIAN_POINT ( 'NONE',  ( 112.1494421295248003, -9.868328341294093420, -13.39321520033831447 ) ) ;
#39497=CARTESIAN_POINT ( 'NONE',  ( 110.5740408578216858, 0.04929351793716424401, -12.14321520033834467 ) ) ;
#39500=CARTESIAN_POINT ( 'NONE',  ( 116.5944421295247793, 0.8980012041604618078, -13.39321520033831447 ) ) ;
#39502=ORIENTED_EDGE ( 'NONE', *, *, #2511, .T. ) ;
#39512=CARTESIAN_POINT ( 'NONE',  ( 112.7745202545247878, -10.62599879583958717, -15.77991374673208469 ) ) ;
#39522=CIRCLE ( 'NONE', #16229, 2.000000000000000000 ) ;
#39526=CARTESIAN_POINT ( 'NONE',  ( 117.2294421295247844, 0.6306099254434621715, -12.14321520033831625 ) ) ;
#39528=B_SPLINE_CURVE_WITH_KNOTS ( 'NONE', 3,
 ( #3337, #44626, #27063, #3111, #13607, #41208, #2884, #23650, #38206, #20676 ),
 .UNSPECIFIED., .F., .F.,
 ( 4, 3, 3, 4 ),
 ( 0.000000000000000000, 0.0002476486447138765215, 0.0004952972925464020452, 0.0009604418836934619681 ),
 .UNSPECIFIED. ) ;
#39531=CARTESIAN_POINT ( 'NONE',  ( 62.54698291256610787, -37.31319233293334037, -5.252116654659598538 ) ) ;
#39532=CARTESIAN_POINT ( 'NONE',  ( 108.6767858795247861, -0.7896495226426338832, -17.46756447353520159 ) ) ;
#39535=FACE_OUTER_BOUND ( 'NONE', #26059, .T. ) ;
#39536=CARTESIAN_POINT ( 'NONE',  ( 116.2659068881580708, -12.01880880694303855, -6.893215200338315363 ) ) ;
#39537=CARTESIAN_POINT ( 'NONE',  ( 106.5931921295248372, -9.868328341294093420, -13.39321520033831447 ) ) ;
#39538=ORIENTED_EDGE ( 'NONE', *, *, #18790, .T. ) ;
#39540=CARTESIAN_POINT ( 'NONE',  ( 116.4555358795247884, -0.7896495226426338832, -17.46756447353520159 ) ) ;
#39541=CARTESIAN_POINT ( 'NONE',  ( 109.2294421560451809, -10.06481071435802832, -15.15239973608284885 ) ) ;
#39543=CARTESIAN_POINT ( 'NONE',  ( 111.3160046295247838, -4.863998795839590272, -18.39754474579285315 ) ) ;
#39544=CARTESIAN_POINT ( 'NONE',  ( 115.4831921295247952, -9.868328341294093420, -13.39321520033831447 ) ) ;
#39546=CARTESIAN_POINT ( 'NONE',  ( 82.42994493343583429, -31.76310523276723430, -22.89321520033831803 ) ) ;
#39550=EDGE_CURVE ( 'NONE', #32144, #40625, #42548, .T. ) ;
#39562=FACE_OUTER_BOUND ( 'NONE', #4983, .T. ) ;
#39563=CARTESIAN_POINT ( 'NONE',  ( 112.7745202545247878, 0.1403307496149616695, -11.32035403202665336 ) ) ;
#39564=AXIS2_PLACEMENT_3D ( 'NONE', #26881, #33703, #15948 ) ;
#39568=DIRECTION ( 'NONE',  ( 0.000000000000000000, -1.000000000000000000, 0.000000000000000000 ) ) ;
#39571=CARTESIAN_POINT ( 'NONE',  ( 109.0935046295247872, -4.863998795839590272, -18.39754474579285315 ) ) ;
#39573=DIRECTION ( 'NONE',  ( 0.000000000000000000, 0.000000000000000000, -1.000000000000000000 ) ) ;
#39580=ADVANCED_FACE ( 'NONE', ( #35455, #7204 ), #21117, .F. ) ;
#39582=CARTESIAN_POINT ( 'NONE',  ( 109.2324108795247923, -1.325403438956436419, -16.93181055722141792 ) ) ;
#39588=CARTESIAN_POINT ( 'NONE',  ( 109.0240515045248202, -2.477300249445798297, -7.631215200338321125 ) ) ;
#39591=DIRECTION ( 'NONE',  ( 0.000000000000000000, 1.000000000000000000, -1.195183497228115774E-16 ) ) ;
#39594=CARTESIAN_POINT ( 'NONE',  ( 106.3153796295248412, -4.863998795839590272, -8.388885654883775800 ) ) ;
#39596=CARTESIAN_POINT ( 'NONE',  ( 82.53488078675573547, -31.62014037238083830, -22.36964567811433469 ) ) ;
#39599=CARTESIAN_POINT ( 'NONE',  ( 106.1070202545248407, -10.62599879583958717, -15.77991374673208469 ) ) ;
#39602=EDGE_LOOP ( 'NONE', ( #25027, #15026, #26074, #10238, #1082, #16847 ) ) ;
#39603=CARTESIAN_POINT ( 'NONE',  ( 70.19189222814998175, -66.16203077818754252, -36.43649583506466882 ) ) ;
#39610=CARTESIAN_POINT ( 'NONE',  ( 112.2883483795247770, -0.7896495226426338832, -9.318865927141430916 ) ) ;
#39612=CARTESIAN_POINT ( 'NONE',  ( 83.14922721495791791, -33.70571089342944049, -22.39321520033831092 ) ) ;
#39630=EDGE_CURVE ( 'NONE', #31933, #20305, #14730, .T. ) ;
#39636=DIRECTION ( 'NONE',  ( 0.000000000000000000, 0.000000000000000000, -1.000000000000000000 ) ) ;
#39640=CARTESIAN_POINT ( 'NONE',  ( 113.8163171295247764, -10.62599879583958540, -13.39321520033831447 ) ) ;
#39641=CARTESIAN_POINT ( 'NONE',  ( 113.7468640045248236, 0.1403307496149616695, -15.46607636864997204 ) ) ;
#39652=CARTESIAN_POINT ( 'NONE',  ( 106.1070202545248407, 0.1403307496149616695, -11.32035403202665336 ) ) ;
#39657=DIRECTION ( 'NONE',  ( 0.000000000000000000, -0.5905882410490338463, -0.8069730661766898461 ) ) ;
#39663=CARTESIAN_POINT ( 'NONE',  ( 114.4413952545248350, -9.868328341294098749, -15.46607636864997204 ) ) ;
#39667=ORIENTED_EDGE ( 'NONE', *, *, #21711, .F. ) ;
#39674=CARTESIAN_POINT ( 'NONE',  ( 92.26512299712632625, -23.76310523276723785, -20.89321520033831447 ) ) ;
#39680=CARTESIAN_POINT ( 'NONE',  ( 70.19189222814998175, -49.76310523276723785, -36.33917278160906505 ) ) ;
#39691=CARTESIAN_POINT ( 'NONE',  ( 114.5803015045248117, -2.477300249445798297, -7.631215200338321125 ) ) ;
#39692=CARTESIAN_POINT ( 'NONE',  ( 108.6073327545248048, -6.936859964151250502, -8.388885654883777576 ) ) ;
#39693=CARTESIAN_POINT ( 'NONE',  ( 108.3295202545248657, 0.1403307496149616695, -11.32035403202665336 ) ) ;
#39698=CARTESIAN_POINT ( 'NONE',  ( 109.3018640045248304, -10.62599879583958717, -11.00651665394454604 ) ) ;
#39699=DIRECTION ( 'NONE',  ( 0.000000000000000000, 0.000000000000000000, -1.000000000000000000 ) ) ;
#39704=CARTESIAN_POINT ( 'NONE',  ( 110.9687390045248350, 0.8980012041604421569, -15.77991374673208469 ) ) ;
#39705=CARTESIAN_POINT ( 'NONE',  ( 110.8298327545248299, -6.936859964151250502, -8.388885654883777576 ) ) ;
#39708=CARTESIAN_POINT ( 'NONE',  ( 65.82164714941100669, 4.169909004287361221, -19.39321520033831447 ) ) ;
#39722=CARTESIAN_POINT ( 'NONE',  ( 107.0099108795247815, -1.325403438956436419, -16.93181055722141792 ) ) ;
#39725=EDGE_LOOP ( 'NONE', ( #28536, #20388, #43844, #3708 ) ) ;
#39728=ORIENTED_EDGE ( 'NONE', *, *, #24371, .T. ) ;
#39730=CARTESIAN_POINT ( 'NONE',  ( 62.15098047326635111, -65.30822568471278089, -44.85084686348432825 ) ) ;
#39731=CARTESIAN_POINT ( 'NONE',  ( 109.7880358795247986, -0.7896495226426338832, -17.46756447353520159 ) ) ;
#39736=CARTESIAN_POINT ( 'NONE',  ( 66.06194382436763135, -14.97931106434683635, -4.893215200338314474 ) ) ;
#39741=CARTESIAN_POINT ( 'NONE',  ( 112.4272546295247821, -4.863998795839590272, -7.631215200338315796 ) ) ;
#39742=CARTESIAN_POINT ( 'NONE',  ( 116.0388171295248014, 0.1403307496149613920, -13.39321520033831447 ) ) ;
#39743=CARTESIAN_POINT ( 'NONE',  ( 112.3578015045248861, -2.477300249445798297, -7.631215200338321125 ) ) ;
#39746=ORIENTED_EDGE ( 'NONE', *, *, #23651, .F. ) ;
#39748=CARTESIAN_POINT ( 'NONE',  ( 62.72729074377712521, -37.49987598507249942, -5.141182161264383765 ) ) ;
#39749=CARTESIAN_POINT ( 'NONE',  ( 108.0517077545248696, -7.250697342233347165, -7.631215200338321125 ) ) ;
#39756=CARTESIAN_POINT ( 'NONE',  ( 109.2294485933674935, -10.43672253586468557, -13.07966451788000128 ) ) ;
#39758=CARTESIAN_POINT ( 'NONE',  ( 113.8857702545248003, 0.1403307496149616695, -11.32035403202665336 ) ) ;
#39759=CARTESIAN_POINT ( 'NONE',  ( 106.9404577545248145, -7.250697342233347165, -7.631215200338321125 ) ) ;
#39761=CARTESIAN_POINT ( 'NONE',  ( 143.3676850761856940, -69.76310523276724496, -16.89321520033831447 ) ) ;
#39762=CARTESIAN_POINT ( 'NONE',  ( 69.23472380947923455, -25.80888859862148621, -5.871751884747615335 ) ) ;
#39772=EDGE_CURVE ( 'NONE', #44361, #9168, #8116, .T. ) ;
#39777=CARTESIAN_POINT ( 'NONE',  ( 105.5513952545248060, 0.8980012041604421569, -11.00651665394454071 ) ) ;
#39780=CARTESIAN_POINT ( 'NONE',  ( 115.1359265045248605, -2.791137627527939813, -8.388885654883777576 ) ) ;
#39788=CARTESIAN_POINT ( 'NONE',  ( 111.5938171295247940, 0.1403307496149613920, -13.39321520033831447 ) ) ;
#39798=ORIENTED_EDGE ( 'NONE', *, *, #11680, .F. ) ;
#39799=CARTESIAN_POINT ( 'NONE',  ( 114.7411459279789909, 0.1843591316377651834, -14.64321520033831447 ) ) ;
#39801=CARTESIAN_POINT ( 'NONE',  ( 108.7462390045248242, -9.868328341294098749, -11.32035403202665869 ) ) ;
#39809=CARTESIAN_POINT ( 'NONE',  ( 109.0935046295247872, -4.863998795839590272, -7.631215200338315796 ) ) ;
#39812=DIRECTION ( 'NONE',  ( 0.9848077530122080203, -0.1736481776669309973, 0.000000000000000000 ) ) ;
#39813=CARTESIAN_POINT ( 'NONE',  ( 87.44708369096657918, -21.99489077589588604, -18.39321520033831803 ) ) ;
#39814=CARTESIAN_POINT ( 'NONE',  ( 114.5803015045248117, -2.477300249445798297, -7.631215200338321125 ) ) ;
#39816=CARTESIAN_POINT ( 'NONE',  ( 78.69189222814998175, -59.80879295971297438, 0.4535904759388441621 ) ) ;
#39819=CARTESIAN_POINT ( 'NONE',  ( 108.7462390045248242, 0.8980012041604421569, -15.77991374673208469 ) ) ;
#39827=VECTOR ( 'NONE', #36713, 1000.000000000000000 ) ;
#39835=CARTESIAN_POINT ( 'NONE',  ( 107.5655358795247736, -0.7896495226426338832, -17.46756447353520159 ) ) ;
#39848=CARTESIAN_POINT ( 'NONE',  ( 64.28107022230250323, -36.18796843822551779, -5.721420406450495655 ) ) ;
#39859=CARTESIAN_POINT ( 'NONE',  ( 113.0523327545247838, -6.936859964151250502, -8.388885654883777576 ) ) ;
#39861=ORIENTED_EDGE ( 'NONE', *, *, #8323, .F. ) ;
#39863=CARTESIAN_POINT ( 'NONE',  ( 116.2471765045247594, -7.250697342233347165, -19.15521520033831138 ) ) ;
#39864=CARTESIAN_POINT ( 'NONE',  ( 108.2600671295247992, 0.1403307496149613920, -13.39321520033831447 ) ) ;
#39868=CARTESIAN_POINT ( 'NONE',  ( 116.6638952545248031, -9.868328341294098749, -15.46607636864997204 ) ) ;
#39869=ORIENTED_EDGE ( 'NONE', *, *, #15015, .F. ) ;
#39873=DIRECTION ( 'NONE',  ( -1.000000000000000000, 0.000000000000000000, 0.000000000000000000 ) ) ;
#39874=CARTESIAN_POINT ( 'NONE',  ( 109.4407702545248355, 0.1403307496149616695, -11.32035403202665336 ) ) ;
#39883=( BOUNDED_CURVE ( )  B_SPLINE_CURVE ( 2, ( #16410, #40123, #12767, #26667, #18919, #36239, #33714, #9566, #15501, #15731, #16185, #5005, #9113, #43548, #1579, #22562, #44235 ),
 .UNSPECIFIED., .F., .T. ) 
 B_SPLINE_CURVE_WITH_KNOTS ( ( 3, 2, 2, 2, 2, 2, 2, 2, 3 ),
 ( 0.5040431156034950178, 0.5124999999999999556, 0.5250000000000000222, 0.5374999999999999778, 0.5500000000000000444, 0.5625000000000000000, 0.5749999999999999556, 0.5875000000000000222, 0.5959568843965060703 ),
 .UNSPECIFIED. ) 
 CURVE ( )  GEOMETRIC_REPRESENTATION_ITEM ( )  RATIONAL_B_SPLINE_CURVE ( ( 0.9666851417651740608, 0.9485006404992010198, 1.000000000000000000, 0.9238795325112869605, 1.000000000000000000, 0.9238795325112869605, 1.000000000000000000, 0.9238795325112869605, 1.000000000000000000, 0.9238795325112869605, 1.000000000000000000, 0.9238795325112869605, 1.000000000000000000, 0.9238795325112869605, 1.000000000000000000, 0.9485006404991980222, 0.9666851417651760592 ) ) 
 REPRESENTATION_ITEM ( '' )  );
#39886=CARTESIAN_POINT ( 'NONE',  ( 109.7880358795247986, -8.402594152722688392, -9.854619843455216355 ) ) ;
#39894=CARTESIAN_POINT ( 'NONE',  ( 111.1076452545248259, -9.868328341294102302, -15.46607636865001645 ) ) ;
#39898=DIRECTION ( 'NONE',  ( 0.000000000000000000, 0.000000000000000000, 1.000000000000000000 ) ) ;
#39899=DIRECTION ( 'NONE',  ( 0.000000000000000000, 0.000000000000000000, 1.000000000000000000 ) ) ;
#39900=CARTESIAN_POINT ( 'NONE',  ( 84.86020291624612355, -30.49489077589588604, -12.39321520033835000 ) ) ;
#39908=CARTESIAN_POINT ( 'NONE',  ( 116.6781481986166824, -8.393872295391240357, -17.05164434167983956 ) ) ;
#39910=DIRECTION ( 'NONE',  ( 0.9387755102040806765, -0.3445294493088623122, 0.000000000000000000 ) ) ;
#39915=CARTESIAN_POINT ( 'NONE',  ( 110.8298327545248299, -2.477300249445798297, -19.15521520033831138 ) ) ;
#39916=CARTESIAN_POINT ( 'NONE',  ( 110.6909265045248247, -2.791137627527939813, -8.388885654883777576 ) ) ;
#39917=CARTESIAN_POINT ( 'NONE',  ( 108.4684265045248424, -2.791137627527939813, -8.388885654883777576 ) ) ;
#39922=CARTESIAN_POINT ( 'NONE',  ( 107.4266296295248821, -4.863998795839590272, -19.15521520033831493 ) ) ;
#39923=CARTESIAN_POINT ( 'NONE',  ( 69.69189222814998175, -41.76310523276723785, -20.39321520033831447 ) ) ;
#39925=EDGE_CURVE ( 'NONE', #43568, #35835, #13667, .T. ) ;
#39928=CARTESIAN_POINT ( 'NONE',  ( 109.5796765045248122, -7.250697342233347165, -19.15521520033831138 ) ) ;
#39931=CARTESIAN_POINT ( 'NONE',  ( 110.7585566399283863, 0.4261359969231631739, -14.64321520033831447 ) ) ;
#39938=ORIENTED_EDGE ( 'NONE', *, *, #17211, .F. ) ;
#39944=CARTESIAN_POINT ( 'NONE',  ( 110.8996837908067761, 0.5115630086001619059, -12.14321520033833224 ) ) ;
#39946=CARTESIAN_POINT ( 'NONE',  ( 116.0388171295248014, -10.62599879583958540, -13.39321520033831447 ) ) ;
#39954=CARTESIAN_POINT ( 'NONE',  ( 62.13589673425203586, -65.32615175216918146, -44.81351878150378809 ) ) ;
#39955=CARTESIAN_POINT ( 'NONE',  ( 108.5378796295247810, -4.863998795839590272, -19.15521520033831493 ) ) ;
#39957=( BOUNDED_SURFACE ( )  B_SPLINE_SURFACE ( 3, 2, ( 
 ( #41616, #3512, #25169 ),
 ( #7837, #21291, #31770 ),
 ( #39067, #21743, #24708 ),
 ( #38834, #42055, #31322 ),
 ( #6946, #38598, #41834 ),
 ( #35174, #7602, #20850 ),
 ( #21517, #96, #4179 ),
 ( #35632, #542, #14454 ),
 ( #31104, #31548, #3952 ),
 ( #17429, #45029, #13787 ) ),
 .UNSPECIFIED., .F., .F., .F. ) 
 B_SPLINE_SURFACE_WITH_KNOTS ( ( 4, 2, 2, 2, 4 ),
 ( 3, 3 ),
 ( 3.141592653589795336, 3.534291735288519920, 3.926990816987240063, 4.319689898685965090, 4.712388980384689674 ),
 ( 0.000000000000000000, 1.000000000000000000 ),
 .UNSPECIFIED. ) 
 GEOMETRIC_REPRESENTATION_ITEM ( )  RATIONAL_B_SPLINE_SURFACE ( (
 ( 1.000000000000000000, 0.8199175108841310067, 1.000000000000000000),
 ( 1.000000000000000000, 0.8199255829187760414, 1.000000000000000000),
 ( 1.000000000000000000, 0.8171960459197700199, 1.000000000000000000),
 ( 1.000000000000000000, 0.8065673029484310419, 1.000000000000000000),
 ( 1.000000000000000000, 0.7986592547571330636, 1.000000000000000000),
 ( 1.000000000000000000, 0.7784387827311890495, 1.000000000000000000),
 ( 1.000000000000000000, 0.7661249975918460464, 1.000000000000000000),
 ( 1.000000000000000000, 0.7384318888118330815, 1.000000000000000000),
 ( 1.000000000000000000, 0.7230611114418840080, 1.000000000000000000),
 ( 1.000000000000000000, 0.7071067811865480168, 1.000000000000000000) ) ) 
 REPRESENTATION_ITEM ( '' )  SURFACE ( )  );
#39962=FACE_BOUND ( 'NONE', #40208, .T. ) ;
#39966=CARTESIAN_POINT ( 'NONE',  ( 114.0941296295247867, -4.863998795839590272, -19.15521520033831493 ) ) ;
#39968=CARTESIAN_POINT ( 'NONE',  ( 112.4967077545247633, -7.250697342233347165, -7.631215200338321125 ) ) ;
#39973=CARTESIAN_POINT ( 'NONE',  ( 109.5102233795247884, -8.938348069036489818, -17.46756447353520159 ) ) ;
#39976=FACE_OUTER_BOUND ( 'NONE', #5883, .T. ) ;
#39977=CARTESIAN_POINT ( 'NONE',  ( 116.7592683588497096, -11.76435134077275890, -6.215002696414487993 ) ) ;
#39980=CARTESIAN_POINT ( 'NONE',  ( 109.4154010812577837, -0.01829820670803256055, -12.14321520033831625 ) ) ;
#39982=CARTESIAN_POINT ( 'NONE',  ( 110.1353015045248469, -6.936859964151250502, -18.39754474579286025 ) ) ;
#39983=CARTESIAN_POINT ( 'NONE',  ( 105.8986608795248401, -8.938348069036489818, -9.318865927141430916 ) ) ;
#39986=CARTESIAN_POINT ( 'NONE',  ( 71.41205933791314919, -25.41584841807908646, -5.221760208415934024 ) ) ;
#39993=EDGE_CURVE ( 'NONE', #40407, #31774, #9241, .T. ) ;
#39995=EDGE_LOOP ( 'NONE', ( #30802, #2029, #39047, #31796 ) ) ;
#39999=B_SPLINE_CURVE_WITH_KNOTS ( 'NONE', 3,
 ( #25492, #19319, #19089, #33204, #36402, #8384, #22066, #5621, #36184, #28912 ),
 .UNSPECIFIED., .F., .F.,
 ( 4, 3, 3, 4 ),
 ( 0.000000000000000000, 0.0002476487219222714723, 0.0004952974148303440237, 0.0009534114850261710648 ),
 .UNSPECIFIED. ) ;
#40004=CARTESIAN_POINT ( 'NONE',  ( 107.3571765045248299, -2.791137627527939813, -8.388885654883777576 ) ) ;
#40005=VECTOR ( 'NONE', #14480, 1000.000000000000000 ) ;
#40006=CARTESIAN_POINT ( 'NONE',  ( 64.61935771200890599, -37.86087448816891765, -4.893215200338314474 ) ) ;
#40007=AXIS2_PLACEMENT_3D ( 'NONE', #6456, #12850, #9194 ) ;
#40012=ORIENTED_EDGE ( 'NONE', *, *, #9982, .F. ) ;
#40013=CARTESIAN_POINT ( 'NONE',  ( 117.1532421295247843, 0.1360012041604560795, -13.39321520033831447 ) ) ;
#40014=CARTESIAN_POINT ( 'NONE',  ( 110.9687390045248350, -9.868328341294098749, -11.32035403202665869 ) ) ;
#40025=B_SPLINE_CURVE_WITH_KNOTS ( 'NONE', 3,
 ( #18056, #14409, #28319, #42231, #28551, #24896, #38789, #4359, #18279, #9772, #23684, #37339, #6568, #6343, #9539 ),
 .UNSPECIFIED., .F., .F.,
 ( 4, 2, 2, 1, 1, 1, 2, 2, 4 ),
 ( 0.000000000000000000, 0.2500000000001662559, 0.3750000000002411404, 0.4375000000002858269, 0.4687500000003081979, 0.4843750000003191891, 0.4921875000003183565, 0.5000000000003175238, 1.000000000000000000 ),
 .UNSPECIFIED. ) ;
#40026=CARTESIAN_POINT ( 'NONE',  ( 111.9410827545248708, -6.936859964151250502, -8.388885654883777576 ) ) ;
#40030=CARTESIAN_POINT ( 'NONE',  ( 106.3848327545248651, -2.477300249445798297, -19.15521520033831138 ) ) ;
#40031=DIRECTION ( 'NONE',  ( -1.000000000000000000, 0.000000000000000000, 0.000000000000000000 ) ) ;
#40032=CARTESIAN_POINT ( 'NONE',  ( 63.31042565271481948, -20.21815917793063733, -0.8932152003383146965 ) ) ;
#40034=CARTESIAN_POINT ( 'NONE',  ( 111.0381921295247878, 0.8980012041604618078, -13.39321520033831447 ) ) ;
#40035=CARTESIAN_POINT ( 'NONE',  ( 116.4429452033932932, 2.229392703617450788, -20.41770221837591137 ) ) ;
#40036=CARTESIAN_POINT ( 'NONE',  ( 83.86179762071230925, -31.76409560463467585, -23.03138878092153519 ) ) ;
#40039=CARTESIAN_POINT ( 'NONE',  ( 106.0375671295248310, -10.62599879583958540, -13.39321520033831447 ) ) ;
#40043=CARTESIAN_POINT ( 'NONE',  ( 116.4587108795247730, -8.399532701772287169, -9.857681294405580275 ) ) ;
#40051=CARTESIAN_POINT ( 'NONE',  ( 108.9545983795247821, -0.7896495226426338832, -9.318865927141430916 ) ) ;
#40056=VERTEX_POINT ( 'NONE', #28359 ) ;
#40060=EDGE_CURVE ( 'NONE', #40384, #38773, #6598, .T. ) ;
#40063=CARTESIAN_POINT ( 'NONE',  ( 61.69189222814998175, -49.76310523276723785, -24.89321520033831447 ) ) ;
#40066=LINE ( 'NONE', #12267, #1967 ) ;
#40069=CARTESIAN_POINT ( 'NONE',  ( 109.6956031537514917, 0.4930828106259610433, -14.64321520033831447 ) ) ;
#40071=CYLINDRICAL_SURFACE ( 'NONE', #28940, 3.000000000000001332 ) ;
#40077=ADVANCED_FACE ( 'NONE', ( #28591 ), #39957, .F. ) ;
#40078=VERTEX_POINT ( 'NONE', #10372 ) ;
#40081=CARTESIAN_POINT ( 'NONE',  ( 116.5944421295247793, -9.868328341294093420, -13.39321520033831447 ) ) ;
#40083=EDGE_CURVE ( 'NONE', #20305, #3693, #316, .T. ) ;
#40087=CARTESIAN_POINT ( 'NONE',  ( 114.5108483795247878, -0.7896495226426338832, -9.318865927141430916 ) ) ;
#40088=CARTESIAN_POINT ( 'NONE',  ( 107.6349890045248401, -9.868328341294098749, -11.32035403202665869 ) ) ;
#40093=CARTESIAN_POINT ( 'NONE',  ( 114.8581140045248361, 0.1403307496149616695, -15.46607636864997204 ) ) ;
#40094=ORIENTED_EDGE ( 'NONE', *, *, #24720, .F. ) ;
#40100=CARTESIAN_POINT ( 'NONE',  ( 107.7044421295247929, -9.868328341294093420, -13.39321520033831447 ) ) ;
#40101=ORIENTED_EDGE ( 'NONE', *, *, #36464, .T. ) ;
#40109=CARTESIAN_POINT ( 'NONE',  ( 112.4967077545247633, -2.791137627527939813, -18.39754474579286025 ) ) ;
#40123=CARTESIAN_POINT ( 'NONE',  ( 110.3894297178593575, -0.3595008806742686081, -15.96590799893916213 ) ) ;
#40141=CARTESIAN_POINT ( 'NONE',  ( 112.4272546295247821, -4.863998795839590272, -7.631215200338315796 ) ) ;
#40142=CARTESIAN_POINT ( 'NONE',  ( 109.9963952545248134, -9.868328341294098749, -15.46607636864997204 ) ) ;
#40143=CARTESIAN_POINT ( 'NONE',  ( 107.2182702545248105, 0.1403307496149616695, -11.32035403202665336 ) ) ;
#40144=AXIS2_PLACEMENT_3D ( 'NONE', #19266, #33596, #2372 ) ;
#40150=CARTESIAN_POINT ( 'NONE',  ( 84.86020291624612355, -30.49489077589588604, -18.39321520033831803 ) ) ;
#40155=CARTESIAN_POINT ( 'NONE',  ( 108.8156921295247912, 0.8980012041604618078, -13.39321520033831447 ) ) ;
#40173=CARTESIAN_POINT ( 'NONE',  ( 113.8163171295247764, -10.62599879583958540, -13.39321520033831447 ) ) ;
#40182=ORIENTED_EDGE ( 'NONE', *, *, #39993, .T. ) ;
#40183=CARTESIAN_POINT ( 'NONE',  ( 71.36400868967236022, -24.42718413923373788, -4.893215200338314474 ) ) ;
#40185=CARTESIAN_POINT ( 'NONE',  ( 76.69189222814998175, -49.76310523276723785, -19.39321520033831447 ) ) ;
#40186=VECTOR ( 'NONE', #31881, 1000.000000000000000 ) ;
#40195=CARTESIAN_POINT ( 'NONE',  ( 113.1217858795247935, -0.7896495226426338832, -17.46756447353520159 ) ) ;
#40197=CARTESIAN_POINT ( 'NONE',  ( 114.0246765045248196, -7.250697342233347165, -19.15521520033831138 ) ) ;
#40202=CARTESIAN_POINT ( 'NONE',  ( 63.51630259865831363, -37.86186143294432327, -4.893262514330128710 ) ) ;
#40203=CARTESIAN_POINT ( 'NONE',  ( 109.4407702545248355, -10.62599879583958717, -15.77991374673208469 ) ) ;
#40207=CARTESIAN_POINT ( 'NONE',  ( 117.2294421295247844, -10.84261285664941177, -5.229271512936652933 ) ) ;
#40208=EDGE_LOOP ( 'NONE', ( #17632, #17655 ) ) ;
#40210=CARTESIAN_POINT ( 'NONE',  ( 109.2294347450687866, -10.29077967592130349, -14.42818681898541300 ) ) ;
#40214=CARTESIAN_POINT ( 'NONE',  ( 110.0658483795247804, -8.402594152722688392, -16.93181055722141792 ) ) ;
#40215=CARTESIAN_POINT ( 'NONE',  ( 109.2324108795247923, -1.325403438956436419, -16.93181055722141792 ) ) ;
#40218=CARTESIAN_POINT ( 'NONE',  ( 69.63874157094764428, -25.41500789246203951, -5.785566283887345840 ) ) ;
#40233=CARTESIAN_POINT ( 'NONE',  ( 106.0375671295248310, -10.62599879583958540, -13.39321520033831447 ) ) ;
#40236=CARTESIAN_POINT ( 'NONE',  ( 109.7185827545247889, -6.936859964151250502, -8.388885654883777576 ) ) ;
#40243=CARTESIAN_POINT ( 'NONE',  ( 116.4555358795247884, -8.402594152722688392, -9.854619843455216355 ) ) ;
#40244=CARTESIAN_POINT ( 'NONE',  ( 108.1211608795247798, -1.325403438956436419, -16.93181055722141792 ) ) ;
#40249=CARTESIAN_POINT ( 'NONE',  ( 61.69189222814998175, -61.90644496644519990, -36.30514255143466329 ) ) ;
#40258=CARTESIAN_POINT ( 'NONE',  ( 108.9545983795247821, -8.402594152722688392, -16.93181055722141792 ) ) ;
#40262=CARTESIAN_POINT ( 'NONE',  ( 115.9693640045247776, 0.1403307496149616695, -15.46607636864997204 ) ) ;
#40266=CARTESIAN_POINT ( 'NONE',  ( 110.2742077545248094, -7.250697342233347165, -7.631215200338321125 ) ) ;
#40268=CARTESIAN_POINT ( 'NONE',  ( 114.8581140045248361, -10.62599879583958717, -11.00651665394454604 ) ) ;
#40273=DIRECTION ( 'NONE',  ( 0.000000000000000000, -0.3713878862591665220, 0.9284778069183713400 ) ) ;
#40274=EDGE_LOOP ( 'NONE', ( #2919, #40101, #22885, #14207 ) ) ;
#40275=CARTESIAN_POINT ( 'NONE',  ( 109.2294421295247844, 0.2400687412228638684, -12.14321520033831625 ) ) ;
#40286=CARTESIAN_POINT ( 'NONE',  ( 110.6909265045248247, -7.250697342233347165, -19.15521520033831138 ) ) ;
#40289=CARTESIAN_POINT ( 'NONE',  ( 116.7891407172877791, -3.223887174354909568, -18.32229490764988000 ) ) ;
#40296=DIRECTION ( 'NONE',  ( 0.000000000000000000, 1.000000000000000000, 0.000000000000000000 ) ) ;
#40306=CARTESIAN_POINT ( 'NONE',  ( 62.22678445075433018, -36.72958069525633817, -5.531797115907686191 ) ) ;
#40310=CARTESIAN_POINT ( 'NONE',  ( 116.8028015045247940, -6.936859964151250502, -18.39754474579286025 ) ) ;
#40314=CARTESIAN_POINT ( 'NONE',  ( 115.9693640045247776, -10.62599879583958717, -11.00651665394454604 ) ) ;
#40315=CARTESIAN_POINT ( 'NONE',  ( 110.5520202545248054, 0.1403307496149616695, -11.32035403202665336 ) ) ;
#40321=CARTESIAN_POINT ( 'NONE',  ( 111.5243640045248412, 0.1403307496149616695, -15.46607636864997204 ) ) ;
#40327=DIRECTION ( 'NONE',  ( -0.9970811988817437355, 0.07634843047859309062, -9.125038414728249219E-18 ) ) ;
#40328=CARTESIAN_POINT ( 'NONE',  ( 116.8800879763089995, -11.65005305785124712, -21.48974400451860234 ) ) ;
#40334=CARTESIAN_POINT ( 'NONE',  ( 117.2294421295247844, 0.2335149919452661482, -4.893215200338314474 ) ) ;
#40337=CARTESIAN_POINT ( 'NONE',  ( 111.5938171295247940, 0.1403307496149613920, -13.39321520033831447 ) ) ;
#40343=ADVANCED_FACE ( 'NONE', ( #32217 ), #12007, .T. ) ;
#40351=DIRECTION ( 'NONE',  ( 0.000000000000000000, 0.000000000000000000, -1.000000000000000000 ) ) ;
#40365=ORIENTED_EDGE ( 'NONE', *, *, #341, .F. ) ;
#40367=CARTESIAN_POINT ( 'NONE',  ( 113.5385046295247804, -4.863998795839590272, -7.631215200338315796 ) ) ;
#40369=CARTESIAN_POINT ( 'NONE',  ( 108.0517077545248696, -2.791137627527939813, -18.39754474579286025 ) ) ;
#40370=CARTESIAN_POINT ( 'NONE',  ( 110.6214733795247867, -1.325403438956436419, -9.854619843455211026 ) ) ;
#40371=CARTESIAN_POINT ( 'NONE',  ( 64.33868347142437472, -36.47288101306110519, -5.626337088425048982 ) ) ;
#40374=LINE ( 'NONE', #9137, #17292 ) ;
#40379=CARTESIAN_POINT ( 'NONE',  ( 105.2041296295248287, -4.863998795839590272, -8.388885654883775800 ) ) ;
#40382=CARTESIAN_POINT ( 'NONE',  ( 108.1906140045248463, -10.62599879583958717, -11.00651665394454604 ) ) ;
#40384=VERTEX_POINT ( 'NONE', #34057 ) ;
#40385=FACE_BOUND ( 'NONE', #12596, .T. ) ;
#40393=EDGE_LOOP ( 'NONE', ( #28758, #2064 ) ) ;
#40398=ORIENTED_EDGE ( 'NONE', *, *, #28135, .T. ) ;
#40401=ADVANCED_FACE ( 'NONE', ( #41599 ), #2824, .F. ) ;
#40402=EDGE_CURVE ( 'NONE', #38575, #38752, #7108, .T. ) ;
#40405=CARTESIAN_POINT ( 'NONE',  ( 111.4549108795247747, -8.938348069036489818, -9.318865927141430916 ) ) ;
#40407=VERTEX_POINT ( 'NONE', #6927 ) ;
#40415=CARTESIAN_POINT ( 'NONE',  ( 84.39081516114413262, -30.32262605124143562, -18.39321520033831803 ) ) ;
#40419=( BOUNDED_CURVE ( )  B_SPLINE_CURVE ( 3, ( #24075, #27270, #17013, #2626 ),
 .UNSPECIFIED., .F., .F. ) 
 B_SPLINE_CURVE_WITH_KNOTS ( ( 4, 4 ),
 ( 1.570796326794895004, 2.115579167352664935 ),
 .UNSPECIFIED. ) 
 CURVE ( )  GEOMETRIC_REPRESENTATION_ITEM ( )  RATIONAL_B_SPLINE_CURVE ( ( 1.000000000000000000, 0.9754201827720950790, 0.9754201827720950790, 1.000000000000000000 ) ) 
 REPRESENTATION_ITEM ( '' )  );
#40427=CARTESIAN_POINT ( 'NONE',  ( 114.1635827545248389, -2.477300249445798297, -19.15521520033831138 ) ) ;
#40428=CARTESIAN_POINT ( 'NONE',  ( 112.2188952545247531, -9.868328341294098749, -15.46607636864997204 ) ) ;
#40429=CARTESIAN_POINT ( 'NONE',  ( 109.8574890045247940, 0.8980012041604421569, -15.77991374673208469 ) ) ;
#40434=CARTESIAN_POINT ( 'NONE',  ( 108.1211608795247798, -8.938348069036489818, -9.318865927141430916 ) ) ;
#40438=DIRECTION ( 'NONE',  ( 0.000000000000000000, 0.000000000000000000, 1.000000000000000000 ) ) ;
#40444=CARTESIAN_POINT ( 'NONE',  ( 116.5249890045247980, 0.8980012041604421569, -15.77991374673208469 ) ) ;
#40445=CARTESIAN_POINT ( 'NONE',  ( 109.4407702545248355, 0.1403307496149616695, -11.32035403202665336 ) ) ;
#40448=CARTESIAN_POINT ( 'NONE',  ( 68.96140303619711176, -25.88415598586878730, -5.893215200338315363 ) ) ;
#40465=CARTESIAN_POINT ( 'NONE',  ( 106.2459265045248173, -7.250697342233347165, -19.15521520033831138 ) ) ;
#40469=CARTESIAN_POINT ( 'NONE',  ( 87.44708369096657918, -29.99489077589588959, -18.39321520033831803 ) ) ;
#40470=CARTESIAN_POINT ( 'NONE',  ( 108.3295202545248657, 0.1403307496149616695, -11.32035403202665336 ) ) ;
#40476=CARTESIAN_POINT ( 'NONE',  ( 116.8059765045247502, -6.935066607705044461, -18.39321520033830737 ) ) ;
#40479=B_SPLINE_CURVE_WITH_KNOTS ( 'NONE', 3,
 ( #14519, #32289, #35008, #39365, #35700, #28659, #13470, #4018, #3790, #17716 ),
 .UNSPECIFIED., .F., .F.,
 ( 4, 3, 3, 4 ),
 ( 0.000000000000000000, 0.0002476487219222729902, 0.0004952974148303419637, 0.0009534114850261800637 ),
 .UNSPECIFIED. ) ;
#40489=CARTESIAN_POINT ( 'NONE',  ( 111.1076452545248259, -9.868328341294098749, -15.46607636864997204 ) ) ;
#40493=CARTESIAN_POINT ( 'NONE',  ( 105.7597546295248350, -4.863998795839590272, -7.631215200338315796 ) ) ;
#40497=CARTESIAN_POINT ( 'NONE',  ( 110.5520202545248054, -10.62599879583958717, -15.77991374673208469 ) ) ;
#40499=CARTESIAN_POINT ( 'NONE',  ( 115.9693640045247776, -10.62599879583958717, -11.00651665394454604 ) ) ;
#40502=CARTESIAN_POINT ( 'NONE',  ( 111.8215301496069998, 0.3591747506842615789, -14.64321520033831447 ) ) ;
#40515=CARTESIAN_POINT ( 'NONE',  ( 107.9128015045248219, -2.477300249445798297, -7.631215200338321125 ) ) ;
#40518=CARTESIAN_POINT ( 'NONE',  ( 110.1353015045248185, -2.477300249445851144, -7.631215200338310467 ) ) ;
#40525=CARTESIAN_POINT ( 'NONE',  ( 113.2606921295247702, -9.868328341294093420, -13.39321520033836421 ) ) ;
#40528=CARTESIAN_POINT ( 'NONE',  ( 106.5931921295248372, -9.868328341294093420, -13.39321520033831447 ) ) ;
#40540=CARTESIAN_POINT ( 'NONE',  ( 116.7333483795247844, -8.402594152722688392, -16.93181055722141792 ) ) ;
#40544=CARTESIAN_POINT ( 'NONE',  ( 106.0375671295248310, 0.1403307496149613920, -13.39321520033831447 ) ) ;
#40545=CARTESIAN_POINT ( 'NONE',  ( 109.7185827545247889, -6.936859964151250502, -8.388885654883777576 ) ) ;
#40546=CARTESIAN_POINT ( 'NONE',  ( 82.82366151329020454, -31.79927569882703153, -23.15978140744613256 ) ) ;
#40549=CARTESIAN_POINT ( 'NONE',  ( 117.2294421295247844, 7.836001204160461420, -14.64321520033831447 ) ) ;
#40551=CARTESIAN_POINT ( 'NONE',  ( 114.7886608795247696, -1.325403438956436419, -16.93181055722141792 ) ) ;
#40559=CARTESIAN_POINT ( 'NONE',  ( 76.69189222814998175, -49.76310523276723785, -7.393215200338315363 ) ) ;
#40568=CARTESIAN_POINT ( 'NONE',  ( 110.4825671295247815, 0.1403307496149613920, -13.39321520033831447 ) ) ;
#40571=ORIENTED_EDGE ( 'NONE', *, *, #21238, .F. ) ;
#40576=VERTEX_POINT ( 'NONE', #3498 ) ;
#40597=CARTESIAN_POINT ( 'NONE',  ( 111.4549108795247747, -8.938348069036489818, -9.318865927141430916 ) ) ;
#40598=CARTESIAN_POINT ( 'NONE',  ( 105.8986608795248401, -1.325403438956436419, -16.93181055722141792 ) ) ;
#40599=CARTESIAN_POINT ( 'NONE',  ( 111.1770983795247787, -8.402594152722688392, -16.93181055722141792 ) ) ;
#40600=CARTESIAN_POINT ( 'NONE',  ( 109.2294421295247844, -8.865838614420134434, -9.247624522711900497 ) ) ;
#40602=EDGE_LOOP ( 'NONE', ( #17759, #22830, #10410, #21145 ) ) ;
#40607=CARTESIAN_POINT ( 'NONE',  ( 105.7597546295248350, -4.863998795839590272, -18.39754474579285315 ) ) ;
#40609=CARTESIAN_POINT ( 'NONE',  ( 114.9275671295247889, 0.1403307496149613920, -13.39321520033831447 ) ) ;
#40625=VERTEX_POINT ( 'NONE', #7140 ) ;
#40628=CARTESIAN_POINT ( 'NONE',  ( 112.5661608795247872, -8.938348069036489818, -9.318865927141430916 ) ) ;
#40637=VERTEX_POINT ( 'NONE', #35453 ) ;
#40640=CARTESIAN_POINT ( 'NONE',  ( 107.9128015045248219, -2.477300249445798297, -7.631215200338321125 ) ) ;
#40648=FACE_OUTER_BOUND ( 'NONE', #23333, .T. ) ;
#40651=CARTESIAN_POINT ( 'NONE',  ( 114.9275671295247889, -10.62599879583958540, -13.39321520033831447 ) ) ;
#40652=CARTESIAN_POINT ( 'NONE',  ( 111.4549108795247747, -1.325403438956436419, -16.93181055722141792 ) ) ;
#40653=CARTESIAN_POINT ( 'NONE',  ( 112.0105358795247810, -0.7896495226426338832, -17.46756447353520159 ) ) ;
#40668=VERTEX_POINT ( 'NONE', #20911 ) ;
#40672=CARTESIAN_POINT ( 'NONE',  ( 107.4266296295248821, -4.863998795839590272, -8.388885654883775800 ) ) ;
#40673=CARTESIAN_POINT ( 'NONE',  ( 111.7327233795247849, -1.325403438956436419, -9.854619843455211026 ) ) ;
#40676=CARTESIAN_POINT ( 'NONE',  ( 71.45846722029260434, -25.75860963767633649, -5.221760208414266025 ) ) ;
#40678=B_SPLINE_CURVE_WITH_KNOTS ( 'NONE', 3,
 ( #450, #14141, #4316, #21653, #42413, #17787, #32131, #4084, #28951, #42189 ),
 .UNSPECIFIED., .F., .F.,
 ( 4, 3, 3, 4 ),
 ( 0.000000000000000000, 0.0002476486447138930014, 0.0004952972925464250303, 0.0009604418836934749786 ),
 .UNSPECIFIED. ) ;
#40686=ORIENTED_EDGE ( 'NONE', *, *, #4400, .F. ) ;
#40691=CARTESIAN_POINT ( 'NONE',  ( 108.5378796295247810, -4.863998795839590272, -19.15521520033831493 ) ) ;
#40695=CARTESIAN_POINT ( 'NONE',  ( 109.3713171295247832, 0.1403307496149613920, -13.39321520033831447 ) ) ;
#40701=CARTESIAN_POINT ( 'NONE',  ( 116.0419921295247860, 0.1360012041604560795, -13.39321520033831447 ) ) ;
#40710=CARTESIAN_POINT ( 'NONE',  ( 114.5984981608379769, 0.3867979994853637526, -14.64321520033831447 ) ) ;
#40712=CARTESIAN_POINT ( 'NONE',  ( 107.4960827545248350, -6.936859964151250502, -8.388885654883777576 ) ) ;
#40717=CARTESIAN_POINT ( 'NONE',  ( 112.4272546295247821, -4.863998795839590272, -18.39754474579285315 ) ) ;
#40722=CARTESIAN_POINT ( 'NONE',  ( 112.1494421295248003, 0.8980012041604618078, -13.39321520033831447 ) ) ;
#40724=CARTESIAN_POINT ( 'NONE',  ( 112.0105358795247810, -0.7896495226426338832, -17.46756447353520159 ) ) ;
#40731=ORIENTED_EDGE ( 'NONE', *, *, #8067, .F. ) ;
#40741=CARTESIAN_POINT ( 'NONE',  ( 110.7603796295247918, -4.863998795839590272, -19.15521520033831493 ) ) ;
#40744=CARTESIAN_POINT ( 'NONE',  ( 116.8434081373642641, -0.9077462878304770610, -16.84372492951588995 ) ) ;
#40750=CARTESIAN_POINT ( 'NONE',  ( 113.7231797178594093, -0.3595008806742178709, -15.96590799893916568 ) ) ;
#40752=CARTESIAN_POINT ( 'NONE',  ( 116.4388388684191256, 2.231149969025194579, -6.374051288094602086 ) ) ;
#40754=CARTESIAN_POINT ( 'NONE',  ( 106.5237390045248418, -9.868328341294098749, -11.32035403202665869 ) ) ;
#40765=CARTESIAN_POINT ( 'NONE',  ( 116.3166296295247832, -4.863998795839590272, -8.388885654883775800 ) ) ;
#40769=CARTESIAN_POINT ( 'NONE',  ( 111.8021765045248372, -7.250697342233347165, -19.15521520033831138 ) ) ;
#40770=CARTESIAN_POINT ( 'NONE',  ( 109.0935046295247872, -4.863998795839590272, -18.39754474579285315 ) ) ;
#40771=CARTESIAN_POINT ( 'NONE',  ( 116.2471765045247594, -7.250697342233347165, -19.15521520033831138 ) ) ;
#40774=EDGE_CURVE ( 'NONE', #36801, #6063, #18154, .T. ) ;
#40776=CARTESIAN_POINT ( 'NONE',  ( 83.84865386347668448, -25.99489077589588604, -15.39321520033831625 ) ) ;
#40777=CARTESIAN_POINT ( 'NONE',  ( 113.6774108795247997, -1.325403438956436419, -16.93181055722141792 ) ) ;
#40778=VERTEX_POINT ( 'NONE', #35691 ) ;
#40785=CARTESIAN_POINT ( 'NONE',  ( 114.2330358795247776, -0.7896495226426338832, -17.46756447353520159 ) ) ;
#40789=VECTOR ( 'NONE', #27940, 1000.000000000000227 ) ;
#40797=CARTESIAN_POINT ( 'NONE',  ( 113.2606921295247702, -9.868328341294093420, -13.39321520033831447 ) ) ;
#40801=ORIENTED_EDGE ( 'NONE', *, *, #527, .F. ) ;
#40816=CARTESIAN_POINT ( 'NONE',  ( 114.3719421295247827, -9.868328341294093420, -13.39321520033831447 ) ) ;
#40817=VECTOR ( 'NONE', #28218, 1000.000000000000000 ) ;
#40820=CIRCLE ( 'NONE', #29153, 0.8718221387495408425 ) ;
#40829=CARTESIAN_POINT ( 'NONE',  ( 111.5243640045248412, -10.62599879583958717, -11.00651665394454604 ) ) ;
#40830=CARTESIAN_POINT ( 'NONE',  ( 107.5655358795247736, -8.402594152722688392, -9.854619843455216355 ) ) ;
#40831=DIRECTION ( 'NONE',  ( -0.1736481776669309696, -0.9848077530122079093, 0.000000000000000000 ) ) ;
#40833=CARTESIAN_POINT ( 'NONE',  ( 64.38113726523094726, -36.68293531231000060, -5.550475082982985420 ) ) ;
#40837=CARTESIAN_POINT ( 'NONE',  ( 117.2294421295247417, -10.75052641725357994, -21.89299348893975505 ) ) ;
#40839=FACE_OUTER_BOUND ( 'NONE', #34716, .T. ) ;
#40841=CARTESIAN_POINT ( 'NONE',  ( 114.5803015045248117, -6.936859964151250502, -18.39754474579286025 ) ) ;
#40851=DIRECTION ( 'NONE',  ( 0.000000000000000000, 0.000000000000000000, -1.000000000000000000 ) ) ;
#40863=CARTESIAN_POINT ( 'NONE',  ( 110.8298327545248299, -2.477300249445798297, -19.15521520033831138 ) ) ;
#40872=CARTESIAN_POINT ( 'NONE',  ( 106.3848327545248651, -2.477300249445798297, -19.15521520033831138 ) ) ;
#40873=CIRCLE ( 'NONE', #22625, 2.999999999999998224 ) ;
#40883=CARTESIAN_POINT ( 'NONE',  ( 107.5655358795247736, -0.7896495226426338832, -17.46756447353520159 ) ) ;
#40884=CARTESIAN_POINT ( 'NONE',  ( 112.6356140045247827, 0.1403307496149616695, -15.46607636864997204 ) ) ;
#40885=CARTESIAN_POINT ( 'NONE',  ( 105.8292077545248446, -7.250697342233347165, -7.631215200338321125 ) ) ;
#40888=VERTEX_POINT ( 'NONE', #14959 ) ;
#40889=AXIS2_PLACEMENT_3D ( 'NONE', #466, #4330, #28293 ) ;
#40897=DIRECTION ( 'NONE',  ( 0.000000000000000000, -0.9284778069183722282, -0.3713878862591645791 ) ) ;
#40904=CARTESIAN_POINT ( 'NONE',  ( 109.5796765045248122, -2.791137627527939813, -8.388885654883777576 ) ) ;
#40905=CARTESIAN_POINT ( 'NONE',  ( 113.0523327545247838, -6.936859964151250502, -8.388885654883777576 ) ) ;
#40916=ORIENTED_EDGE ( 'NONE', *, *, #29962, .T. ) ;
#40918=AXIS2_PLACEMENT_3D ( 'NONE', #30394, #3025, #44765 ) ;
#40922=EDGE_CURVE ( 'NONE', #28016, #21643, #15864, .T. ) ;
#40924=EDGE_CURVE ( 'NONE', #27136, #42526, #14095, .T. ) ;
#40929=CARTESIAN_POINT ( 'NONE',  ( 110.8992858795247827, -8.402594152722688392, -9.854619843455216355 ) ) ;
#40930=CARTESIAN_POINT ( 'NONE',  ( 64.19189222814998175, -49.76310523276725206, -29.87698278062875445 ) ) ;
#40934=ORIENTED_EDGE ( 'NONE', *, *, #39235, .T. ) ;
#40940=CARTESIAN_POINT ( 'NONE',  ( 70.29296507063932609, -26.37030337512767275, -5.626337071866863049 ) ) ;
#40946=CARTESIAN_POINT ( 'NONE',  ( 106.6626452545248611, -9.868328341294098749, -15.46607636864997204 ) ) ;
#40950=CARTESIAN_POINT ( 'NONE',  ( 112.7050671295247923, 0.1403307496149613920, -13.39321520033831447 ) ) ;
#40953=CARTESIAN_POINT ( 'NONE',  ( 65.49983523453742862, -18.16718729050178993, -4.893215200338314474 ) ) ;
#40954=CARTESIAN_POINT ( 'NONE',  ( 109.2294421295247275, -1.527404628864407199, -17.14082320569335494 ) ) ;
#40956=CARTESIAN_POINT ( 'NONE',  ( 112.2188952545247531, 0.8980012041604421569, -11.00651665394454071 ) ) ;
#40957=LINE ( 'NONE', #41414, #13187 ) ;
#40958=CARTESIAN_POINT ( 'NONE',  ( 116.0388171295248014, -10.62599879583958540, -13.39321520033831447 ) ) ;
#40961=CARTESIAN_POINT ( 'NONE',  ( 114.7886608795247696, -8.938348069036441856, -9.318865927141425587 ) ) ;
#40976=CARTESIAN_POINT ( 'NONE',  ( 90.41915846579418314, -16.87387181286558757, -6.893215200338315363 ) ) ;
#40977=CARTESIAN_POINT ( 'NONE',  ( 110.3436608795247764, -1.325403438956436419, -16.93181055722141792 ) ) ;
#40980=CARTESIAN_POINT ( 'NONE',  ( 111.8021765045248372, -7.250697342233347165, -19.15521520033831138 ) ) ;
#40986=CARTESIAN_POINT ( 'NONE',  ( 113.3995983795247895, -8.402594152722633325, -16.93181055722145345 ) ) ;
#40992=CARTESIAN_POINT ( 'NONE',  ( 106.6626452545248611, -9.868328341294098749, -15.46607636864997204 ) ) ;
#41000=ORIENTED_EDGE ( 'NONE', *, *, #44574, .T. ) ;
#41007=CARTESIAN_POINT ( 'NONE',  ( 111.7327233795247849, -8.938348069036489818, -17.46756447353520159 ) ) ;
#41008=FACE_OUTER_BOUND ( 'NONE', #21048, .T. ) ;
#41009=CARTESIAN_POINT ( 'NONE',  ( 82.94154871197187617, -31.82278776394949205, -23.23890551632149482 ) ) ;
#41011=VECTOR ( 'NONE', #22425, 1000.000000000000000 ) ;
#41013=DIRECTION ( 'NONE',  ( 0.000000000000000000, -0.9284778069183718952, -0.3713878862591650232 ) ) ;
#41014=CARTESIAN_POINT ( 'NONE',  ( 114.7192077545248594, -2.791137627527939813, -18.39754474579286025 ) ) ;
#41016=PLANE ( 'NONE',  #16767 ) ;
#41032=EDGE_CURVE ( 'NONE', #529, #25300, #41340, .T. ) ;
#41033=CARTESIAN_POINT ( 'NONE',  ( 106.6626452545248611, -9.868328341294098749, -15.46607636864997204 ) ) ;
#41043=DIRECTION ( 'NONE',  ( 0.000000000000000000, 0.000000000000000000, -1.000000000000000000 ) ) ;
#41044=CARTESIAN_POINT ( 'NONE',  ( 87.44708369096657918, -29.99489077589588959, -18.39321520033831803 ) ) ;
#41046=EDGE_CURVE ( 'NONE', #21853, #27652, #12904, .T. ) ;
#41050=AXIS2_PLACEMENT_3D ( 'NONE', #37809, #41480, #3598 ) ;
#41061=CARTESIAN_POINT ( 'NONE',  ( 108.1906140045248463, -10.62599879583958717, -11.00651665394454604 ) ) ;
#41062=CARTESIAN_POINT ( 'NONE',  ( 69.69189222814998175, -41.76310523276723785, -20.39321520033831447 ) ) ;
#41063=CARTESIAN_POINT ( 'NONE',  ( 105.3430358795248338, -8.402594152722688392, -9.854619843455216355 ) ) ;
#41070=CARTESIAN_POINT ( 'NONE',  ( 67.69189222814998175, -49.76310523276723785, -34.89321520033831092 ) ) ;
#41073=CARTESIAN_POINT ( 'NONE',  ( 115.8999108795247821, -1.325403438956436419, -16.93181055722141792 ) ) ;
#41094=CARTESIAN_POINT ( 'NONE',  ( 112.1494421295248003, 0.8980012041604618078, -13.39321520033831447 ) ) ;
#41096=ORIENTED_EDGE ( 'NONE', *, *, #32620, .F. ) ;
#41100=CARTESIAN_POINT ( 'NONE',  ( 78.69189222814998175, -60.26310523276723785, -29.64311716074571379 ) ) ;
#41104=LINE ( 'NONE', #9862, #10231 ) ;
#41115=CARTESIAN_POINT ( 'NONE',  ( 109.9269421295247753, 0.8980012041604618078, -13.39321520033831447 ) ) ;
#41116=CARTESIAN_POINT ( 'NONE',  ( 111.5243640045248412, 0.1403307496149616695, -15.46607636864997204 ) ) ;
#41117=CARTESIAN_POINT ( 'NONE',  ( 116.0388171295248014, 0.1403307496149613920, -13.39321520033831447 ) ) ;
#41129=CARTESIAN_POINT ( 'NONE',  ( 115.5526452545247622, -9.868328341294098749, -15.46607636864997204 ) ) ;
#41135=CARTESIAN_POINT ( 'NONE',  ( 106.3848327545248651, -6.936859964151250502, -8.388885654883777576 ) ) ;
#41136=CARTESIAN_POINT ( 'NONE',  ( 112.5661608795247872, -1.325403438956436419, -16.93181055722141792 ) ) ;
#41153=ORIENTED_EDGE ( 'NONE', *, *, #11621, .F. ) ;
#41156=CARTESIAN_POINT ( 'NONE',  ( 115.8304577545247582, -7.250697342233347165, -7.631215200338321125 ) ) ;
#41161=ADVANCED_BREP_SHAPE_REPRESENTATION ( '', ( #6587, #12375 ), #21301 ) ;
#41164=AXIS2_PLACEMENT_3D ( 'NONE', #30034, #19095, #15911 ) ;
#41165=CARTESIAN_POINT ( 'NONE',  ( 116.4597320646196863, 0.6269505268395592079, -14.64321520033831447 ) ) ;
#41171=ORIENTED_EDGE ( 'NONE', *, *, #32554, .F. ) ;
#41174=CARTESIAN_POINT ( 'NONE',  ( 106.5237390045248418, -9.868328341294098749, -11.32035403202665869 ) ) ;
#41178=CARTESIAN_POINT ( 'NONE',  ( 114.2330358795247776, -8.402594152722688392, -9.854619843455216355 ) ) ;
#41179=CARTESIAN_POINT ( 'NONE',  ( 111.9410827545248708, -2.477300249445798297, -19.15521520033830427 ) ) ;
#41182=CARTESIAN_POINT ( 'NONE',  ( 106.4542858795248179, -0.7896495226426338832, -17.46756447353520159 ) ) ;
#41184=LINE ( 'NONE', #10389, #42272 ) ;
#41185=CARTESIAN_POINT ( 'NONE',  ( 114.5108483795247878, -0.7896495226426338832, -9.318865927141430916 ) ) ;
#41199=VERTEX_POINT ( 'NONE', #32944 ) ;
#41204=CARTESIAN_POINT ( 'NONE',  ( 116.8537841442347656, -0.5650535969755431376, -16.42331166093997652 ) ) ;
#41205=CARTESIAN_POINT ( 'NONE',  ( 115.4137390045248566, 0.8980012041604421569, -15.77991374673208469 ) ) ;
#41208=CARTESIAN_POINT ( 'NONE',  ( 112.9810566399283829, 0.4261359969231631739, -14.64321520033830026 ) ) ;
#41209=EDGE_CURVE ( 'NONE', #40056, #27343, #33619, .T. ) ;
#41212=CARTESIAN_POINT ( 'NONE',  ( 117.0960808822395478, 1.608673864571572798, -5.427676334679006231 ) ) ;
#41215=CARTESIAN_POINT ( 'NONE',  ( 105.3430358795248338, -8.402594152722688392, -9.854619843455216355 ) ) ;
#41216=CARTESIAN_POINT ( 'NONE',  ( 111.3598964071292841, 0.2518737723193609224, -14.64321520033828783 ) ) ;
#41231=CARTESIAN_POINT ( 'NONE',  ( 109.3713171295247832, -10.62599879583958540, -13.39321520033831447 ) ) ;
#41232=CARTESIAN_POINT ( 'NONE',  ( 106.5931921295248372, -9.868328341294093420, -13.39321520033831447 ) ) ;
#41233=CARTESIAN_POINT ( 'NONE',  ( 115.7610046295247912, -4.863998795839590272, -7.631215200338315796 ) ) ;
#41236=CARTESIAN_POINT ( 'NONE',  ( 109.2294580127160941, -8.142638662055460941, -8.698686866961791608 ) ) ;
#41237=CARTESIAN_POINT ( 'NONE',  ( 112.7491510812576934, -0.01829820670803256055, -12.14321520033831625 ) ) ;
#41238=CARTESIAN_POINT ( 'NONE',  ( 108.5378796295247810, -4.863998795839590272, -8.388885654883775800 ) ) ;
#41239=ORIENTED_EDGE ( 'NONE', *, *, #20325, .T. ) ;
#41241=FACE_OUTER_BOUND ( 'NONE', #18822, .T. ) ;
#41250=ORIENTED_EDGE ( 'NONE', *, *, #20325, .F. ) ;
#41254=CIRCLE ( 'NONE', #18670, 10.00000000000000178 ) ;
#41260=CARTESIAN_POINT ( 'NONE',  ( 116.3166296295247832, -4.863998795839590272, -19.15521520033831493 ) ) ;
#41262=PLANE ( 'NONE',  #41050 ) ;
#41274=DIRECTION ( 'NONE',  ( -0.07634843047859418697, -0.9970811988817437355, 0.000000000000000000 ) ) ;
#41284=ORIENTED_EDGE ( 'NONE', *, *, #22779, .F. ) ;
#41287=CARTESIAN_POINT ( 'NONE',  ( 106.8710046295248759, -4.863998795839590272, -7.631215200338315796 ) ) ;
#41289=CARTESIAN_POINT ( 'NONE',  ( 105.0652233795248378, -1.325403438956436419, -9.854619843455211026 ) ) ;
#41290=CARTESIAN_POINT ( 'NONE',  ( 105.5513952545248060, -9.868328341294098749, -15.46607636864997204 ) ) ;
#41291=CARTESIAN_POINT ( 'NONE',  ( 64.46535740945334680, -37.09977221485072363, -5.366017974039236194 ) ) ;
#41297=EDGE_CURVE ( 'NONE', #9382, #18860, #33159, .T. ) ;
#41298=VECTOR ( 'NONE', #10910, 1000.000000000000000 ) ;
#41300=CARTESIAN_POINT ( 'NONE',  ( 106.1070202545248407, -10.62599879583958717, -15.77991374673208469 ) ) ;
#41303=DIRECTION ( 'NONE',  ( -1.000000000000000000, 0.000000000000000000, 0.000000000000000000 ) ) ;
#41306=EDGE_CURVE ( 'NONE', #9168, #930, #38278, .T. ) ;
#41309=CARTESIAN_POINT ( 'NONE',  ( 76.69189222814998175, -50.16718729050181480, -6.893215200338315363 ) ) ;
#41314=CARTESIAN_POINT ( 'NONE',  ( 116.5949565311550913, -9.864074739043591222, -13.32529961072451741 ) ) ;
#41315=AXIS2_PLACEMENT_3D ( 'NONE', #7638, #17686, #31584 ) ;
#41318=VERTEX_POINT ( 'NONE', #44370 ) ;
#41322=CARTESIAN_POINT ( 'NONE',  ( 107.2877233795247776, -8.938348069036489818, -17.46756447353520159 ) ) ;
#41329=CARTESIAN_POINT ( 'NONE',  ( 69.69189222814998175, -41.76310523276723785, -6.393215200338315363 ) ) ;
#41331=DIRECTION ( 'NONE',  ( 0.000000000000000000, 0.000000000000000000, 1.000000000000000000 ) ) ;
#41333=DIRECTION ( 'NONE',  ( 1.591814108749227602E-14, -1.000000000000000000, 0.000000000000000000 ) ) ;
#41340=B_SPLINE_CURVE_WITH_KNOTS ( 'NONE', 3,
 ( #19050, #43226, #29760, #39799, #8568, #33611, #40710, #37264, #5366, #44139 ),
 .UNSPECIFIED., .F., .F.,
 ( 4, 3, 3, 4 ),
 ( 0.000000000000000000, 0.0002476487219222709845, 0.0004952974148303440237, 0.0009534114850261750764 ),
 .UNSPECIFIED. ) ;
#41345=CARTESIAN_POINT ( 'NONE',  ( 109.7185827545247889, -2.477300249445798297, -19.15521520033831138 ) ) ;
#41346=CARTESIAN_POINT ( 'NONE',  ( 113.1912390045248031, -9.868328341294098749, -11.32035403202665869 ) ) ;
#41347=CARTESIAN_POINT ( 'NONE',  ( 106.2459265045248173, -7.250697342233347165, -19.15521520033831138 ) ) ;
#41348=AXIS2_PLACEMENT_3D ( 'NONE', #32043, #811, #21342 ) ;
#41353=CARTESIAN_POINT ( 'NONE',  ( 109.8574890045247940, 0.8980012041604421569, -15.77991374673208469 ) ) ;
#41360=CARTESIAN_POINT ( 'NONE',  ( 105.5513952545248060, 0.8980012041604421569, -11.00651665394454071 ) ) ;
#41362=LINE ( 'NONE', #10119, #4824 ) ;
#41366=CARTESIAN_POINT ( 'NONE',  ( 108.7462390045248242, -9.868328341294098749, -11.32035403202665869 ) ) ;
#41367=CARTESIAN_POINT ( 'NONE',  ( 108.5378796295247810, -4.863998795839590272, -8.388885654883775800 ) ) ;
#41372=AXIS2_PLACEMENT_3D ( 'NONE', #29314, #12220, #26119 ) ;
#41377=( BOUNDED_CURVE ( )  B_SPLINE_CURVE ( 2, ( #21980, #32454, #39540, #32677, #14919, #28375, #11723, #32232, #42515, #18563, #11275, #28829, #35649, #1445, #4423, #11505, #1229 ),
 .UNSPECIFIED., .F., .T. ) 
 B_SPLINE_CURVE_WITH_KNOTS ( ( 3, 2, 2, 2, 2, 2, 2, 2, 3 ),
 ( 0.003509120678721945087, 0.01250000000000000069, 0.02500000000000000139, 0.03749999999999999861, 0.04999999999999999584, 0.06250000000000000000, 0.07499999999999999722, 0.08749999999999999445, 0.09649087932127788092 ),
 .UNSPECIFIED. ) 
 CURVE ( )  GEOMETRIC_REPRESENTATION_ITEM ( )  RATIONAL_B_SPLINE_CURVE ( ( 0.9692594319298230010, 0.9452488050343769155, 1.000000000000000000, 0.9238795325112869605, 1.000000000000000000, 0.9238795325112869605, 1.000000000000000000, 0.9238795325112869605, 1.000000000000000000, 0.9238795325112869605, 1.000000000000000000, 0.9238795325112869605, 1.000000000000000000, 0.9238795325112869605, 1.000000000000000000, 0.9452488050343769155, 0.9692594319298220018 ) ) 
 REPRESENTATION_ITEM ( '' )  );
#41386=FACE_OUTER_BOUND ( 'NONE', #28870, .T. ) ;
#41387=CARTESIAN_POINT ( 'NONE',  ( 115.9693640045247776, -10.62599879583958717, -11.00651665394454604 ) ) ;
#41388=CARTESIAN_POINT ( 'NONE',  ( 108.7294421295247844, -9.051693226400931991, -21.89321520033831447 ) ) ;
#41394=CARTESIAN_POINT ( 'NONE',  ( 116.1758551332721936, 0.2334052082820642360, -14.64321520033831447 ) ) ;
#41395=CARTESIAN_POINT ( 'NONE',  ( 113.0523327545247838, -2.477300249445798297, -19.15521520033830427 ) ) ;
#41397=CARTESIAN_POINT ( 'NONE',  ( 66.21962885992722647, -37.11159810974177731, -4.893215200338314474 ) ) ;
#41400=VERTEX_POINT ( 'NONE', #41847 ) ;
#41402=CARTESIAN_POINT ( 'NONE',  ( 107.2294421295247844, -9.051693226400931991, -21.89321520033831447 ) ) ;
#41403=CARTESIAN_POINT ( 'NONE',  ( 115.7610046295247912, -4.863998795839590272, -7.631215200338315796 ) ) ;
#41407=CARTESIAN_POINT ( 'NONE',  ( 108.4684265045248424, -2.791137627527939813, -8.388885654883777576 ) ) ;
#41408=CARTESIAN_POINT ( 'NONE',  ( 112.1114130180079798, 0.7607806665037644134, -14.64321520033833046 ) ) ;
#41409=CARTESIAN_POINT ( 'NONE',  ( 109.2294421295247844, -1.388378309844742642, -16.99368411936019641 ) ) ;
#41412=CARTESIAN_POINT ( 'NONE',  ( 106.3153796295248412, -4.863998795839590272, -19.15521520033831493 ) ) ;
#41414=CARTESIAN_POINT ( 'NONE',  ( 87.44708369096657918, -21.99489077589588604, -4.893215200338314474 ) ) ;
#41415=CARTESIAN_POINT ( 'NONE',  ( 111.4549108795247747, -8.938348069036489818, -9.318865927141430916 ) ) ;
#41418=CARTESIAN_POINT ( 'NONE',  ( 112.0630644685027875, 0.6938714319018670640, -14.64321520033829671 ) ) ;
#41430=CARTESIAN_POINT ( 'NONE',  ( 116.8411265865987332, -0.9886851213817485773, -16.93018519047561554 ) ) ;
#41431=CARTESIAN_POINT ( 'NONE',  ( 115.4831921295247952, 0.8980012041604618078, -13.39321520033831447 ) ) ;
#41437=CARTESIAN_POINT ( 'NONE',  ( 116.8772542192391199, 1.929060082349297822, -5.778250657087603770 ) ) ;
#41439=CARTESIAN_POINT ( 'NONE',  ( 106.8710046295248759, -4.863998795839590272, -18.39754474579285315 ) ) ;
#41443=CARTESIAN_POINT ( 'NONE',  ( 115.5695697905468933, 0.6938714319018670640, -12.14321520033833579 ) ) ;
#41452=CARTESIAN_POINT ( 'NONE',  ( 112.2883483795247770, -0.7896495226426338832, -9.318865927141430916 ) ) ;
#41459=CARTESIAN_POINT ( 'NONE',  ( 107.8433483795247838, -8.402594152722688392, -16.93181055722141792 ) ) ;
#41460=CARTESIAN_POINT ( 'NONE',  ( 109.2294424423713650, -0.4563628856859095473, -15.90327673384510376 ) ) ;
#41473=FACE_OUTER_BOUND ( 'NONE', #7184, .T. ) ;
#41478=CARTESIAN_POINT ( 'NONE',  ( 115.9693640045247776, -10.62599879583958717, -11.00651665394454604 ) ) ;
#41480=DIRECTION ( 'NONE',  ( 0.000000000000000000, 0.000000000000000000, -1.000000000000000000 ) ) ;
#41485=ORIENTED_EDGE ( 'NONE', *, *, #45112, .F. ) ;
#41486=CARTESIAN_POINT ( 'NONE',  ( 114.5803015045248117, -2.477300249445798297, -7.631215200338321125 ) ) ;
#41489=DIRECTION ( 'NONE',  ( 0.4649787261689616868, 0.8853218534579894161, 0.000000000000000000 ) ) ;
#41490=EDGE_CURVE ( 'NONE', #36673, #44158, #18127, .T. ) ;
#41491=CARTESIAN_POINT ( 'NONE',  ( 78.69189222814995333, -59.47240852290178026, 0.2605592176021376827 ) ) ;
#41498=CARTESIAN_POINT ( 'NONE',  ( 72.69189222814998175, -41.76310523276723785, -24.89321520033831447 ) ) ;
#41507=CARTESIAN_POINT ( 'NONE',  ( 109.0935046295247872, -4.863998795839590272, -7.631215200338315796 ) ) ;
#41508=CARTESIAN_POINT ( 'NONE',  ( 107.2877233795247776, -1.325403438956436419, -9.854619843455211026 ) ) ;
#41513=VECTOR ( 'NONE', #13284, 1000.000000000000000 ) ;
#41518=CARTESIAN_POINT ( 'NONE',  ( 115.4137390045248566, -9.868328341294098749, -11.32035403202665869 ) ) ;
#41520=ORIENTED_EDGE ( 'NONE', *, *, #35777, .F. ) ;
#41530=DIRECTION ( 'NONE',  ( 1.000000000000000000, 0.000000000000000000, 0.000000000000000000 ) ) ;
#41538=CARTESIAN_POINT ( 'NONE',  ( 106.8710046295248759, -4.863998795839590272, -7.631215200338315796 ) ) ;
#41546=DIRECTION ( 'NONE',  ( 1.000000000000000000, 0.000000000000000000, 0.000000000000000000 ) ) ;
#41547=EDGE_CURVE ( 'NONE', #22388, #15377, #41946, .T. ) ;
#41548=DIRECTION ( 'NONE',  ( 0.000000000000000000, -0.6998542122237657592, -0.7142857142857138575 ) ) ;
#41561=CARTESIAN_POINT ( 'NONE',  ( 108.8156921295247912, 0.8980012041604618078, -13.39321520033831447 ) ) ;
#41562=CARTESIAN_POINT ( 'NONE',  ( 108.3295202545248657, 0.1403307496149616695, -11.32035403202665336 ) ) ;
#41563=CARTESIAN_POINT ( 'NONE',  ( 108.2600671295247992, -10.62599879583958540, -13.39321520033831447 ) ) ;
#41569=CARTESIAN_POINT ( 'NONE',  ( 109.5796765045248122, -7.250697342233347165, -19.15521520033831138 ) ) ;
#41575=CARTESIAN_POINT ( 'NONE',  ( 107.1488171295247867, -10.62599879583958540, -13.39321520033831447 ) ) ;
#41581=CARTESIAN_POINT ( 'NONE',  ( 115.6915515045247531, -2.477300249445798297, -7.631215200338321125 ) ) ;
#41582=CARTESIAN_POINT ( 'NONE',  ( 106.9404577545248145, -2.791137627527939813, -18.39754474579286025 ) ) ;
#41596=ORIENTED_EDGE ( 'NONE', *, *, #29187, .F. ) ;
#41599=FACE_OUTER_BOUND ( 'NONE', #12142, .T. ) ;
#41604=CARTESIAN_POINT ( 'NONE',  ( 114.2330358795247776, -0.7896495226426338832, -17.46756447353520159 ) ) ;
#41609=VECTOR ( 'NONE', #43095, 1000.000000000000000 ) ;
#41616=CARTESIAN_POINT ( 'NONE',  ( 84.39081516114413262, -30.32262605124143562, -12.39321520033831447 ) ) ;
#41619=ORIENTED_EDGE ( 'NONE', *, *, #10549, .F. ) ;
#41622=CARTESIAN_POINT ( 'NONE',  ( 106.7320983795247855, -8.402594152722688392, -16.93181055722141792 ) ) ;
#41626=FACE_OUTER_BOUND ( 'NONE', #36063, .T. ) ;
#41627=CARTESIAN_POINT ( 'NONE',  ( 110.1353015045248469, -6.936859964151250502, -18.39754474579286025 ) ) ;
#41628=CARTESIAN_POINT ( 'NONE',  ( 111.1282721536728104, 0.3967854368540359999, -10.50530088663808925 ) ) ;
#41632=CARTESIAN_POINT ( 'NONE',  ( 107.9822546295247889, -4.863998795839590272, -7.631215200338315796 ) ) ;
#41634=CARTESIAN_POINT ( 'NONE',  ( 109.2324108795247923, -8.938348069036489818, -9.318865927141430916 ) ) ;
#41643=AXIS2_PLACEMENT_3D ( 'NONE', #43571, #35810, #12340 ) ;
#41650=CARTESIAN_POINT ( 'NONE',  ( 116.8404992881385311, -1.011272923461008499, -16.95395943642953540 ) ) ;
#41651=CARTESIAN_POINT ( 'NONE',  ( 115.8304577545247582, -7.250697342233347165, -7.631215200338321125 ) ) ;
#41654=DIRECTION ( 'NONE',  ( 0.000000000000000000, 0.000000000000000000, 1.000000000000000000 ) ) ;
#41663=LINE ( 'NONE', #24327, #2534 ) ;
#41664=CARTESIAN_POINT ( 'NONE',  ( 114.5803015045248117, -6.936859964151250502, -18.39754474579286025 ) ) ;
#41667=CARTESIAN_POINT ( 'NONE',  ( 115.6179021944298881, 0.6269505268395592079, -12.14321520033831625 ) ) ;
#41670=ORIENTED_EDGE ( 'NONE', *, *, #45135, .T. ) ;
#41676=CARTESIAN_POINT ( 'NONE',  ( 105.2041296295248287, -4.863998795839590272, -8.388885654883775800 ) ) ;
#41677=CARTESIAN_POINT ( 'NONE',  ( 111.1076452545248259, 0.8980012041604421569, -11.00651665394454071 ) ) ;
#41681=CARTESIAN_POINT ( 'NONE',  ( 107.4960827545248350, -6.936859964151250502, -8.388885654883777576 ) ) ;
#41682=CARTESIAN_POINT ( 'NONE',  ( 61.69189222814998175, -69.76310523276724496, -16.89321520033831447 ) ) ;
#41685=DIRECTION ( 'NONE',  ( -1.000000000000000000, 0.000000000000000000, 0.000000000000000000 ) ) ;
#41686=ORIENTED_EDGE ( 'NONE', *, *, #34184, .T. ) ;
#41687=LINE ( 'NONE', #24352, #26115 ) ;
#41694=CARTESIAN_POINT ( 'NONE',  ( 106.3848327545248651, -6.936859964151250502, -8.388885654883777576 ) ) ;
#41703=CARTESIAN_POINT ( 'NONE',  ( 114.9275671295247889, -10.62599879583958540, -13.39321520033831447 ) ) ;
#41705=DIRECTION ( 'NONE',  ( -0.3445294493088569276, -0.9387755102040827859, 0.000000000000000000 ) ) ;
#41708=CARTESIAN_POINT ( 'NONE',  ( 77.38862445244474486, -56.64805777995697156, -1.793693935343831258 ) ) ;
#41713=AXIS2_PLACEMENT_3D ( 'NONE', #25633, #40438, #15812 ) ;
#41721=CARTESIAN_POINT ( 'NONE',  ( 115.9693640045247776, 0.1403307496149616695, -15.46607636864997204 ) ) ;
#41724=CARTESIAN_POINT ( 'NONE',  ( 105.4124890045248293, -9.868328341294098749, -11.32035403202665869 ) ) ;
#41733=CARTESIAN_POINT ( 'NONE',  ( 113.3301452545248083, -9.868328341294098749, -15.46607636864997204 ) ) ;
#41735=ORIENTED_EDGE ( 'NONE', *, *, #13758, .F. ) ;
#41740=CARTESIAN_POINT ( 'NONE',  ( 70.19189222814998175, -66.20485342690169261, -45.06987807991856698 ) ) ;
#41742=DIRECTION ( 'NONE',  ( -1.165517335421915886E-15, -1.000000000000000000, -1.010925141707166031E-30 ) ) ;
#41744=ORIENTED_EDGE ( 'NONE', *, *, #9989, .T. ) ;
#41747=AXIS2_PLACEMENT_3D ( 'NONE', #36356, #5127, #19043 ) ;
#41748=CARTESIAN_POINT ( 'NONE',  ( 116.5952498694597921, -9.864550231015533299, -13.34038451353460886 ) ) ;
#41749=AXIS2_PLACEMENT_3D ( 'NONE', #42953, #35645, #35184 ) ;
#41756=CARTESIAN_POINT ( 'NONE',  ( 106.3153796295248412, -4.863998795839590272, -19.15521520033831493 ) ) ;
#41759=ORIENTED_EDGE ( 'NONE', *, *, #3745, .F. ) ;
#41763=DIRECTION ( 'NONE',  ( -0.9970811988817435134, 0.07634843047859724008, 0.000000000000000000 ) ) ;
#41764=CARTESIAN_POINT ( 'NONE',  ( 87.44708369096657918, -21.99489077589588604, -18.39321520033831803 ) ) ;
#41767=CARTESIAN_POINT ( 'NONE',  ( 63.69189222814998175, -55.76602098829192755, -2.607500914624014232 ) ) ;
#41773=CARTESIAN_POINT ( 'NONE',  ( 69.63874157094764428, -25.41500789246203951, -5.785566283887345840 ) ) ;
#41780=CARTESIAN_POINT ( 'NONE',  ( 107.9822546295247889, -4.863998795839590272, -7.631215200338315796 ) ) ;
#41782=CARTESIAN_POINT ( 'NONE',  ( 106.9404577545248145, -2.791137627527939813, -18.39754474579286025 ) ) ;
#41783=CARTESIAN_POINT ( 'NONE',  ( 115.9693640045247776, 0.1403307496149616695, -15.46607636864997204 ) ) ;
#41786=EDGE_LOOP ( 'NONE', ( #34493, #6446, #40686, #12086, #18530 ) ) ;
#41788=CARTESIAN_POINT ( 'NONE',  ( 110.2047546295247855, -4.863998795839590272, -7.631215200338315796 ) ) ;
#41789=CARTESIAN_POINT ( 'NONE',  ( 73.53114257624162065, -54.10809544429395856, -19.39321520033831447 ) ) ;
#41795=CARTESIAN_POINT ( 'NONE',  ( 113.8163171295247764, -10.62599879583958540, -13.39321520033831447 ) ) ;
#41796=CARTESIAN_POINT ( 'NONE',  ( 106.3848327545248651, -2.477300249445798297, -19.15521520033831138 ) ) ;
#41802=CARTESIAN_POINT ( 'NONE',  ( 114.2330358795247776, -0.7896495226426338832, -17.46756447353520159 ) ) ;
#41803=CARTESIAN_POINT ( 'NONE',  ( 106.1764733795248219, -1.325403438956436419, -9.854619843455211026 ) ) ;
#41809=EDGE_CURVE ( 'NONE', #3847, #10734, #41377, .T. ) ;
#41812=CARTESIAN_POINT ( 'NONE',  ( 78.69189222814998175, -46.76310523276723785, -4.893215200338314474 ) ) ;
#41816=VECTOR ( 'NONE', #5732, 1000.000000000000114 ) ;
#41817=CARTESIAN_POINT ( 'NONE',  ( 111.1770983795247787, -8.402594152722688392, -16.93181055722141792 ) ) ;
#41818=VERTEX_POINT ( 'NONE', #37219 ) ;
#41823=CARTESIAN_POINT ( 'NONE',  ( 90.67797751089673852, -17.83979763915464289, -20.89321520033831447 ) ) ;
#41825=CARTESIAN_POINT ( 'NONE',  ( 106.9404577545248145, -2.791137627527939813, -18.39754474579286025 ) ) ;
#41831=CARTESIAN_POINT ( 'NONE',  ( 116.6766162288780890, -8.450459793919360862, -16.99402653318119505 ) ) ;
#41834=CARTESIAN_POINT ( 'NONE',  ( 85.19105201044544629, -29.19355814263353821, -9.935028317583610047 ) ) ;
#41835=CARTESIAN_POINT ( 'NONE',  ( 116.2659068881580708, -12.01880880694303855, -4.893215200338314474 ) ) ;
#41840=CARTESIAN_POINT ( 'NONE',  ( 110.1353015045248469, -2.477300249445798297, -7.631215200338321125 ) ) ;
#41846=CARTESIAN_POINT ( 'NONE',  ( 108.8156921295247912, -9.868328341294093420, -13.39321520033831447 ) ) ;
#41847=CARTESIAN_POINT ( 'NONE',  ( 111.0001630180080809, 0.7607806665038616689, -14.64321520033831447 ) ) ;
#41848=CARTESIAN_POINT ( 'NONE',  ( 109.2294481158511275, -7.112626342048868899, -18.18810309623751564 ) ) ;
#41851=CARTESIAN_POINT ( 'NONE',  ( 117.0111608795247946, -1.325403438956436419, -16.93181055722141792 ) ) ;
#41852=CARTESIAN_POINT ( 'NONE',  ( 107.9822546295247889, -4.863998795839590272, -7.631215200338315796 ) ) ;
#41869=CARTESIAN_POINT ( 'NONE',  ( 113.0523327545247838, -2.477300249445798297, -19.15521520033831138 ) ) ;
#41870=CARTESIAN_POINT ( 'NONE',  ( 61.76986277844709861, -39.32091226840162079, -4.893215200338314474 ) ) ;
#41878=CARTESIAN_POINT ( 'NONE',  ( 113.8163171295247764, 0.1403307496149613920, -13.39321520033831447 ) ) ;
#41883=FACE_OUTER_BOUND ( 'NONE', #24920, .T. ) ;
#41892=CARTESIAN_POINT ( 'NONE',  ( 106.7320983795247855, -8.402594152722688392, -16.93181055722141792 ) ) ;
#41893=CARTESIAN_POINT ( 'NONE',  ( 110.7603796295247918, -4.863998795839590272, -19.15521520033831493 ) ) ;
#41897=CARTESIAN_POINT ( 'NONE',  ( 109.2294421295247844, 0.2400687412228638684, -12.14321520033831625 ) ) ;
#41899=CARTESIAN_POINT ( 'NONE',  ( 106.9404577545248145, -2.791137627527939813, -18.39754474579286025 ) ) ;
#41900=CARTESIAN_POINT ( 'NONE',  ( 117.1221491469711964, 1.552509864743009782, -21.40721312732405934 ) ) ;
#41903=CARTESIAN_POINT ( 'NONE',  ( 112.7745202545247878, -10.62599879583958717, -15.77991374673208469 ) ) ;
#41915=CARTESIAN_POINT ( 'NONE',  ( 107.7738952545248310, -9.868328341294098749, -15.46607636864997204 ) ) ;
#41923=CARTESIAN_POINT ( 'NONE',  ( 106.3848327545248651, -6.936859964151250502, -8.388885654883777576 ) ) ;
#41928=CARTESIAN_POINT ( 'NONE',  ( 77.01163399656647357, -56.15206630274370525, -2.229255299424385939 ) ) ;
#41930=DIRECTION ( 'NONE',  ( -0.9970811988817434024, 0.07634843047859753151, 0.000000000000000000 ) ) ;
#41933=AXIS2_PLACEMENT_3D ( 'NONE', #899, #4543, #24852 ) ;
#41940=ORIENTED_EDGE ( 'NONE', *, *, #14761, .F. ) ;
#41942=CARTESIAN_POINT ( 'NONE',  ( 109.3713171295247832, -10.62599879583958540, -13.39321520033831447 ) ) ;
#41945=CARTESIAN_POINT ( 'NONE',  ( 113.7698838361194760, 0.1075849324168598464, -12.14321520033829849 ) ) ;
#41946=CIRCLE ( 'NONE', #9205, 5.635000000000000675 ) ;
#41951=CARTESIAN_POINT ( 'NONE',  ( 85.75809888461174069, -18.45227461768569199, -4.893215200338314474 ) ) ;
#41954=CARTESIAN_POINT ( 'NONE',  ( 111.4549108795247747, -1.325403438956436419, -16.93181055722141792 ) ) ;
#41956=ORIENTED_EDGE ( 'NONE', *, *, #30873, .F. ) ;
#41973=PRODUCT_DEFINITION_SHAPE ( 'NONE', 'NONE',  #33583 ) ;
#41976=CARTESIAN_POINT ( 'NONE',  ( 107.5655358795247736, -0.7896495226426338832, -17.46756447353520159 ) ) ;
#41996=CIRCLE ( 'NONE', #10684, 20.00000000000000355 ) ;
#41998=CARTESIAN_POINT ( 'NONE',  ( 114.1635827545248389, -6.936859964151250502, -8.388885654883777576 ) ) ;
#41999=CARTESIAN_POINT ( 'NONE',  ( 107.6349890045248401, -9.868328341294098749, -11.32035403202665869 ) ) ;
#42000=CARTESIAN_POINT ( 'NONE',  ( 113.3995983795247895, -8.402594152722688392, -16.93181055722141792 ) ) ;
#42005=CARTESIAN_POINT ( 'NONE',  ( 109.7185827545247889, -2.477300249445798297, -19.15521520033831138 ) ) ;
#42006=DIRECTION ( 'NONE',  ( -1.000000000000000000, -1.671245155169139691E-16, 0.000000000000000000 ) ) ;
#42011=CARTESIAN_POINT ( 'NONE',  ( 105.6208483795248299, -0.7896495226426338832, -9.318865927141430916 ) ) ;
#42016=CARTESIAN_POINT ( 'NONE',  ( 115.4831921295247952, 0.8980012041604618078, -13.39321520033831447 ) ) ;
#42017=CARTESIAN_POINT ( 'NONE',  ( 107.8433483795247838, -8.402594152722688392, -16.93181055722141792 ) ) ;
#42023=ADVANCED_FACE ( 'NONE', ( #36319 ), #5089, .F. ) ;
#42028=ORIENTED_EDGE ( 'NONE', *, *, #31744, .F. ) ;
#42033=ADVANCED_FACE ( 'NONE', ( #29493 ), #3377, .T. ) ;
#42034=CARTESIAN_POINT ( 'NONE',  ( 109.2324108795247923, -1.325403438956436419, -16.93181055722141792 ) ) ;
#42043=CARTESIAN_POINT ( 'NONE',  ( 114.7886608795247696, -8.938348069036489818, -9.318865927141430916 ) ) ;
#42055=CARTESIAN_POINT ( 'NONE',  ( 84.70844274511026128, -29.45715287386303061, -10.31656915580773948 ) ) ;
#42060=DIRECTION ( 'NONE',  ( 0.000000000000000000, 1.000000000000000000, 0.000000000000000000 ) ) ;
#42061=CARTESIAN_POINT ( 'NONE',  ( 109.8574890045247940, 0.8980012041604421569, -15.77991374673208469 ) ) ;
#42067=CARTESIAN_POINT ( 'NONE',  ( 108.1211608795247798, -1.325403438956436419, -16.93181055722141792 ) ) ;
#42070=CARTESIAN_POINT ( 'NONE',  ( 109.2294421270962914, -8.142351692595484636, -17.62070062977968021 ) ) ;
#42072=CARTESIAN_POINT ( 'NONE',  ( 107.3571765045248299, -7.250697342233347165, -19.15521520033831138 ) ) ;
#42074=CARTESIAN_POINT ( 'NONE',  ( 109.0935046295247872, -4.863998795839590272, -7.631215200338315796 ) ) ;
#42077=DIRECTION ( 'NONE',  ( 0.000000000000000000, 0.000000000000000000, -1.000000000000000000 ) ) ;
#42085=ORIENTED_EDGE ( 'NONE', *, *, #22951, .F. ) ;
#42087=EDGE_CURVE ( 'NONE', #4906, #14703, #41254, .T. ) ;
#42090=CARTESIAN_POINT ( 'NONE',  ( 108.1211608795247798, -8.938348069036489818, -9.318865927141430916 ) ) ;
#42093=LINE ( 'NONE', #10632, #13160 ) ;
#42097=CARTESIAN_POINT ( 'NONE',  ( 111.0762212410415799, 0.7607806665037644134, -12.14321520033829316 ) ) ;
#42100=CARTESIAN_POINT ( 'NONE',  ( 113.6774108795247997, -1.325403438956436419, -16.93181055722141792 ) ) ;
#42114=CARTESIAN_POINT ( 'NONE',  ( 115.6915515045247531, -6.936859964151250502, -18.39754474579286025 ) ) ;
#42117=CARTESIAN_POINT ( 'NONE',  ( 85.96066202508467313, -27.32956148653828876, -8.622328686912057449 ) ) ;
#42118=CARTESIAN_POINT ( 'NONE',  ( 112.3578015045248861, -2.477300249445798297, -7.631215200338321125 ) ) ;
#42122=CARTESIAN_POINT ( 'NONE',  ( 109.2294439528113230, -3.574589291641149025, -8.025114565246834530 ) ) ;
#42124=CARTESIAN_POINT ( 'NONE',  ( 110.0658483795247804, -8.402594152722688392, -16.93181055722141792 ) ) ;
#42128=CARTESIAN_POINT ( 'NONE',  ( 111.3854577545248645, -7.250697342233347165, -7.631215200338321125 ) ) ;
#42130=ORIENTED_EDGE ( 'NONE', *, *, #13644, .T. ) ;
#42138=CARTESIAN_POINT ( 'NONE',  ( 114.3719421295247827, 0.8980012041604618078, -13.39321520033831447 ) ) ;
#42148=CARTESIAN_POINT ( 'NONE',  ( 116.3166296295247832, -4.863998795839590272, -19.15521520033831493 ) ) ;
#42153=( BOUNDED_SURFACE ( )  B_SPLINE_SURFACE ( 3, 2, ( 
 ( #5148, #11782, #15877 ),
 ( #18402, #11331, #29774 ),
 ( #32511, #40036, #32730 ),
 ( #25689, #4481, #39140 ),
 ( #22706, #43013, #8357 ),
 ( #19065, #22261, #42799 ),
 ( #15198, #32949, #1059 ),
 ( #39596, #22483, #32294 ),
 ( #1286, #1726, #12009 ),
 ( #14974, #8138, #4924 ),
 ( #18838, #15648, #1504 ),
 ( #29552, #11560, #22039 ),
 ( #15424, #25911, #25242 ),
 ( #5379, #7905, #26132 ) ),
 .UNSPECIFIED., .F., .F., .F. ) 
 B_SPLINE_SURFACE_WITH_KNOTS ( ( 4, 2, 2, 2, 2, 2, 4 ),
 ( 3, 3 ),
 ( 2.482289681851995056, 3.039814506485170043, 3.318576918801754871, 3.597339331118345029, 3.876101743434930302, 4.154864155751514687, 4.712388980384689674 ),
 ( 0.000000000000000000, 1.000000000000000000 ),
 .UNSPECIFIED. ) 
 GEOMETRIC_REPRESENTATION_ITEM ( )  RATIONAL_B_SPLINE_SURFACE ( (
 ( 1.000000000000000000, 0.6031903678053659457, 1.000000000000000000),
 ( 1.000000000000000000, 0.5868400859402069791, 1.000000000000000000),
 ( 1.000000000000000000, 0.5760967621943400285, 1.000000000000000000),
 ( 1.000000000000000000, 0.5718412329145610151, 1.000000000000000000),
 ( 1.000000000000000000, 0.5723757457118600067, 1.000000000000000000),
 ( 1.000000000000000000, 0.5772784653944200706, 1.000000000000000000),
 ( 1.000000000000000000, 0.5816430333813810138, 1.000000000000000000),
 ( 1.000000000000000000, 0.5936320506908580041, 1.000000000000000000),
 ( 1.000000000000000000, 0.6012496247163490182, 1.000000000000000000),
 ( 1.000000000000000000, 0.6188356767525979851, 1.000000000000000000),
 ( 1.000000000000000000, 0.6287978291299359812, 1.000000000000000000),
 ( 1.000000000000000000, 0.6606618940965899300, 1.000000000000000000),
 ( 1.000000000000000000, 0.6844987252709670011, 1.000000000000000000),
 ( 1.000000000000000000, 0.7071067811865470176, 1.000000000000000000) ) ) 
 REPRESENTATION_ITEM ( '' )  SURFACE ( )  );
#42165=CARTESIAN_POINT ( 'NONE',  ( 113.6774108795247997, -1.325403438956436419, -16.93181055722141792 ) ) ;
#42176=DIRECTION ( 'NONE',  ( 0.000000000000000000, 1.000000000000000000, 0.000000000000000000 ) ) ;
#42177=CARTESIAN_POINT ( 'NONE',  ( 110.1353015045248469, -6.936859964151250502, -18.39754474579286025 ) ) ;
#42185=CARTESIAN_POINT ( 'NONE',  ( 0.000000000000000000, 0.000000000000000000, 0.000000000000000000 ) ) ;
#42189=CARTESIAN_POINT ( 'NONE',  ( 110.5266510812576826, -0.01829820670803256055, -12.14321520033831625 ) ) ;
#42198=CARTESIAN_POINT ( 'NONE',  ( 107.9822546295247889, -4.863998795839590272, -7.631215200338315796 ) ) ;
#42203=CARTESIAN_POINT ( 'NONE',  ( 66.82415148905926117, -40.21211973637273474, -4.893215200338314474 ) ) ;
#42208=DIRECTION ( 'NONE',  ( 0.000000000000000000, 0.000000000000000000, 1.000000000000000000 ) ) ;
#42220=CARTESIAN_POINT ( 'NONE',  ( 114.5108483795247878, -8.402594152722688392, -16.93181055722141792 ) ) ;
#42221=CARTESIAN_POINT ( 'NONE',  ( 107.2877233795247776, -1.325403438956436419, -9.854619843455211026 ) ) ;
#42222=CARTESIAN_POINT ( 'NONE',  ( 115.6220983795247861, -8.402594152722688392, -16.93181055722141792 ) ) ;
#42227=CARTESIAN_POINT ( 'NONE',  ( 111.4549108795247747, -8.938348069036489818, -9.318865927141430916 ) ) ;
#42231=CARTESIAN_POINT ( 'NONE',  ( 79.23106798748115409, 4.957210186511446182, -6.038458229677214462 ) ) ;
#42233=CARTESIAN_POINT ( 'NONE',  ( 114.7886608795247696, -8.938348069036489818, -9.318865927141430916 ) ) ;
#42234=CARTESIAN_POINT ( 'NONE',  ( 111.5938171295247940, 0.1403307496149613920, -13.39321520033831447 ) ) ;
#42240=CARTESIAN_POINT ( 'NONE',  ( 107.3571765045248299, -2.791137627527939813, -8.388885654883777576 ) ) ;
#42250=VECTOR ( 'NONE', #22409, 1000.000000000000000 ) ;
#42253=CARTESIAN_POINT ( 'NONE',  ( 108.6073327545248048, -6.936859964151250502, -8.388885654883777576 ) ) ;
#42262=CARTESIAN_POINT ( 'NONE',  ( 92.26512299712632625, -23.76310523276723785, -20.89321520033831447 ) ) ;
#42263=CARTESIAN_POINT ( 'NONE',  ( 109.2324108795247923, -8.938348069036489818, -9.318865927141430916 ) ) ;
#42269=VERTEX_POINT ( 'NONE', #38345 ) ;
#42272=VECTOR ( 'NONE', #31122, 1000.000000000000000 ) ;
#42274=CARTESIAN_POINT ( 'NONE',  ( 115.7610046295247912, -4.863998795839590272, -7.631215200338315796 ) ) ;
#42280=CARTESIAN_POINT ( 'NONE',  ( 111.9410827545248708, -2.477300249445798297, -19.15521520033831138 ) ) ;
#42284=ADVANCED_FACE ( 'NONE', ( #16956 ), #27664, .T. ) ;
#42286=CARTESIAN_POINT ( 'NONE',  ( 109.1629577545248395, -2.791137627527939813, -18.39754474579286025 ) ) ;
#42289=CARTESIAN_POINT ( 'NONE',  ( 109.2294421421874375, -4.292925824281061509, -18.52829067132285346 ) ) ;
#42292=CARTESIAN_POINT ( 'NONE',  ( 115.2053796295247849, -4.863998795839590272, -8.388885654883775800 ) ) ;
#42293=CARTESIAN_POINT ( 'NONE',  ( 108.8156921295247912, 0.8980012041604618078, -13.39321520033831447 ) ) ;
#42308=VECTOR ( 'NONE', #30494, 1000.000000000000000 ) ;
#42311=CARTESIAN_POINT ( 'NONE',  ( 107.7044421295247929, 0.8980012041604618078, -13.39321520033831447 ) ) ;
#42320=CARTESIAN_POINT ( 'NONE',  ( 112.4773541094426719, 0.3591747506842615789, -12.14321520033833046 ) ) ;
#42321=CARTESIAN_POINT ( 'NONE',  ( 114.6497546295247929, -4.863998795839590272, -18.39754474579285315 ) ) ;
#42335=CARTESIAN_POINT ( 'NONE',  ( 115.6220983795247861, -8.402594152722688392, -16.93181055722141792 ) ) ;
#42337=EDGE_CURVE ( 'NONE', #11942, #14735, #41362, .T. ) ;
#42340=CARTESIAN_POINT ( 'NONE',  ( 85.54408422177358773, -28.33925901115217982, -9.149378981526259835 ) ) ;
#42341=CARTESIAN_POINT ( 'NONE',  ( 114.6497546295247929, -4.863998795839590272, -7.631215200338315796 ) ) ;
#42343=CIRCLE ( 'NONE', #23431, 1.000000000000000888 ) ;
#42345=CARTESIAN_POINT ( 'NONE',  ( 116.3166296295247832, -4.863998795839541422, -8.388885654883775800 ) ) ;
#42346=CARTESIAN_POINT ( 'NONE',  ( 109.2295678159355390, -5.842956214023153017, -7.856223403944330386 ) ) ;
#42348=CARTESIAN_POINT ( 'NONE',  ( 113.6079577545248043, -7.250697342233347165, -7.631215200338321125 ) ) ;
#42349=CARTESIAN_POINT ( 'NONE',  ( 116.8168314703984976, 1.985137923759451306, -20.92218200132013806 ) ) ;
#42352=CARTESIAN_POINT ( 'NONE',  ( 112.7050671295247923, -10.62599879583958540, -13.39321520033831447 ) ) ;
#42361=ADVANCED_FACE ( 'NONE', ( #6905 ), #20815, .T. ) ;
#42362=CARTESIAN_POINT ( 'NONE',  ( 112.3578015045248861, -2.477300249445798297, -7.631215200338321125 ) ) ;
#42371=CARTESIAN_POINT ( 'NONE',  ( 116.3860827545247787, -2.477300249445798297, -19.15521520033831138 ) ) ;
#42375=CARTESIAN_POINT ( 'NONE',  ( 64.98167240748409768, -37.86052959031123777, -4.893215200338314474 ) ) ;
#42377=FACE_OUTER_BOUND ( 'NONE', #5900, .T. ) ;
#42388=CARTESIAN_POINT ( 'NONE',  ( 114.1635827545248389, -6.936859964151250502, -8.388885654883777576 ) ) ;
#42390=CARTESIAN_POINT ( 'NONE',  ( 114.5108483795247878, -8.402594152722633325, -16.93181055722144990 ) ) ;
#42391=CIRCLE ( 'NONE', #8894, 3.000000000000002665 ) ;
#42401=CARTESIAN_POINT ( 'NONE',  ( 112.7745202545247878, 0.1403307496149616695, -11.32035403202665336 ) ) ;
#42402=EDGE_LOOP ( 'NONE', ( #21209, #34815, #26657, #12556, #2247 ) ) ;
#42409=CARTESIAN_POINT ( 'NONE',  ( 68.68839935636917460, -25.95913848132418522, -5.893215200338315363 ) ) ;
#42413=CARTESIAN_POINT ( 'NONE',  ( 110.1582811052981867, 0.4930828106259610433, -12.14321520033828428 ) ) ;
#42416=CARTESIAN_POINT ( 'NONE',  ( 115.2053796295247849, -4.863998795839590272, -8.388885654883775800 ) ) ;
#42419=ORIENTED_EDGE ( 'NONE', *, *, #19468, .F. ) ;
#42424=CARTESIAN_POINT ( 'NONE',  ( 111.3854577545248503, -2.791137627527887410, -18.39754474579284249 ) ) ;
#42430=CARTESIAN_POINT ( 'NONE',  ( 79.40221886803639961, 5.047344816279970559, -20.48083050651887405 ) ) ;
#42443=CARTESIAN_POINT ( 'NONE',  ( 113.1706121053768186, 0.3967854368540359999, -16.28112951403850772 ) ) ;
#42444=CARTESIAN_POINT ( 'NONE',  ( 114.7886608795247696, -8.938348069036489818, -9.318865927141430916 ) ) ;
#42445=CARTESIAN_POINT ( 'NONE',  ( 114.5803015045248117, -6.936859964151250502, -18.39754474579286025 ) ) ;
#42446=CARTESIAN_POINT ( 'NONE',  ( 114.6497546295247929, -4.863998795839590272, -18.39754474579285315 ) ) ;
#42449=ORIENTED_EDGE ( 'NONE', *, *, #23940, .F. ) ;
#42451=CARTESIAN_POINT ( 'NONE',  ( 107.3571765045248299, -7.250697342233347165, -19.15521520033831138 ) ) ;
#42458=CARTESIAN_POINT ( 'NONE',  ( 113.5385046295247804, -4.863998795839590272, -7.631215200338315796 ) ) ;
#42459=CARTESIAN_POINT ( 'NONE',  ( 111.8716296295247901, -4.863998795839590272, -8.388885654883775800 ) ) ;
#42470=VERTEX_POINT ( 'NONE', #4140 ) ;
#42472=AXIS2_PLACEMENT_3D ( 'NONE', #39104, #42978, #11527 ) ;
#42479=CARTESIAN_POINT ( 'NONE',  ( 107.0793640045248196, 0.1403307496149616695, -15.46607636864997204 ) ) ;
#42491=CARTESIAN_POINT ( 'NONE',  ( 112.9134265045247645, -7.250697342233347165, -19.15521520033831138 ) ) ;
#42502=CARTESIAN_POINT ( 'NONE',  ( 64.85649322025210495, -35.54674243456235416, -5.785566283887345840 ) ) ;
#42503=CARTESIAN_POINT ( 'NONE',  ( 69.37572422742091760, -11.86958442233774313, -21.89321520033831447 ) ) ;
#42508=CARTESIAN_POINT ( 'NONE',  ( 110.4131140045248287, -10.62599879583958717, -11.00651665394454604 ) ) ;
#42513=CARTESIAN_POINT ( 'NONE',  ( 106.4542858795248179, -8.402594152722688392, -9.854619843455216355 ) ) ;
#42515=CARTESIAN_POINT ( 'NONE',  ( 116.0388171295248014, -10.62599879583958540, -13.39321520033831447 ) ) ;
#42516=CARTESIAN_POINT ( 'NONE',  ( 109.2294425275515266, -7.200841873015452421, -18.15047811013180024 ) ) ;
#42519=CARTESIAN_POINT ( 'NONE',  ( 116.0388171295248014, 0.1403307496149613920, -13.39321520033831447 ) ) ;
#42520=CARTESIAN_POINT ( 'NONE',  ( 114.6497546295247929, -4.863998795839590272, -18.39754474579285315 ) ) ;
#42526=VERTEX_POINT ( 'NONE', #14191 ) ;
#42536=CARTESIAN_POINT ( 'NONE',  ( 108.8851452545248151, 0.8980012041604421569, -11.00651665394454071 ) ) ;
#42537=CYLINDRICAL_SURFACE ( 'NONE', #32966, 0.9999999999999990008 ) ;
#42539=CARTESIAN_POINT ( 'NONE',  ( 112.3578015045248861, -6.936859964151250502, -18.39754474579286025 ) ) ;
#42544=CARTESIAN_POINT ( 'NONE',  ( 112.5680291257774854, 0.2334052082820642360, -12.14321520033833046 ) ) ;
#42545=CARTESIAN_POINT ( 'NONE',  ( 110.4825671295247815, 0.1403307496149613920, -13.39321520033831447 ) ) ;
#42548=LINE ( 'NONE', #28865, #34055 ) ;
#42553=ORIENTED_EDGE ( 'NONE', *, *, #1337, .F. ) ;
#42556=CARTESIAN_POINT ( 'NONE',  ( 114.0941296295247867, -4.863998795839590272, -8.388885654883775800 ) ) ;
#42560=CARTESIAN_POINT ( 'NONE',  ( 84.99660211880991767, -29.66455880986359261, -10.80014759642894084 ) ) ;
#42561=CARTESIAN_POINT ( 'NONE',  ( 114.1635827545248389, -2.477300249445798297, -19.15521520033831138 ) ) ;
#42565=CARTESIAN_POINT ( 'NONE',  ( 109.2294432708102221, -4.940976372564280794, -7.813933925037506611 ) ) ;
#42567=CARTESIAN_POINT ( 'NONE',  ( 115.0664733795247798, -8.938348069036489818, -17.46756447353520159 ) ) ;
#42568=CARTESIAN_POINT ( 'NONE',  ( 117.1097356970102084, 1.580032931476776481, -21.38384006208493915 ) ) ;
#42571=CARTESIAN_POINT ( 'NONE',  ( 112.2883483795247770, -0.7896495226426338832, -9.318865927141430916 ) ) ;
#42573=ORIENTED_EDGE ( 'NONE', *, *, #35034, .F. ) ;
#42575=B_SPLINE_CURVE_WITH_KNOTS ( 'NONE', 3,
 ( #41409, #40954, #9709, #30901, #23621, #20202, #18339, #11050, #770, #14244, #14692, #24954, #110, #25184, #331, #7852, #35419, #3742, #39083, #3967, #20866, #17443, #31562, #14468, #21079, #42289, #31786, #3525, #10386, #4424, #21758, #28160, #35650, #10608, #24295, #35190, #28830, #31336, #32233, #4195, #38849, #21531, #14920, #28376, #17666, #34744, #41848, #1004, #42516, #38182, #7618, #18113, #32006, #11276, #6959, #17888, #14024, #28607, #558, #24511, #27938, #42070, #38396, #7168, #34956, #10828, #24725, #38613, #7389, #21307, #4642, #8744, #12403, #15368, #19237, #15817, #16042, #19006, #29716, #25850, #5539, #36099, #43629, #22204, #18564, #33120, #22651, #39541, #1668, #1888, #25636, #26303, #40210, #1230, #11952, #8526, #22428, #4871, #5321, #29049, #2113, #36547, #8977, #22875, #11506, #32892, #36769, #11724, #19457, #39756, #32678, #33340, #36320, #32455, #15591, #26076, #25410, #42741, #5090, #29494, #43407, #12175, #39310, #42957, #8080, #21981, #35871, #15143, #29272, #8302, #18788 ),
 .UNSPECIFIED., .F., .F.,
 ( 4, 2, 2, 2, 1, 1, 1, 2, 2, 2, 2, 1, 1, 1, 2, 2, 2, 2, 1, 1, 1, 1, 2, 2, 2, 2, 2, 2, 1, 1, 1, 2, 2, 2, 2, 1, 1, 2, 2, 2, 2, 1, 1, 1, 1, 2, 2, 2, 2, 2, 2, 1, 1, 1, 2, 2, 2, 2, 1, 1, 2, 2, 2, 2, 1, 1, 1, 1, 2, 2, 2, 2, 2, 2, 1, 1, 1, 2, 2, 2, 4 ),
 ( 0.000000000000000000, 0.06249999999995042854, 0.09374999999992583710, 0.1093749999999135691, 0.1171874999999075323, 0.1210937499999046457, 0.1230468749999032024, 0.1240234374999024808, 0.1249999999999017453, 0.1562499999998799571, 0.1718749999998689937, 0.1796874999998634981, 0.1835937499998608613, 0.1855468749998595290, 0.1865234374998589462, 0.1874999999998583633, 0.2187499999998322175, 0.2343749999998191169, 0.2421874999998125666, 0.2460937499998093192, 0.2480468749998077649, 0.2490234374998069877, 0.2495117187498066547, 0.2499999999998063216, 0.3124999999997608024, 0.3437499999997379319, 0.3593749999997266076, 0.3671874999997210010, 0.3710937499997181144, 0.3730468749997166711, 0.3740234374997159494, 0.3745117187497156164, 0.3749999999997152833, 0.4062499999997020161, 0.4218749999996954103, 0.4296874999996921352, 0.4335937499996906919, 0.4355468749996899702, 0.4374999999996892486, 0.4687499999996765365, 0.4843749999996702083, 0.4921874999996670441, 0.4960937499996653233, 0.4980468749996646016, 0.4990234374996641575, 0.4995117187496638245, 0.4999999999996634914, 0.5624999999997134514, 0.5937499999997383204, 0.6093749999997509770, 0.6171874999997574163, 0.6210937499997605249, 0.6230468749997619682, 0.6240234374997627453, 0.6245117187497630784, 0.6249999999997635225, 0.6562499999997883915, 0.6718749999998008260, 0.6796874999998070432, 0.6835937499998102629, 0.6855468749998119282, 0.6874999999998135936, 0.7187499999998397948, 0.7343749999998528954, 0.7421874999998594458, 0.7460937499998626654, 0.7480468749998644418, 0.7490234374998653299, 0.7495117187498657740, 0.7499999999998663291, 0.8124999999998983036, 0.8437499999999145128, 0.8593749999999226175, 0.8671874999999266143, 0.8710937499999286127, 0.8730468749999297229, 0.8740234374999301670, 0.8745117187499302780, 0.8749999999999305000, 0.9374999999999651390, 1.000000000000000000 ),
 .UNSPECIFIED. ) ;
#42582=ADVANCED_FACE ( 'NONE', ( #7337 ), #35135, .T. ) ;
#42583=CARTESIAN_POINT ( 'NONE',  ( 113.9552233795247815, -8.938348069036489818, -17.46756447353520159 ) ) ;
#42590=EDGE_CURVE ( 'NONE', #816, #12848, #11226, .T. ) ;
#42592=ORIENTED_EDGE ( 'NONE', *, *, #7822, .T. ) ;
#42593=CARTESIAN_POINT ( 'NONE',  ( 55.39394582045726168, -26.25884925591183716, -7.393215200338315363 ) ) ;
#42595=LINE ( 'NONE', #11357, #41298 ) ;
#42597=CARTESIAN_POINT ( 'NONE',  ( 77.39830673346236267, -56.66119886563520680, -1.782287558316724141 ) ) ;
#42598=CARTESIAN_POINT ( 'NONE',  ( 64.22513517183551812, -35.03390339818633947, -5.893215200338315363 ) ) ;
#42605=EDGE_CURVE ( 'NONE', #41400, #27136, #16778, .T. ) ;
#42610=ADVANCED_FACE ( 'NONE', ( #30123 ), #23279, .F. ) ;
#42615=CARTESIAN_POINT ( 'NONE',  ( 113.5385046295247804, -4.863998795839590272, -18.39754474579285315 ) ) ;
#42626=CARTESIAN_POINT ( 'NONE',  ( 111.9410827545248708, -6.936859964151250502, -8.388885654883777576 ) ) ;
#42638=CARTESIAN_POINT ( 'NONE',  ( 116.4555358795247884, -8.402594152722688392, -9.854619843455216355 ) ) ;
#42649=FACE_OUTER_BOUND ( 'NONE', #10839, .T. ) ;
#42651=FACE_OUTER_BOUND ( 'NONE', #28812, .T. ) ;
#42663=EDGE_LOOP ( 'NONE', ( #43852, #14457, #25598, #31711 ) ) ;
#42667=LINE ( 'NONE', #22137, #5276 ) ;
#42668=CARTESIAN_POINT ( 'NONE',  ( 112.9828796295247884, -4.863998795839590272, -8.388885654883775800 ) ) ;
#42669=CARTESIAN_POINT ( 'NONE',  ( 111.8716296295247901, -4.863998795839590272, -8.388885654883775800 ) ) ;
#42674=CARTESIAN_POINT ( 'NONE',  ( 105.4819421295248247, 0.8980012041604618078, -13.39321520033831447 ) ) ;
#42676=EDGE_CURVE ( 'NONE', #29882, #13861, #15309, .T. ) ;
#42682=CARTESIAN_POINT ( 'NONE',  ( 115.4831921295247952, 0.8980012041604618078, -13.39321520033831447 ) ) ;
#42683=CARTESIAN_POINT ( 'NONE',  ( 109.5102233795247884, -1.325403438956436419, -9.854619843455211026 ) ) ;
#42684=VERTEX_POINT ( 'NONE', #5266 ) ;
#42688=AXIS2_PLACEMENT_3D ( 'NONE', #21055, #306, #10803 ) ;
#42699=CARTESIAN_POINT ( 'NONE',  ( 117.2294421295247844, -4.863998795839590272, -13.39321520033831447 ) ) ;
#42701=CARTESIAN_POINT ( 'NONE',  ( 114.8581140045248361, -10.62599879583958717, -11.00651665394454604 ) ) ;
#42715=CARTESIAN_POINT ( 'NONE',  ( 112.1494421295248003, 0.8980012041604618078, -13.39321520033831447 ) ) ;
#42721=EDGE_LOOP ( 'NONE', ( #13033, #1631, #2793, #27627, #41735, #29084 ) ) ;
#42732=CARTESIAN_POINT ( 'NONE',  ( 112.2188952545247531, 0.8980012041604421569, -11.00651665394454071 ) ) ;
#42737=CARTESIAN_POINT ( 'NONE',  ( 106.8710046295248759, -4.863998795839590272, -18.39754474579285315 ) ) ;
#42739=VERTEX_POINT ( 'NONE', #36938 ) ;
#42741=CARTESIAN_POINT ( 'NONE',  ( 109.2294694551411141, -10.13459952827899357, -11.33384148904508493 ) ) ;
#42744=CARTESIAN_POINT ( 'NONE',  ( 114.7192077545248594, -2.791137627527939813, -18.39754474579286025 ) ) ;
#42745=CARTESIAN_POINT ( 'NONE',  ( 113.8163171295247764, 0.1403307496149613920, -13.39321520033831447 ) ) ;
#42753=AXIS2_PLACEMENT_3D ( 'NONE', #9112, #19370, #33260 ) ;
#42763=CARTESIAN_POINT ( 'NONE',  ( 109.6491296295247793, -4.863998795839590272, -19.15521520033831493 ) ) ;
#42767=CARTESIAN_POINT ( 'NONE',  ( 113.1912390045248031, -9.868328341294098749, -11.32035403202665869 ) ) ;
#42773=CARTESIAN_POINT ( 'NONE',  ( 111.2465515045248168, -6.936859964151250502, -18.39754474579286025 ) ) ;
#42776=DIRECTION ( 'NONE',  ( -1.000000000000000000, 0.000000000000000000, 0.000000000000000000 ) ) ;
#42786=CARTESIAN_POINT ( 'NONE',  ( 112.8439733795247832, -1.325403438956436419, -9.854619843455211026 ) ) ;
#42789=CARTESIAN_POINT ( 'NONE',  ( 84.86020291624612355, -29.99489077589588959, -12.39321520033834645 ) ) ;
#42790=CARTESIAN_POINT ( 'NONE',  ( 109.1629577545248395, -7.250697342233347165, -7.631215200338321125 ) ) ;
#42794=CARTESIAN_POINT ( 'NONE',  ( 109.2294421281825407, -4.894246902762260376, -7.815410045176730769 ) ) ;
#42796=VECTOR ( 'NONE', #26568, 999.9999999999998863 ) ;
#42797=CARTESIAN_POINT ( 'NONE',  ( 106.5237390045248418, -9.868328341294098749, -11.32035403202665869 ) ) ;
#42798=CARTESIAN_POINT ( 'NONE',  ( 116.7565503026016813, -4.863998795840742240, -18.55532337341522364 ) ) ;
#42799=CARTESIAN_POINT ( 'NONE',  ( 83.39219417991402850, -33.04367333191778755, -22.35815310413347845 ) ) ;
#42802=CARTESIAN_POINT ( 'NONE',  ( 109.6491296295247793, -4.863998795839590272, -19.15521520033831493 ) ) ;
#42811=CARTESIAN_POINT ( 'NONE',  ( 112.8439733795247832, -8.938348069036489818, -17.46756447353520159 ) ) ;
#42818=ORIENTED_EDGE ( 'NONE', *, *, #33534, .F. ) ;
#42825=CARTESIAN_POINT ( 'NONE',  ( 64.01282776924010420, -34.86145050234441811, -5.893215200338315363 ) ) ;
#42838=CARTESIAN_POINT ( 'NONE',  ( 113.2606921295247702, -9.868328341294093420, -13.39321520033831447 ) ) ;
#42839=ADVANCED_FACE ( 'NONE', ( #40385, #37851 ), #23743, .F. ) ;
#42843=CARTESIAN_POINT ( 'NONE',  ( 116.5944421295247793, -9.868328341294093420, -13.39321520033831447 ) ) ;
#42844=B_SPLINE_CURVE_WITH_KNOTS ( 'NONE', 3,
 ( #14949, #31816, #28411, #363, #35907, #588, #42320, #42544, #7417, #14498 ),
 .UNSPECIFIED., .F., .F.,
 ( 4, 3, 3, 4 ),
 ( 0.000000000000000000, 0.0002476486447138875262, 0.0004952972925464160315, 0.0009604418836934749786 ),
 .UNSPECIFIED. ) ;
#42851=CARTESIAN_POINT ( 'NONE',  ( 108.1211608795247798, -1.325403438956436419, -16.93181055722141792 ) ) ;
#42862=CARTESIAN_POINT ( 'NONE',  ( 116.9417077545247992, -2.791137627527939813, -18.39754474579286025 ) ) ;
#42865=ORIENTED_EDGE ( 'NONE', *, *, #27960, .T. ) ;
#42877=DIRECTION ( 'NONE',  ( 0.9999995469159187467, 0.0009519285464175227711, 0.000000000000000000 ) ) ;
#42884=CARTESIAN_POINT ( 'NONE',  ( 116.7523363153857048, -5.088870560009469024, -18.55110938619918670 ) ) ;
#42892=CARTESIAN_POINT ( 'NONE',  ( 114.9275671295247889, 0.1403307496149613920, -13.39321520033831447 ) ) ;
#42893=CARTESIAN_POINT ( 'NONE',  ( 113.8163171295247764, 0.1403307496149613920, -13.39321520033831447 ) ) ;
#42901=CARTESIAN_POINT ( 'NONE',  ( 109.2295480519286883, -0.08797490772791666247, -15.21102469340631558 ) ) ;
#42904=ADVANCED_FACE ( 'NONE', ( #38075 ), #3425, .F. ) ;
#42905=CARTESIAN_POINT ( 'NONE',  ( 110.2047546295247855, -4.863998795839590272, -7.631215200338315796 ) ) ;
#42906=CARTESIAN_POINT ( 'NONE',  ( 110.1353015045248469, -6.936859964151250502, -18.39754474579286025 ) ) ;
#42925=CARTESIAN_POINT ( 'NONE',  ( 107.9128015045248219, -6.936859964151250502, -18.39754474579286025 ) ) ;
#42936=CARTESIAN_POINT ( 'NONE',  ( 62.35495919926018615, -65.08422123914256474, -45.30333471292594538 ) ) ;
#42937=CARTESIAN_POINT ( 'NONE',  ( 110.2742077545248094, -7.250697342233347165, -7.631215200338321125 ) ) ;
#42944=CARTESIAN_POINT ( 'NONE',  ( 115.8999108795247821, -8.938348069036489818, -9.318865927141430916 ) ) ;
#42945=CARTESIAN_POINT ( 'NONE',  ( 114.3024890045248156, 0.8980012041604421569, -15.77991374673208469 ) ) ;
#42949=CARTESIAN_POINT ( 'NONE',  ( 62.70685217410979106, -37.48166990149824329, -5.152479539365462990 ) ) ;
#42950=CARTESIAN_POINT ( 'NONE',  ( 105.5513952545248060, 0.8980012041604421569, -11.00651665394454071 ) ) ;
#42953=CARTESIAN_POINT ( 'NONE',  ( 107.2294421295247844, -9.051693226400931991, -21.39321520033831447 ) ) ;
#42954=DIRECTION ( 'NONE',  ( 0.000000000000000000, 0.000000000000000000, -1.000000000000000000 ) ) ;
#42957=CARTESIAN_POINT ( 'NONE',  ( 109.2294422178231201, -10.02089344363390744, -11.03051820906416403 ) ) ;
#42959=CARTESIAN_POINT ( 'NONE',  ( 113.7468640045248236, 0.1403307496149616695, -15.46607636864997204 ) ) ;
#42960=CARTESIAN_POINT ( 'NONE',  ( 106.0375671295248310, -10.62599879583958540, -13.39321520033831447 ) ) ;
#42963=CARTESIAN_POINT ( 'NONE',  ( 117.2294421295247844, 1.035107641088057973, -5.059859068394715109 ) ) ;
#42969=DIRECTION ( 'NONE',  ( 0.000000000000000000, 0.000000000000000000, 1.000000000000000000 ) ) ;
#42977=EDGE_CURVE ( 'NONE', #6307, #35850, #18803, .T. ) ;
#42978=DIRECTION ( 'NONE',  ( 0.7697712484781088493, -0.6383198453882299450, 0.000000000000000000 ) ) ;
#42980=CARTESIAN_POINT ( 'NONE',  ( 115.0664733795247798, -1.325403438956436419, -9.854619843455211026 ) ) ;
#42983=VECTOR ( 'NONE', #10310, 1000.000000000000000 ) ;
#42984=LINE ( 'NONE', #11751, #6211 ) ;
#42989=CARTESIAN_POINT ( 'NONE',  ( 109.4407702545248355, 0.1403307496149616695, -11.32035403202665336 ) ) ;
#42999=CARTESIAN_POINT ( 'NONE',  ( 111.8716296295247901, -4.863998795839590272, -8.388885654883775800 ) ) ;
#43003=CARTESIAN_POINT ( 'NONE',  ( 85.50018718514893123, -28.44542656748122056, -9.229114258165695972 ) ) ;
#43004=CARTESIAN_POINT ( 'NONE',  ( 108.2600671295247992, -10.62599879583958540, -13.39321520033831447 ) ) ;
#43011=CARTESIAN_POINT ( 'NONE',  ( 113.9552233795247815, -8.938348069036489818, -17.46756447353520159 ) ) ;
#43013=CARTESIAN_POINT ( 'NONE',  ( 83.86207143271133191, -31.76334952037468540, -22.85450806870273865 ) ) ;
#43016=CARTESIAN_POINT ( 'NONE',  ( 108.6073327545248048, -2.477300249445798297, -19.15521520033831138 ) ) ;
#43020=CARTESIAN_POINT ( 'NONE',  ( 112.3759981608379803, 0.3867979994853637526, -14.64321520033830026 ) ) ;
#43028=CARTESIAN_POINT ( 'NONE',  ( 114.7192077545248594, -7.250697342233347165, -7.631215200338321125 ) ) ;
#43031=CARTESIAN_POINT ( 'NONE',  ( 116.8221226705892803, -1.747798139657595673, -17.59079367583192166 ) ) ;
#43032=CARTESIAN_POINT ( 'NONE',  ( 117.2294421295247844, 0.6306099254434621715, -14.64321520033831447 ) ) ;
#43037=CARTESIAN_POINT ( 'NONE',  ( 76.69189222814998175, -45.49566950204133065, -7.393215200338315363 ) ) ;
#43059=CARTESIAN_POINT ( 'NONE',  ( 111.0381921295247878, -9.868328341294093420, -13.39321520033831447 ) ) ;
#43060=CARTESIAN_POINT ( 'NONE',  ( 112.4272546295247821, -4.863998795839590272, -18.39754474579285315 ) ) ;
#43061=CARTESIAN_POINT ( 'NONE',  ( 83.46705746533213244, -32.83968548964498524, -23.89321520033831803 ) ) ;
#43063=DIRECTION ( 'NONE',  ( 0.000000000000000000, -1.000000000000000000, 0.000000000000000000 ) ) ;
#43065=ORIENTED_EDGE ( 'NONE', *, *, #1924, .F. ) ;
#43070=CARTESIAN_POINT ( 'NONE',  ( 109.0935046295247872, -4.863998795839590272, -18.39754474579285315 ) ) ;
#43074=AXIS2_PLACEMENT_3D ( 'NONE', #39256, #8022, #21710 ) ;
#43078=( BOUNDED_CURVE ( )  B_SPLINE_CURVE ( 2, ( #9972, #40750, #36626, #33650, #5401, #9507, #40986, #27065, #40525, #9740, #13163, #9058, #26609, #23193, #44399, #20229, #5846 ),
 .UNSPECIFIED., .F., .T. ) 
 B_SPLINE_CURVE_WITH_KNOTS ( ( 3, 2, 2, 2, 2, 2, 2, 2, 3 ),
 ( 0.2040431156034945015, 0.2124999999999999944, 0.2250000000000000056, 0.2374999999999999889, 0.2500000000000000000, 0.2625000000000000111, 0.2750000000000000222, 0.2874999999999999778, 0.2959568843965054707 ),
 .UNSPECIFIED. ) 
 CURVE ( )  GEOMETRIC_REPRESENTATION_ITEM ( )  RATIONAL_B_SPLINE_CURVE ( ( 0.9666851417651740608, 0.9485006404992000206, 1.000000000000000000, 0.9238795325112869605, 1.000000000000000000, 0.9238795325112869605, 1.000000000000000000, 0.9238795325112869605, 1.000000000000000000, 0.9238795325112869605, 1.000000000000000000, 0.9238795325112869605, 1.000000000000000000, 0.9238795325112869605, 1.000000000000000000, 0.9485006404991980222, 0.9666851417651760592 ) ) 
 REPRESENTATION_ITEM ( '' )  );
#43079=DIRECTION ( 'NONE',  ( 0.000000000000000000, 0.000000000000000000, 1.000000000000000000 ) ) ;
#43082=CARTESIAN_POINT ( 'NONE',  ( 114.6497546295247929, -4.863998795839590272, -18.39754474579285315 ) ) ;
#43086=ORIENTED_EDGE ( 'NONE', *, *, #39235, .F. ) ;
#43090=CARTESIAN_POINT ( 'NONE',  ( 110.8992858795247827, -8.402594152722736354, -9.854619843455244776 ) ) ;
#43095=DIRECTION ( 'NONE',  ( 0.3445294493088594256, 0.9387755102040817867, 0.000000000000000000 ) ) ;
#43096=CARTESIAN_POINT ( 'NONE',  ( 115.3001676093651753, 0.5600166689815611054, -14.64321520033831447 ) ) ;
#43099=DIRECTION ( 'NONE',  ( -1.000000000000000000, 0.000000000000000000, 0.000000000000000000 ) ) ;
#43104=CARTESIAN_POINT ( 'NONE',  ( 116.6277022568074102, -9.657689035024059621, -14.93094152719381107 ) ) ;
#43110=CARTESIAN_POINT ( 'NONE',  ( 114.6497546295247929, -4.863998795839590272, -7.631215200338315796 ) ) ;
#43111=CARTESIAN_POINT ( 'NONE',  ( 112.0799890045248475, -9.868328341294098749, -11.32035403202665869 ) ) ;
#43112=CARTESIAN_POINT ( 'NONE',  ( 110.4825671295247815, 0.1403307496149613920, -13.39321520033831447 ) ) ;
#43115=ORIENTED_EDGE ( 'NONE', *, *, #23468, .F. ) ;
#43117=CARTESIAN_POINT ( 'NONE',  ( 108.6767858795247861, -0.7896495226426338832, -17.46756447353520159 ) ) ;
#43120=ADVANCED_FACE ( 'NONE', ( #44559 ), #16973, .F. ) ;
#43124=CARTESIAN_POINT ( 'NONE',  ( 112.4272546295247821, -4.863998795839590272, -7.631215200338315796 ) ) ;
#43125=CARTESIAN_POINT ( 'NONE',  ( 112.0799890045248475, -9.868328341294098749, -11.32035403202665869 ) ) ;
#43134=EDGE_LOOP ( 'NONE', ( #7242, #21498, #10260, #18237 ) ) ;
#43138=DIRECTION ( 'NONE',  ( 0.000000000000000000, 0.9284778069183718952, 0.3713878862591650232 ) ) ;
#43143=CARTESIAN_POINT ( 'NONE',  ( 116.5249890045247980, 0.8980012041604421569, -15.77991374673208469 ) ) ;
#43148=ORIENTED_EDGE ( 'NONE', *, *, #13618, .T. ) ;
#43157=CARTESIAN_POINT ( 'NONE',  ( 111.4549108795247747, -8.938348069036489818, -9.318865927141430916 ) ) ;
#43158=( BOUNDED_CURVE ( )  B_SPLINE_CURVE ( 2, ( #1520, #1970, #36174, #26150, #12026, #19536, #12256, #36844, #18855, #29347, #43707, #15441, #5613, #40518, #5839, #29796, #26378 ),
 .UNSPECIFIED., .F., .T. ) 
 B_SPLINE_CURVE_WITH_KNOTS ( ( 3, 2, 2, 2, 2, 2, 2, 2, 3 ),
 ( 0.5035091206787219997, 0.5124999999999999556, 0.5250000000000000222, 0.5374999999999999778, 0.5500000000000000444, 0.5625000000000000000, 0.5749999999999999556, 0.5875000000000000222, 0.5964908793212779781 ),
 .UNSPECIFIED. ) 
 CURVE ( )  GEOMETRIC_REPRESENTATION_ITEM ( )  RATIONAL_B_SPLINE_CURVE ( ( 0.9692594319298230010, 0.9452488050343759163, 1.000000000000000000, 0.9238795325112869605, 1.000000000000000000, 0.9238795325112869605, 1.000000000000000000, 0.9238795325112869605, 1.000000000000000000, 0.9238795325112869605, 1.000000000000000000, 0.9238795325112869605, 1.000000000000000000, 0.9238795325112869605, 1.000000000000000000, 0.9452488050343769155, 0.9692594319298230010 ) ) 
 REPRESENTATION_ITEM ( '' )  );
#43163=DIRECTION ( 'NONE',  ( -1.000000000000000000, 0.000000000000000000, 0.000000000000000000 ) ) ;
#43166=EDGE_CURVE ( 'NONE', #36261, #41199, #44111, .T. ) ;
#43168=CARTESIAN_POINT ( 'NONE',  ( 111.4549108795247747, -8.938348069036489818, -9.318865927141430916 ) ) ;
#43170=CARTESIAN_POINT ( 'NONE',  ( 116.1082702545247827, 0.1403307496149616695, -11.32035403202665336 ) ) ;
#43171=CARTESIAN_POINT ( 'NONE',  ( 113.3301452545248083, 0.8980012041604421569, -11.00651665394454071 ) ) ;
#43182=( GEOMETRIC_REPRESENTATION_CONTEXT ( 3 ) GLOBAL_UNCERTAINTY_ASSIGNED_CONTEXT ( ( #24680 ) ) GLOBAL_UNIT_ASSIGNED_CONTEXT ( ( #30518, #30073, #13207 ) ) REPRESENTATION_CONTEXT ( 'NONE', 'WORKASPACE' ) );
#43184=CARTESIAN_POINT ( 'NONE',  ( 116.9384279471258878, -11.58292435961694089, -5.930349853556944772 ) ) ;
#43186=AXIS2_PLACEMENT_3D ( 'NONE', #29293, #12657, #8767 ) ;
#43190=CARTESIAN_POINT ( 'NONE',  ( 113.6079577545248043, -2.791137627527939813, -18.39754474579286025 ) ) ;
#43191=CARTESIAN_POINT ( 'NONE',  ( 105.7597546295248350, -4.863998795839590272, -7.631215200338315796 ) ) ;
#43209=CARTESIAN_POINT ( 'NONE',  ( 112.6356140045247827, 0.1403307496149616695, -15.46607636864997204 ) ) ;
#43217=CARTESIAN_POINT ( 'NONE',  ( 108.8851452545248151, -9.868328341294098749, -15.46607636864997204 ) ) ;
#43221=CARTESIAN_POINT ( 'NONE',  ( 78.69189222814998175, -49.76310523276723785, -24.89321520033831447 ) ) ;
#43226=CARTESIAN_POINT ( 'NONE',  ( 114.8360934012278847, 0.04929351793716424401, -14.64321520033828783 ) ) ;
#43228=CARTESIAN_POINT ( 'NONE',  ( 110.4825671295247815, 0.1403307496149613920, -13.39321520033831447 ) ) ;
#43234=CARTESIAN_POINT ( 'NONE',  ( 110.1353015045248469, -2.477300249445798297, -7.631215200338321125 ) ) ;
#43241=CARTESIAN_POINT ( 'NONE',  ( 115.7610046295247912, -4.863998795839590272, -7.631215200338315796 ) ) ;
#43246=CARTESIAN_POINT ( 'NONE',  ( 108.4684265045247997, -7.250697342233347165, -19.15521520033831138 ) ) ;
#43258=CARTESIAN_POINT ( 'NONE',  ( 108.2600671295247992, -10.62599879583958540, -13.39321520033831447 ) ) ;
#43262=ORIENTED_EDGE ( 'NONE', *, *, #351, .F. ) ;
#43267=DIRECTION ( 'NONE',  ( 0.000000000000000000, 0.000000000000000000, 1.000000000000000000 ) ) ;
#43280=CARTESIAN_POINT ( 'NONE',  ( 113.6079577545248043, -2.791137627527939813, -18.39754474579286025 ) ) ;
#43282=ORIENTED_EDGE ( 'NONE', *, *, #13999, .F. ) ;
#43284=CARTESIAN_POINT ( 'NONE',  ( 113.6774108795247997, -8.938348069036489818, -9.318865927141430916 ) ) ;
#43285=CARTESIAN_POINT ( 'NONE',  ( 110.4131140045248287, 0.1403307496149616695, -15.46607636864997204 ) ) ;
#43287=VECTOR ( 'NONE', #12145, 1000.000000000000000 ) ;
#43291=CARTESIAN_POINT ( 'NONE',  ( 116.8722546295247895, -4.863998795839590272, -18.39754474579285315 ) ) ;
#43292=ORIENTED_EDGE ( 'NONE', *, *, #43498, .T. ) ;
#43298=CARTESIAN_POINT ( 'NONE',  ( 107.8433483795247838, -8.402594152722688392, -16.93181055722141792 ) ) ;
#43304=CARTESIAN_POINT ( 'NONE',  ( 70.19189222814998175, -41.58126682492877535, -29.83537093841426469 ) ) ;
#43305=CARTESIAN_POINT ( 'NONE',  ( 71.85867159647438029, -25.32195970414818476, -4.893215200338314474 ) ) ;
#43307=CARTESIAN_POINT ( 'NONE',  ( 114.5803015045248117, -6.936859964151250502, -18.39754474579286025 ) ) ;
#43338=CARTESIAN_POINT ( 'NONE',  ( 111.7327233795247849, -8.938348069036489818, -17.46756447353520159 ) ) ;
#43339=CARTESIAN_POINT ( 'NONE',  ( 108.3295202545248657, 0.1403307496149616695, -11.32035403202665336 ) ) ;
#43340=CARTESIAN_POINT ( 'NONE',  ( 111.3160046295247838, -4.863998795839590272, -18.39754474579285315 ) ) ;
#43344=CARTESIAN_POINT ( 'NONE',  ( 106.0375671295248310, -10.62599879583958540, -13.39321520033831447 ) ) ;
#43350=CARTESIAN_POINT ( 'NONE',  ( 111.2465515045248168, -2.477300249445798297, -7.631215200338321125 ) ) ;
#43351=LINE ( 'NONE', #33059, #22781 ) ;
#43361=EDGE_LOOP ( 'NONE', ( #18724, #19439, #9557, #28841, #20996, #33493 ) ) ;
#43366=ORIENTED_EDGE ( 'NONE', *, *, #23542, .T. ) ;
#43369=CARTESIAN_POINT ( 'NONE',  ( 106.4542858795248179, -8.402594152722688392, -9.854619843455216355 ) ) ;
#43374=AXIS2_PLACEMENT_3D ( 'NONE', #19512, #40031, #22702 ) ;
#43380=CARTESIAN_POINT ( 'NONE',  ( 62.16180176470561491, -65.29550861636488435, -44.87722419103883453 ) ) ;
#43382=CARTESIAN_POINT ( 'NONE',  ( 106.8710046295248759, -4.863998795839590272, -7.631215200338315796 ) ) ;
#43392=CARTESIAN_POINT ( 'NONE',  ( 111.3854577545248645, -7.250697342233347165, -7.631215200338321125 ) ) ;
#43393=CARTESIAN_POINT ( 'NONE',  ( 115.7610046295247912, -4.863998795839590272, -18.39754474579285315 ) ) ;
#43394=CARTESIAN_POINT ( 'NONE',  ( 109.9963952545248134, 0.8980012041604421569, -11.00651665394454071 ) ) ;
#43398=CARTESIAN_POINT ( 'NONE',  ( 62.88810427208139942, -37.62639143044070522, -5.060171215880807871 ) ) ;
#43403=PLANE ( 'NONE',  #41713 ) ;
#43404=EDGE_CURVE ( 'NONE', #35019, #11934, #8714, .T. ) ;
#43406=DIRECTION ( 'NONE',  ( 0.000000000000000000, 0.000000000000000000, -1.000000000000000000 ) ) ;
#43407=CARTESIAN_POINT ( 'NONE',  ( 109.2294458807338344, -10.05974036254392878, -11.12818462664568386 ) ) ;
#43410=CARTESIAN_POINT ( 'NONE',  ( 110.2742077545248094, -2.791137627527939813, -18.39754474579286025 ) ) ;
#43411=CARTESIAN_POINT ( 'NONE',  ( 115.2748327545248657, -6.936859964151250502, -8.388885654883777576 ) ) ;
#43414=CARTESIAN_POINT ( 'NONE',  ( 70.07532415883380850, -25.67919796285898926, -5.724353937072305776 ) ) ;
#43437=CARTESIAN_POINT ( 'NONE',  ( 107.7044421295247929, -9.868328341294093420, -13.39321520033831447 ) ) ;
#43438=CARTESIAN_POINT ( 'NONE',  ( 70.36267391504958368, -5.685877709920885259, -19.39321520033831447 ) ) ;
#43445=CARTESIAN_POINT ( 'NONE',  ( 111.4549108795247747, -1.325403438956436419, -16.93181055722141792 ) ) ;
#43457=CARTESIAN_POINT ( 'NONE',  ( 108.2600671295247992, 0.1403307496149613920, -13.39321520033831447 ) ) ;
#43463=CARTESIAN_POINT ( 'NONE',  ( 108.4684265045247997, -7.250697342233347165, -19.15521520033831138 ) ) ;
#43467=CARTESIAN_POINT ( 'NONE',  ( 108.7462390045248242, 0.8980012041604421569, -15.77991374673208469 ) ) ;
#43469=CARTESIAN_POINT ( 'NONE',  ( 63.69189222814998175, -37.86175736943883408, -4.893215200338314474 ) ) ;
#43472=CARTESIAN_POINT ( 'NONE',  ( 107.4960827545248350, -2.477300249445798297, -19.15521520033831138 ) ) ;
#43474=LINE ( 'NONE', #33180, #25030 ) ;
#43476=DIRECTION ( 'NONE',  ( 0.9387755102040822308, -0.3445294493088585375, 0.000000000000000000 ) ) ;
#43485=CARTESIAN_POINT ( 'NONE',  ( 111.3854577545248645, -7.250697342233347165, -7.631215200338321125 ) ) ;
#43488=CARTESIAN_POINT ( 'NONE',  ( 116.3166296295247832, -4.863998795839590272, -19.15521520033831493 ) ) ;
#43495=EDGE_CURVE ( 'NONE', #4599, #44158, #22724, .T. ) ;
#43498=EDGE_CURVE ( 'NONE', #15377, #31774, #29631, .T. ) ;
#43503=CARTESIAN_POINT ( 'NONE',  ( 116.0286950891469786, 2.331313199634366118, -19.89321520033831447 ) ) ;
#43514=CARTESIAN_POINT ( 'NONE',  ( 114.0246765045248196, -7.250697342233347165, -19.15521520033831138 ) ) ;
#43515=CARTESIAN_POINT ( 'NONE',  ( 108.0517077545248696, -2.791137627527939813, -18.39754474579286025 ) ) ;
#43516=CARTESIAN_POINT ( 'NONE',  ( 78.69189222814998175, -55.76310523276723785, -40.89321520033831092 ) ) ;
#43525=CARTESIAN_POINT ( 'NONE',  ( 109.2324108795247923, -1.325403438956436419, -16.93181055722141792 ) ) ;
#43535=CARTESIAN_POINT ( 'NONE',  ( 109.9269421295247753, -9.868328341294093420, -13.39321520033831447 ) ) ;
#43548=CARTESIAN_POINT ( 'NONE',  ( 109.5796765045248264, -2.791137627527992215, -8.388885654883745602 ) ) ;
#43550=CARTESIAN_POINT ( 'NONE',  ( 116.0286950891469786, 2.331313199634366118, -6.893215200338315363 ) ) ;
#43563=CARTESIAN_POINT ( 'NONE',  ( 110.7603796295247918, -4.863998795839590272, -19.15521520033831493 ) ) ;
#43564=CARTESIAN_POINT ( 'NONE',  ( 109.3713171295247832, 0.1403307496149613920, -13.39321520033831447 ) ) ;
#43565=CARTESIAN_POINT ( 'NONE',  ( 108.3989733795248753, -1.325403438956436419, -9.854619843455211026 ) ) ;
#43568=VERTEX_POINT ( 'NONE', #15777 ) ;
#43569=DIRECTION ( 'NONE',  ( 0.000000000000000000, -0.9284778069183718952, -0.3713878862591650232 ) ) ;
#43571=CARTESIAN_POINT ( 'NONE',  ( 143.3676850761856940, -69.76310523276724496, -16.89321520033831447 ) ) ;
#43575=CARTESIAN_POINT ( 'NONE',  ( 111.0381921295247878, 0.8980012041604618078, -13.39321520033831447 ) ) ;
#43577=EDGE_LOOP ( 'NONE', ( #37417, #35377, #16773, #28567 ) ) ;
#43578=CARTESIAN_POINT ( 'NONE',  ( 110.8551676093651821, 0.5600166689815611054, -14.64321520033834645 ) ) ;
#43586=ORIENTED_EDGE ( 'NONE', *, *, #24490, .F. ) ;
#43593=CARTESIAN_POINT ( 'NONE',  ( 112.0105358795247810, -0.7896495226426338832, -17.46756447353520159 ) ) ;
#43596=ORIENTED_EDGE ( 'NONE', *, *, #18077, .T. ) ;
#43601=EDGE_LOOP ( 'NONE', ( #5020, #10571 ) ) ;
#43604=CARTESIAN_POINT ( 'NONE',  ( 106.9404577545248145, -7.250697342233347165, -7.631215200338321125 ) ) ;
#43613=B_SPLINE_CURVE_WITH_KNOTS ( 'NONE', 3,
 ( #25547, #14381, #31922, #35101, #32373, #4332, #18484, #28970, #14157, #7306, #42430, #28074, #24646, #1140, #21224 ),
 .UNSPECIFIED., .F., .F.,
 ( 4, 2, 2, 1, 1, 1, 2, 2, 4 ),
 ( 0.000000000000000000, 0.2500000000001339484, 0.3750000000001929013, 0.4375000000002189915, 0.4687500000002216560, 0.4843750000002229883, 0.4921875000002237099, 0.5000000000002243761, 1.000000000000000000 ),
 .UNSPECIFIED. ) ;
#43615=CARTESIAN_POINT ( 'NONE',  ( 113.0523327545247838, -2.477300249445798297, -19.15521520033831138 ) ) ;
#43617=CARTESIAN_POINT ( 'NONE',  ( 110.2047546295247855, -4.863998795839590272, -7.631215200338315796 ) ) ;
#43622=CARTESIAN_POINT ( 'NONE',  ( 105.7597546295248350, -4.863998795839590272, -7.631215200338315796 ) ) ;
#43628=CARTESIAN_POINT ( 'NONE',  ( 83.82415148905927538, -46.76310523276723785, -6.893215200338315363 ) ) ;
#43629=CARTESIAN_POINT ( 'NONE',  ( 109.2294539694104287, -9.998871404483669068, -15.31448480652960242 ) ) ;
#43631=CARTESIAN_POINT ( 'NONE',  ( 112.5661608795247872, -1.325403438956436419, -16.93181055722141792 ) ) ;
#43632=CARTESIAN_POINT ( 'NONE',  ( 110.4825671295247815, 0.1403307496149613920, -13.39321520033831447 ) ) ;
#43635=DIRECTION ( 'NONE',  ( -1.000000000000000000, 0.000000000000000000, 0.000000000000000000 ) ) ;
#43636=CARTESIAN_POINT ( 'NONE',  ( 69.22226139490459218, -26.09593875132798857, -5.871463680831255694 ) ) ;
#43644=EDGE_LOOP ( 'NONE', ( #30891, #13709, #9562, #40571, #38326, #17778, #12330, #21725, #6844, #39276, #17789 ) ) ;
#43649=CARTESIAN_POINT ( 'NONE',  ( 106.1070202545248407, -10.62599879583958717, -15.77991374673208469 ) ) ;
#43652=CARTESIAN_POINT ( 'NONE',  ( 109.0240515045248202, -6.936859964151250502, -18.39754474579286025 ) ) ;
#43659=DIRECTION ( 'NONE',  ( 1.000000000000000000, 0.000000000000000000, 0.000000000000000000 ) ) ;
#43661=CARTESIAN_POINT ( 'NONE',  ( 116.7333483795247844, -8.402594152722688392, -16.93181055722141792 ) ) ;
#43662=CARTESIAN_POINT ( 'NONE',  ( 108.1906140045248037, 0.1403307496149616695, -15.46607636864997204 ) ) ;
#43666=DIRECTION ( 'NONE',  ( 1.000000000000000000, 0.000000000000000000, 0.000000000000000000 ) ) ;
#43668=CARTESIAN_POINT ( 'NONE',  ( 70.09311708302951160, -26.31909214926311691, -5.693345267502175844 ) ) ;
#43673=CARTESIAN_POINT ( 'NONE',  ( 78.69189222814998175, -69.76310523276724496, 3.106784799661685526 ) ) ;
#43674=CARTESIAN_POINT ( 'NONE',  ( 109.3713171295247832, 0.1403307496149613920, -13.39321520033831447 ) ) ;
#43678=CARTESIAN_POINT ( 'NONE',  ( 107.9822546295247889, -4.863998795839590272, -7.631215200338315796 ) ) ;
#43680=FACE_OUTER_BOUND ( 'NONE', #38006, .T. ) ;
#43681=CARTESIAN_POINT ( 'NONE',  ( 76.69189222814998175, -49.76310523276720232, -19.39321520033831447 ) ) ;
#43682=CARTESIAN_POINT ( 'NONE',  ( 111.7327233795247849, -8.938348069036489818, -17.46756447353520159 ) ) ;
#43685=CARTESIAN_POINT ( 'NONE',  ( 115.4137390045248566, 0.8980012041604421569, -15.77991374673208469 ) ) ;
#43688=CARTESIAN_POINT ( 'NONE',  ( 106.9404577545248145, -7.250697342233347165, -7.631215200338321125 ) ) ;
#43694=CARTESIAN_POINT ( 'NONE',  ( 116.1808983795247769, -1.328464889906837199, -9.857681294405580275 ) ) ;
#43704=CARTESIAN_POINT ( 'NONE',  ( 109.7185827545247889, -2.477300249445798297, -19.15521520033831138 ) ) ;
#43707=CARTESIAN_POINT ( 'NONE',  ( 110.3436608795247764, -8.938348069036489818, -9.318865927141430916 ) ) ;
#43714=EDGE_CURVE ( 'NONE', #38815, #32422, #534, .T. ) ;
#43718=B_SPLINE_CURVE_WITH_KNOTS ( 'NONE', 3,
 ( #10147, #30436, #41165, #3067, #37493, #44131, #6495, #41394, #44355, #20633 ),
 .UNSPECIFIED., .F., .F.,
 ( 4, 3, 3, 4 ),
 ( 0.000000000000000000, 0.0002476486447139085055, 0.0004952972925464399923, 0.0009604418836934780143 ),
 .UNSPECIFIED. ) ;
#43722=EDGE_CURVE ( 'NONE', #15763, #34483, #7325, .T. ) ;
#43734=CARTESIAN_POINT ( 'NONE',  ( 114.0941296295247867, -4.863998795839590272, -8.388885654883775800 ) ) ;
#43738=CARTESIAN_POINT ( 'NONE',  ( 116.5249890045247980, 0.8980012041604421569, -15.77991374673208469 ) ) ;
#43739=CARTESIAN_POINT ( 'NONE',  ( 110.2742077545248094, -2.791137627527939813, -18.39754474579286025 ) ) ;
#43742=AXIS2_PLACEMENT_3D ( 'NONE', #338, #42077, #24732 ) ;
#43744=CARTESIAN_POINT ( 'NONE',  ( 111.9410827545248708, -6.936859964151250502, -8.388885654883777576 ) ) ;
#43746=AXIS2_PLACEMENT_3D ( 'NONE', #26471, #38017, #6793 ) ;
#43747=ADVANCED_FACE ( 'NONE', ( #12479, #22281 ), #43939, .F. ) ;
#43752=EDGE_CURVE ( 'NONE', #41400, #36736, #43158, .T. ) ;
#43755=CARTESIAN_POINT ( 'NONE',  ( 105.2041296295248287, -4.863998795839590272, -8.388885654883775800 ) ) ;
#43763=CARTESIAN_POINT ( 'NONE',  ( 111.1770983795247787, -8.402594152722688392, -16.93181055722141792 ) ) ;
#43789=EDGE_CURVE ( 'NONE', #28148, #44662, #16198, .T. ) ;
#43791=VERTEX_POINT ( 'NONE', #19990 ) ;
#43793=CARTESIAN_POINT ( 'NONE',  ( 113.0523327545247838, -2.477300249445798297, -19.15521520033831138 ) ) ;
#43794=CARTESIAN_POINT ( 'NONE',  ( 109.7185827545247889, -6.936859964151250502, -8.388885654883777576 ) ) ;
#43795=CARTESIAN_POINT ( 'NONE',  ( 109.3018640045248304, 0.1403307496149616695, -15.46607636864997204 ) ) ;
#43797=CARTESIAN_POINT ( 'NONE',  ( 64.53707254195585108, -37.45440240364068529, -5.176427727597975093 ) ) ;
#43800=LINE ( 'NONE', #12565, #28900 ) ;
#43804=CARTESIAN_POINT ( 'NONE',  ( 106.1070202545248407, 0.1403307496149616695, -11.32035403202665336 ) ) ;
#43806=CARTESIAN_POINT ( 'NONE',  ( 109.7185827545247889, -2.477300249445798297, -19.15521520033831138 ) ) ;
#43807=DIRECTION ( 'NONE',  ( 1.000000000000000000, 0.000000000000000000, 0.000000000000000000 ) ) ;
#43809=DIRECTION ( 'NONE',  ( 0.9848077530122080203, -0.1736481776669309973, 0.000000000000000000 ) ) ;
#43815=FACE_OUTER_BOUND ( 'NONE', #24642, .T. ) ;
#43827=CARTESIAN_POINT ( 'NONE',  ( 111.8021765045248372, -7.250697342233347165, -19.15521520033831138 ) ) ;
#43829=ORIENTED_EDGE ( 'NONE', *, *, #44643, .T. ) ;
#43837=CARTESIAN_POINT ( 'NONE',  ( 106.2459265045248173, -7.250697342233347165, -19.15521520033831138 ) ) ;
#43844=ORIENTED_EDGE ( 'NONE', *, *, #29504, .F. ) ;
#43847=CARTESIAN_POINT ( 'NONE',  ( 83.46705746533213244, -32.83968548964498524, -23.89321520033831803 ) ) ;
#43848=CARTESIAN_POINT ( 'NONE',  ( 113.9552233795247815, -8.938348069036489818, -17.46756447353520159 ) ) ;
#43849=CARTESIAN_POINT ( 'NONE',  ( 113.3995983795247895, -8.402594152722688392, -16.93181055722141792 ) ) ;
#43850=CARTESIAN_POINT ( 'NONE',  ( 111.0381921295247878, 0.8980012041604618078, -13.39321520033831447 ) ) ;
#43852=ORIENTED_EDGE ( 'NONE', *, *, #24744, .T. ) ;
#43855=CARTESIAN_POINT ( 'NONE',  ( 107.7738952545248310, 0.8980012041604421569, -11.00651665394454071 ) ) ;
#43866=CARTESIAN_POINT ( 'NONE',  ( 111.2465515045248168, -6.936859964151250502, -18.39754474579286025 ) ) ;
#43867=CARTESIAN_POINT ( 'NONE',  ( 109.9963952545248134, -9.868328341294098749, -15.46607636864997204 ) ) ;
#43870=CARTESIAN_POINT ( 'NONE',  ( 69.20676056990819802, -25.74134712006483738, -5.871647083323465743 ) ) ;
#43885=CARTESIAN_POINT ( 'NONE',  ( 108.7462390045248242, 0.8980012041604421569, -15.77991374673208469 ) ) ;
#43889=CARTESIAN_POINT ( 'NONE',  ( 107.5655358795247736, -8.402594152722688392, -9.854619843455216355 ) ) ;
#43890=VECTOR ( 'NONE', #23572, 1000.000000000000000 ) ;
#43895=ORIENTED_EDGE ( 'NONE', *, *, #126, .T. ) ;
#43896=CARTESIAN_POINT ( 'NONE',  ( 116.3166296295247832, -4.863998795839590272, -8.388885654883775800 ) ) ;
#43902=CARTESIAN_POINT ( 'NONE',  ( 70.50211253258815702, -26.42392322955106465, -5.550474951698388892 ) ) ;
#43906=CARTESIAN_POINT ( 'NONE',  ( 110.4384831777918805, -0.01829820670803256055, -14.64321520033831447 ) ) ;
#43908=CARTESIAN_POINT ( 'NONE',  ( 111.4549108795247747, -1.325403438956436419, -16.93181055722141792 ) ) ;
#43912=CARTESIAN_POINT ( 'NONE',  ( 112.9134265045247645, -2.791137627527939813, -8.388885654883777576 ) ) ;
#43916=CARTESIAN_POINT ( 'NONE',  ( 112.4967077545247633, -7.250697342233347165, -7.631215200338321125 ) ) ;
#43918=CARTESIAN_POINT ( 'NONE',  ( 112.5661608795247872, -8.938348069036489818, -9.318865927141430916 ) ) ;
#43921=CARTESIAN_POINT ( 'NONE',  ( 105.6903015045248253, -2.477300249445798297, -7.631215200338321125 ) ) ;
#43924=ORIENTED_EDGE ( 'NONE', *, *, #30102, .T. ) ;
#43925=CARTESIAN_POINT ( 'NONE',  ( 85.56953267055843071, -21.30583187727814121, -6.893215200338315363 ) ) ;
#43926=AXIS2_PLACEMENT_3D ( 'NONE', #30747, #6579, #10232 ) ;
#43933=ORIENTED_EDGE ( 'NONE', *, *, #7456, .F. ) ;
#43936=CARTESIAN_POINT ( 'NONE',  ( 109.0935046295247872, -4.863998795839590272, -7.631215200338315796 ) ) ;
#43939=PLANE ( 'NONE',  #15803 ) ;
#43947=CARTESIAN_POINT ( 'NONE',  ( 105.0652233795248378, -1.325403438956436419, -9.854619843455211026 ) ) ;
#43949=CARTESIAN_POINT ( 'NONE',  ( 109.3272331777918822, -0.01829820670803256055, -14.64321520033831447 ) ) ;
#43960=CARTESIAN_POINT ( 'NONE',  ( 113.3995983795247895, -8.402594152722688392, -16.93181055722141792 ) ) ;
#43964=CARTESIAN_POINT ( 'NONE',  ( 112.9134265045247645, -7.250697342233347165, -19.15521520033831138 ) ) ;
#43965=CARTESIAN_POINT ( 'NONE',  ( 110.1353015045248469, -6.936859964151250502, -18.39754474579286025 ) ) ;
#43966=CARTESIAN_POINT ( 'NONE',  ( 82.61796790274630098, -31.77134309784167243, -23.02235920239622047 ) ) ;
#43970=CARTESIAN_POINT ( 'NONE',  ( 61.69189222814998175, -58.16308431783641453, -34.89321520033831092 ) ) ;
#43971=CARTESIAN_POINT ( 'NONE',  ( 112.1494421295248003, -9.868328341294093420, -13.39321520033831447 ) ) ;
#43979=CARTESIAN_POINT ( 'NONE',  ( 116.9118497693529690, -11.61451501706865308, -21.52314428506147337 ) ) ;
#43990=AXIS2_PLACEMENT_3D ( 'NONE', #26728, #33313, #16013 ) ;
#43992=CARTESIAN_POINT ( 'NONE',  ( 111.3854577545248645, -2.791137627527939813, -18.39754474579286025 ) ) ;
#44004=ADVANCED_FACE ( 'NONE', ( #32027 ), #38869, .T. ) ;
#44010=DIRECTION ( 'NONE',  ( 1.000000000000000000, 0.000000000000000000, 0.000000000000000000 ) ) ;
#44022=CARTESIAN_POINT ( 'NONE',  ( 112.6356140045247827, -10.62599879583958717, -11.00651665394454604 ) ) ;
#44023=CARTESIAN_POINT ( 'NONE',  ( 111.9410827545248708, -6.936859964151250502, -8.388885654883777576 ) ) ;
#44024=CARTESIAN_POINT ( 'NONE',  ( 108.6073327545248048, -6.936859964151250502, -8.388885654883777576 ) ) ;
#44027=ORIENTED_EDGE ( 'NONE', *, *, #30927, .F. ) ;
#44029=CARTESIAN_POINT ( 'NONE',  ( 109.2294434778830663, -7.784931826024912738, -8.490152284657904502 ) ) ;
#44032=CARTESIAN_POINT ( 'NONE',  ( 105.2735827545248810, -6.936859964151250502, -8.388885654883777576 ) ) ;
#44034=CARTESIAN_POINT ( 'NONE',  ( 115.8304577545247582, -2.791137627527939813, -18.39754474579286025 ) ) ;
#44055=CARTESIAN_POINT ( 'NONE',  ( 113.7468640045248236, -10.62599879583958717, -11.00651665394454604 ) ) ;
#44058=ORIENTED_EDGE ( 'NONE', *, *, #23804, .T. ) ;
#44065=CARTESIAN_POINT ( 'NONE',  ( 108.1211608795247798, -8.938348069036489818, -9.318865927141430916 ) ) ;
#44074=VERTEX_POINT ( 'NONE', #12195 ) ;
#44076=LINE ( 'NONE', #13060, #36558 ) ;
#44078=VECTOR ( 'NONE', #17367, 1000.000000000000000 ) ;
#44079=CARTESIAN_POINT ( 'NONE',  ( 111.8716296295247901, -4.863998795839590272, -19.15521520033831493 ) ) ;
#44080=CARTESIAN_POINT ( 'NONE',  ( 113.0523327545247838, -6.936859964151250502, -8.388885654883777576 ) ) ;
#44081=CARTESIAN_POINT ( 'NONE',  ( 112.2883483795247770, -0.7896495226426338832, -9.318865927141430916 ) ) ;
#44098=CARTESIAN_POINT ( 'NONE',  ( 108.6073327545248048, -6.936859964151250502, -8.388885654883777576 ) ) ;
#44099=CARTESIAN_POINT ( 'NONE',  ( 112.7050671295247923, 0.1403307496149613920, -13.39321520033831447 ) ) ;
#44101=CARTESIAN_POINT ( 'NONE',  ( 61.69189222814998175, -58.16308431783641453, -34.89321520033831092 ) ) ;
#44102=CARTESIAN_POINT ( 'NONE',  ( 68.68839935636917460, -25.95913848132418522, -5.893215200338315363 ) ) ;
#44111=LINE ( 'NONE', #16059, #23063 ) ;
#44116=CARTESIAN_POINT ( 'NONE',  ( 106.9404577545248145, -7.250697342233347165, -7.631215200338321125 ) ) ;
#44121=CARTESIAN_POINT ( 'NONE',  ( 108.5378796295247810, -4.863998795839590272, -8.388885654883775800 ) ) ;
#44131=CARTESIAN_POINT ( 'NONE',  ( 116.3148066399283778, 0.4261359969231631739, -14.64321520033831447 ) ) ;
#44134=CARTESIAN_POINT ( 'NONE',  ( 114.4099712410415748, 0.7607806665037644134, -12.14321520033829316 ) ) ;
#44138=ORIENTED_EDGE ( 'NONE', *, *, #25920, .F. ) ;
#44139=CARTESIAN_POINT ( 'NONE',  ( 114.3339130180080758, 0.7607806665038616689, -14.64321520033833579 ) ) ;
#44141=CARTESIAN_POINT ( 'NONE',  ( 114.7192077545248594, -7.250697342233347165, -7.631215200338321125 ) ) ;
#44145=CARTESIAN_POINT ( 'NONE',  ( 112.5661608795247872, -1.325403438956436419, -16.93181055722141792 ) ) ;
#44150=CARTESIAN_POINT ( 'NONE',  ( 112.4272546295247821, -4.863998795839590272, -7.631215200338315796 ) ) ;
#44152=CARTESIAN_POINT ( 'NONE',  ( 112.6356140045247827, -10.62599879583958717, -11.00651665394454604 ) ) ;
#44155=CARTESIAN_POINT ( 'NONE',  ( 114.6497546295247929, -4.863998795839590272, -7.631215200338315796 ) ) ;
#44158=VERTEX_POINT ( 'NONE', #30984 ) ;
#44167=( BOUNDED_CURVE ( )  B_SPLINE_CURVE ( 2, ( #8145, #8592, #40043, #22490, #18630, #4708, #43694, #36832, #36384 ),
 .UNSPECIFIED., .F., .F. ) 
 B_SPLINE_CURVE_WITH_KNOTS ( ( 3, 2, 2, 2, 3 ),
 ( 0.5030750193655179059, 0.6250000000000000000, 0.7500000000000000000, 0.8750000000000000000, 0.9595335776365219171 ),
 .UNSPECIFIED. ) 
 CURVE ( )  GEOMETRIC_REPRESENTATION_ITEM ( )  RATIONAL_B_SPLINE_CURVE ( ( 0.9963469806983950017, 0.9257521078044069762, 1.000000000000000000, 0.9238795325112869605, 1.000000000000000000, 0.9238795325112869605, 1.000000000000000000, 0.9485221164145160033, 0.9666699875272299902 ) ) 
 REPRESENTATION_ITEM ( '' )  );
#44170=CARTESIAN_POINT ( 'NONE',  ( 107.4960827545248350, -2.477300249445798297, -19.15521520033831138 ) ) ;
#44183=CARTESIAN_POINT ( 'NONE',  ( 107.1488171295248861, 0.1403307496149613920, -13.39321520033831447 ) ) ;
#44191=ORIENTED_EDGE ( 'NONE', *, *, #32152, .T. ) ;
#44194=CARTESIAN_POINT ( 'NONE',  ( 116.2471765045247594, -2.791137627527939813, -8.388885654883777576 ) ) ;
#44198=CARTESIAN_POINT ( 'NONE',  ( 110.5520202545248054, -10.62599879583958717, -15.77991374673208469 ) ) ;
#44199=CARTESIAN_POINT ( 'NONE',  ( 109.3018640045248304, 0.1403307496149616695, -15.46607636864997204 ) ) ;
#44200=CARTESIAN_POINT ( 'NONE',  ( 116.3166296295247832, -4.863998795839590272, -19.15521520033831493 ) ) ;
#44205=CARTESIAN_POINT ( 'NONE',  ( 114.6497546295247929, -4.863998795839590272, -18.39754474579285315 ) ) ;
#44223=CARTESIAN_POINT ( 'NONE',  ( 113.4690515045247992, -6.936859964151250502, -18.39754474579286025 ) ) ;
#44226=ORIENTED_EDGE ( 'NONE', *, *, #13644, .F. ) ;
#44234=DIRECTION ( 'NONE',  ( 0.000000000000000000, 0.000000000000000000, 1.000000000000000000 ) ) ;
#44235=CARTESIAN_POINT ( 'NONE',  ( 109.4154010812577837, -0.01829820670803256055, -12.14321520033831625 ) ) ;
#44241=CARTESIAN_POINT ( 'NONE',  ( 117.1500671295247713, 0.1403307496149613920, -13.39321520033831447 ) ) ;
#44251=ORIENTED_EDGE ( 'NONE', *, *, #27157, .F. ) ;
#44254=CARTESIAN_POINT ( 'NONE',  ( 113.6774108795247997, -8.938348069036489818, -9.318865927141430916 ) ) ;
#44255=CARTESIAN_POINT ( 'NONE',  ( 105.2735827545248810, -6.936859964151250502, -8.388885654883777576 ) ) ;
#44256=CARTESIAN_POINT ( 'NONE',  ( 104.9957702545248566, 0.1403307496149616695, -11.32035403202665336 ) ) ;
#44259=EDGE_LOOP ( 'NONE', ( #92, #23564, #44191, #18068 ) ) ;
#44261=DIRECTION ( 'NONE',  ( 0.000000000000000000, 0.000000000000000000, 1.000000000000000000 ) ) ;
#44265=CARTESIAN_POINT ( 'NONE',  ( 105.6208483795248299, -0.7896495226426338832, -9.318865927141430916 ) ) ;
#44266=DIRECTION ( 'NONE',  ( 0.000000000000000000, 0.000000000000000000, -1.000000000000000000 ) ) ;
#44267=ORIENTED_EDGE ( 'NONE', *, *, #33948, .F. ) ;
#44268=DIRECTION ( 'NONE',  ( -0.000000000000000000, 0.9284778069183718952, 0.3713878862591650232 ) ) ;
#44278=ORIENTED_EDGE ( 'NONE', *, *, #7486, .F. ) ;
#44287=CARTESIAN_POINT ( 'NONE',  ( 113.1217858795247935, -0.7896495226426338832, -17.46756447353520159 ) ) ;
#44293=DIRECTION ( 'NONE',  ( 0.000000000000000000, 0.000000000000000000, 1.000000000000000000 ) ) ;
#44297=CARTESIAN_POINT ( 'NONE',  ( 108.0517077545248696, -7.250697342233347165, -7.631215200338321125 ) ) ;
#44306=EDGE_CURVE ( 'NONE', #17767, #27212, #15220, .T. ) ;
#44308=CARTESIAN_POINT ( 'NONE',  ( 106.1764733795248219, -8.938348069036489818, -17.46756447353520159 ) ) ;
#44309=CARTESIAN_POINT ( 'NONE',  ( 112.2883483795247770, -8.402594152722688392, -16.93181055722141792 ) ) ;
#44310=CARTESIAN_POINT ( 'NONE',  ( 107.9128015045248219, -2.477300249445798297, -7.631215200338321125 ) ) ;
#44327=CARTESIAN_POINT ( 'NONE',  ( 106.5237390045248418, -9.868328341294098749, -11.32035403202665869 ) ) ;
#44328=CARTESIAN_POINT ( 'NONE',  ( 113.2606921295247702, -9.868328341294093420, -13.39321520033831447 ) ) ;
#44343=CARTESIAN_POINT ( 'NONE',  ( 106.6626452545248611, 0.8980012041604421569, -11.00651665394454071 ) ) ;
#44347=CARTESIAN_POINT ( 'NONE',  ( 109.3018640045248304, 0.1403307496149616695, -15.46607636864997204 ) ) ;
#44355=CARTESIAN_POINT ( 'NONE',  ( 116.0852504229301729, 0.1075849324168598464, -14.64321520033831447 ) ) ;
#44356=CARTESIAN_POINT ( 'NONE',  ( 69.69189222814998175, -41.76310523276723785, -7.393215200338315363 ) ) ;
#44358=CARTESIAN_POINT ( 'NONE',  ( 70.26514696789978132, -26.36317451685219027, -5.635745540951655030 ) ) ;
#44361=VERTEX_POINT ( 'NONE', #40063 ) ;
#44363=DIRECTION ( 'NONE',  ( 0.000000000000000000, 0.000000000000000000, -1.000000000000000000 ) ) ;
#44364=CARTESIAN_POINT ( 'NONE',  ( 114.8581140045248361, -10.62599879583958717, -11.00651665394454604 ) ) ;
#44369=CARTESIAN_POINT ( 'NONE',  ( 113.1217858795247935, -8.402594152722688392, -9.854619843455216355 ) ) ;
#44370=CARTESIAN_POINT ( 'NONE',  ( 61.69189222814998175, -66.36873802749349238, -42.40236911872441539 ) ) ;
#44373=CARTESIAN_POINT ( 'NONE',  ( 109.0935046295247872, -4.863998795839590272, -7.631215200338315796 ) ) ;
#44374=CARTESIAN_POINT ( 'NONE',  ( 61.69189222814998175, -49.76310523276723785, -7.393215200338315363 ) ) ;
#44375=CARTESIAN_POINT ( 'NONE',  ( 114.0941296295247867, -4.863998795839590272, -19.15521520033831493 ) ) ;
#44389=CARTESIAN_POINT ( 'NONE',  ( 105.7597546295248350, -4.863998795839590272, -7.631215200338315796 ) ) ;
#44390=CARTESIAN_POINT ( 'NONE',  ( 112.7745202545247878, 0.1403307496149616695, -11.32035403202665336 ) ) ;
#44391=CIRCLE ( 'NONE', #21821, 5.000000000000004441 ) ;
#44393=CARTESIAN_POINT ( 'NONE',  ( 116.8497197753081451, -0.6930611473297154657, -16.59100722635417213 ) ) ;
#44394=CARTESIAN_POINT ( 'NONE',  ( 113.2606921295247702, 0.8980012041604618078, -13.39321520033831447 ) ) ;
#44396=VECTOR ( 'NONE', #38064, 1000.000000000000000 ) ;
#44399=CARTESIAN_POINT ( 'NONE',  ( 112.8439733795247832, -1.325403438956533675, -9.854619843455175499 ) ) ;
#44403=CARTESIAN_POINT ( 'NONE',  ( 107.2182702545248105, 0.1403307496149616695, -11.32035403202665336 ) ) ;
#44404=CARTESIAN_POINT ( 'NONE',  ( 111.0884957829843813, 0.6362173239733635022, -14.64321520033831447 ) ) ;
#44417=CARTESIAN_POINT ( 'NONE',  ( 112.8439733795247832, -8.938348069036489818, -17.46756447353520159 ) ) ;
#44418=CARTESIAN_POINT ( 'NONE',  ( 105.7597546295248350, -4.863998795839590272, -18.39754474579285315 ) ) ;
#44423=CARTESIAN_POINT ( 'NONE',  ( 112.8914883310706898, 0.1843591316377651834, -12.14321520033831625 ) ) ;
#44424=CARTESIAN_POINT ( 'NONE',  ( 112.7050671295247923, 0.1403307496149613920, -13.39321520033831447 ) ) ;
#44433=CARTESIAN_POINT ( 'NONE',  ( 116.6114517406422380, -11.86984128825793228, -21.21871708423150693 ) ) ;
#44434=ORIENTED_EDGE ( 'NONE', *, *, #9214, .F. ) ;
#44444=CARTESIAN_POINT ( 'NONE',  ( 111.3160046295247838, -4.863998795839590272, -18.39754474579285315 ) ) ;
#44469=ORIENTED_EDGE ( 'NONE', *, *, #5532, .F. ) ;
#44471=CARTESIAN_POINT ( 'NONE',  ( 105.5513952545248060, 0.8980012041604421569, -11.00651665394454071 ) ) ;
#44474=CARTESIAN_POINT ( 'NONE',  ( 64.61935771200890599, -37.86087448816891765, -4.893215200338314474 ) ) ;
#44477=DIRECTION ( 'NONE',  ( -1.000000000000000000, 0.000000000000000000, 0.000000000000000000 ) ) ;
#44482=CARTESIAN_POINT ( 'NONE',  ( 106.4542858795248179, -0.7896495226426338832, -17.46756447353520159 ) ) ;
#44500=VECTOR ( 'NONE', #22791, 1000.000000000000114 ) ;
#44504=CARTESIAN_POINT ( 'NONE',  ( 111.0381921295247878, 0.8980012041604618078, -13.39321520033831447 ) ) ;
#44520=ADVANCED_FACE ( 'NONE', ( #41386 ), #23831, .T. ) ;
#44525=CARTESIAN_POINT ( 'NONE',  ( 109.5796765045248122, -7.250697342233347165, -19.15521520033831138 ) ) ;
#44527=CARTESIAN_POINT ( 'NONE',  ( 111.3160046295247838, -4.863998795839590272, -18.39754474579285315 ) ) ;
#44528=CARTESIAN_POINT ( 'NONE',  ( 106.6626452545248611, 0.8980012041604421569, -11.00651665394454071 ) ) ;
#44541=CARTESIAN_POINT ( 'NONE',  ( 105.6903015045248253, -2.477300249445798297, -7.631215200338321125 ) ) ;
#44543=CARTESIAN_POINT ( 'NONE',  ( 78.69189222814998175, -50.16718729050182191, 3.106784799661685526 ) ) ;
#44546=CARTESIAN_POINT ( 'NONE',  ( 108.3295202545248657, 0.1403307496149616695, -11.32035403202665336 ) ) ;
#44547=CARTESIAN_POINT ( 'NONE',  ( 109.6491296295247793, -4.863998795839590272, -8.388885654883775800 ) ) ;
#44552=ORIENTED_EDGE ( 'NONE', *, *, #14501, .F. ) ;
#44558=VERTEX_POINT ( 'NONE', #39283 ) ;
#44559=FACE_OUTER_BOUND ( 'NONE', #11992, .T. ) ;
#44566=DIRECTION ( 'NONE',  ( 1.000000000000000000, 0.000000000000000000, 0.000000000000000000 ) ) ;
#44569=ADVANCED_FACE ( 'NONE', ( #7144 ), #17863, .T. ) ;
#44572=CARTESIAN_POINT ( 'NONE',  ( 116.1082702545247827, -10.62599879583958717, -15.77991374673208469 ) ) ;
#44574=EDGE_CURVE ( 'NONE', #14664, #40056, #354, .T. ) ;
#44581=LINE ( 'NONE', #23371, #35284 ) ;
#44583=CARTESIAN_POINT ( 'NONE',  ( 111.6379010812576809, -0.01829820670803256055, -12.14321520033831625 ) ) ;
#44584=AXIS2_PLACEMENT_3D ( 'NONE', #13, #7078, #41530 ) ;
#44585=CARTESIAN_POINT ( 'NONE',  ( 71.37572422742091760, -11.86958442233774313, -21.39321520033831447 ) ) ;
#44592=CARTESIAN_POINT ( 'NONE',  ( 115.8999108795247821, -8.938348069036489818, -9.318865927141430916 ) ) ;
#44595=DIRECTION ( 'NONE',  ( 0.000000000000000000, 0.000000000000000000, 1.000000000000000000 ) ) ;
#44596=CARTESIAN_POINT ( 'NONE',  ( 105.5513952545248060, 0.8980012041604421569, -11.00651665394454071 ) ) ;
#44601=CARTESIAN_POINT ( 'NONE',  ( 108.5378796295247810, -4.863998795839590272, -19.15521520033831493 ) ) ;
#44603=CARTESIAN_POINT ( 'NONE',  ( 111.8021765045248372, -7.250697342233347165, -19.15521520033831138 ) ) ;
#44606=CARTESIAN_POINT ( 'NONE',  ( 115.2053796295247849, -4.863998795839590272, -19.15521520033831493 ) ) ;
#44621=CARTESIAN_POINT ( 'NONE',  ( 116.8413970861548705, -0.9790246463113243536, -16.91993411223075583 ) ) ;
#44622=CARTESIAN_POINT ( 'NONE',  ( 113.1912390045248031, 0.8980012041604421569, -15.77991374673208469 ) ) ;
#44626=CARTESIAN_POINT ( 'NONE',  ( 113.1743144685027858, 0.6938714319018670640, -14.64321520033829316 ) ) ;
#44631=CARTESIAN_POINT ( 'NONE',  ( 116.8076447119520083, 1.993636652035369217, -5.877315907535680672 ) ) ;
#44633=CARTESIAN_POINT ( 'NONE',  ( 106.1764733795248219, -1.325403438956436419, -9.854619843455211026 ) ) ;
#44634=CARTESIAN_POINT ( 'NONE',  ( 111.4548954522301898, 0.1168444861212661334, -14.64321520033828783 ) ) ;
#44637=CARTESIAN_POINT ( 'NONE',  ( 115.6662166496844861, 0.5600166689815611054, -12.14321520033831625 ) ) ;
#44643=EDGE_CURVE ( 'NONE', #41318, #20631, #1477, .T. ) ;
#44645=CARTESIAN_POINT ( 'NONE',  ( 117.1500671295247713, 0.1403307496149613920, -13.39321520033831447 ) ) ;
#44648=CARTESIAN_POINT ( 'NONE',  ( 109.6491296295247793, -4.863998795839590272, -19.15521520033831493 ) ) ;
#44650=CARTESIAN_POINT ( 'NONE',  ( 115.8999108795247821, -8.938348069036489818, -9.318865927141430916 ) ) ;
#44655=CARTESIAN_POINT ( 'NONE',  ( 109.6491296295247793, -4.863998795839590272, -8.388885654883775800 ) ) ;
#44657=DIRECTION ( 'NONE',  ( 1.000000000000000000, 0.000000000000000000, 0.000000000000000000 ) ) ;
#44662=VERTEX_POINT ( 'NONE', #14366 ) ;
#44664=CARTESIAN_POINT ( 'NONE',  ( 104.9957702545248566, 0.1403307496149616695, -11.32035403202665336 ) ) ;
#44673=CARTESIAN_POINT ( 'NONE',  ( 116.5249890045247980, 0.8980012041604421569, -15.77991374673208469 ) ) ;
#44675=DIRECTION ( 'NONE',  ( 1.000000000000000000, 0.000000000000000000, 0.000000000000000000 ) ) ;
#44679=CIRCLE ( 'NONE', #4586, 5.000000000000004441 ) ;
#44685=DIRECTION ( 'NONE',  ( 0.000000000000000000, 0.000000000000000000, -1.000000000000000000 ) ) ;
#44691=VECTOR ( 'NONE', #11126, 1000.000000000000000 ) ;
#44703=CARTESIAN_POINT ( 'NONE',  ( 108.3989733795248753, -8.938348069036489818, -17.46756447353520159 ) ) ;
#44704=CARTESIAN_POINT ( 'NONE',  ( 107.1488171295248861, 0.1403307496149613920, -13.39321520033831447 ) ) ;
#44705=CARTESIAN_POINT ( 'NONE',  ( 105.9681140045248355, 0.1403307496149616695, -15.46607636864997204 ) ) ;
#44710=CARTESIAN_POINT ( 'NONE',  ( 87.44708369096657918, -21.99489077589588604, -4.893215200338314474 ) ) ;
#44715=CARTESIAN_POINT ( 'NONE',  ( 115.2748327545248657, -6.936859964151250502, -8.388885654883777576 ) ) ;
#44728=CARTESIAN_POINT ( 'NONE',  ( 63.69189222814998175, -69.76310523276724496, -16.89321520033831447 ) ) ;
#44736=CARTESIAN_POINT ( 'NONE',  ( 108.3295202545248657, -10.62599879583958717, -15.77991374673208469 ) ) ;
#44743=CIRCLE ( 'NONE', #24330, 5.000000000000004441 ) ;
#44746=ADVANCED_FACE ( 'NONE', ( #3865 ), #7742, .T. ) ;
#44756=CARTESIAN_POINT ( 'NONE',  ( 106.5931921295248372, 0.8980012041604618078, -13.39321520033831447 ) ) ;
#44757=CARTESIAN_POINT ( 'NONE',  ( 113.6079577545248043, -2.791137627527939813, -18.39754474579286025 ) ) ;
#44758=CARTESIAN_POINT ( 'NONE',  ( 105.6208483795248299, -0.7896495226426338832, -9.318865927141430916 ) ) ;
#44763=CARTESIAN_POINT ( 'NONE',  ( 111.7327233795247849, -8.938348069036489818, -17.46756447353520159 ) ) ;
#44765=DIRECTION ( 'NONE',  ( 0.000000000000000000, 0.000000000000000000, -1.000000000000000000 ) ) ;
#44771=CARTESIAN_POINT ( 'NONE',  ( 115.8304577545247582, -2.791137627527939813, -18.39754474579286025 ) ) ;
#44777=CARTESIAN_POINT ( 'NONE',  ( 106.1070202545248407, 0.1403307496149616695, -11.32035403202665336 ) ) ;
#44778=CARTESIAN_POINT ( 'NONE',  ( 107.2877233795247776, -1.325403438956436419, -9.854619843455211026 ) ) ;
#44782=ORIENTED_EDGE ( 'NONE', *, *, #15267, .F. ) ;
#44783=AXIS2_PLACEMENT_3D ( 'NONE', #31207, #45129, #9805 ) ;
#44787=EDGE_LOOP ( 'NONE', ( #2972, #10368, #43924, #28071, #34972, #3567, #25385 ) ) ;
#44798=CARTESIAN_POINT ( 'NONE',  ( 114.0246765045248196, -7.250697342233347165, -19.15521520033831138 ) ) ;
#44805=CIRCLE ( 'NONE', #41164, 2.999999999999998224 ) ;
#44808=CARTESIAN_POINT ( 'NONE',  ( 112.8439733795247832, -8.938348069036441856, -17.46756447353520514 ) ) ;
#44810=CARTESIAN_POINT ( 'NONE',  ( 64.69075612292361654, -36.94291761115415795, -5.470407532193525491 ) ) ;
#44813=ORIENTED_EDGE ( 'NONE', *, *, #4400, .T. ) ;
#44816=CARTESIAN_POINT ( 'NONE',  ( 114.2330358795247776, -0.7896495226426338832, -17.46756447353520159 ) ) ;
#44820=CARTESIAN_POINT ( 'NONE',  ( 69.69189222814998175, -41.76310523276723785, -47.71602681600972318 ) ) ;
#44821=CARTESIAN_POINT ( 'NONE',  ( 114.3024890045248156, -9.868328341294098749, -11.32035403202665869 ) ) ;
#44825=CARTESIAN_POINT ( 'NONE',  ( 106.1070202545248407, -10.62599879583958717, -15.77991374673208469 ) ) ;
#44827=CARTESIAN_POINT ( 'NONE',  ( 109.8574890045247940, 0.8980012041604421569, -15.77991374673208469 ) ) ;
#44830=DIRECTION ( 'NONE',  ( 1.000000000000000000, 0.000000000000000000, 0.000000000000000000 ) ) ;
#44834=ORIENTED_EDGE ( 'NONE', *, *, #29504, .T. ) ;
#44843=EDGE_CURVE ( 'NONE', #36736, #4599, #40678, .T. ) ;
#44847=CIRCLE ( 'NONE', #1133, 6.132259260909266985 ) ;
#44851=CARTESIAN_POINT ( 'NONE',  ( 114.8581140045248361, -10.62599879583958717, -11.00651665394454604 ) ) ;
#44854=DIRECTION ( 'NONE',  ( -1.000000000000000000, -1.697309329729404623E-15, 0.000000000000000000 ) ) ;
#44855=CARTESIAN_POINT ( 'NONE',  ( 116.2471765045247594, -2.791137627527939813, -8.388885654883777576 ) ) ;
#44857=CARTESIAN_POINT ( 'NONE',  ( 116.7920406659710864, 2.007758018742032302, -5.899424721369208591 ) ) ;
#44859=CARTESIAN_POINT ( 'NONE',  ( 107.3571765045248299, -2.791137627527939813, -8.388885654883777576 ) ) ;
#44863=CARTESIAN_POINT ( 'NONE',  ( 115.5212212410415873, 0.7607806665037644134, -12.14321520033829493 ) ) ;
#44873=CARTESIAN_POINT ( 'NONE',  ( 110.8298327545248299, -2.477300249445798297, -19.15521520033831138 ) ) ;
#44875=CARTESIAN_POINT ( 'NONE',  ( 115.2053796295247849, -4.863998795839590272, -19.15521520033831493 ) ) ;
#44881=CARTESIAN_POINT ( 'NONE',  ( 109.1629577545248395, -2.791137627527939813, -18.39754474579286025 ) ) ;
#44898=CARTESIAN_POINT ( 'NONE',  ( 116.0388171295248014, -10.62599879583958540, -13.39321520033831447 ) ) ;
#44908=CARTESIAN_POINT ( 'NONE',  ( 107.0793640045248196, 0.1403307496149616695, -15.46607636864997204 ) ) ;
#44910=CARTESIAN_POINT ( 'NONE',  ( 85.75809888461174069, -18.45227461768569199, -21.89321520033831447 ) ) ;
#44926=CARTESIAN_POINT ( 'NONE',  ( 107.5655358795247736, -0.7896495226426338832, -17.46756447353520159 ) ) ;
#44936=ADVANCED_FACE ( 'NONE', ( #17565 ), #227, .T. ) ;
#44937=AXIS2_PLACEMENT_3D ( 'NONE', #37129, #20729, #30985 ) ;
#44939=CARTESIAN_POINT ( 'NONE',  ( 106.3848327545248651, -2.477300249445798297, -19.15521520033831138 ) ) ;
#44941=VERTEX_POINT ( 'NONE', #40334 ) ;
#44950=ORIENTED_EDGE ( 'NONE', *, *, #42977, .T. ) ;
#44952=ADVANCED_FACE ( 'NONE', ( #23233 ), #19132, .T. ) ;
#44956=EDGE_LOOP ( 'NONE', ( #34433, #20991, #30838, #25282 ) ) ;
#44960=CARTESIAN_POINT ( 'NONE',  ( 109.5102233795247884, -8.938348069036489818, -17.46756447353520159 ) ) ;
#44967=VECTOR ( 'NONE', #9748, 1000.000000000000114 ) ;
#44971=DIRECTION ( 'NONE',  ( 0.000000000000000000, 0.000000000000000000, -1.000000000000000000 ) ) ;
#44977=ORIENTED_EDGE ( 'NONE', *, *, #22011, .T. ) ;
#44980=CARTESIAN_POINT ( 'NONE',  ( 110.2742077545248094, -7.250697342233347165, -7.631215200338321125 ) ) ;
#44981=CARTESIAN_POINT ( 'NONE',  ( 110.4825671295247815, 0.1403307496149613920, -13.39321520033831447 ) ) ;
#44982=CARTESIAN_POINT ( 'NONE',  ( 106.5237390045248418, 0.8980012041604421569, -15.77991374673208469 ) ) ;
#44987=CARTESIAN_POINT ( 'NONE',  ( 112.0799890045248475, 0.8980012041604421569, -15.77991374673208469 ) ) ;
#44991=DIRECTION ( 'NONE',  ( 1.000000000000000000, 1.671245155169139691E-16, 0.000000000000000000 ) ) ;
#44994=CARTESIAN_POINT ( 'NONE',  ( 107.5655358795247736, -0.7896495226426338832, -17.46756447353520159 ) ) ;
#44999=CARTESIAN_POINT ( 'NONE',  ( 116.4555358795247884, -0.7896495226426338832, -17.46756447353520159 ) ) ;
#45000=CARTESIAN_POINT ( 'NONE',  ( 108.9545983795247821, -8.402594152722688392, -16.93181055722141792 ) ) ;
#45018=ORIENTED_EDGE ( 'NONE', *, *, #25431, .F. ) ;
#45021=CARTESIAN_POINT ( 'NONE',  ( 113.6079577545248043, -7.250697342233347165, -7.631215200338321125 ) ) ;
#45029=CARTESIAN_POINT ( 'NONE',  ( 86.04230958663551121, -25.82262605124140364, -8.393215200338314474 ) ) ;
#45030=DIRECTION ( 'NONE',  ( 1.000000000000000000, 0.000000000000000000, 0.000000000000000000 ) ) ;
#45033=ORIENTED_EDGE ( 'NONE', *, *, #43789, .F. ) ;
#45036=CARTESIAN_POINT ( 'NONE',  ( 107.6349890045248401, -9.868328341294098749, -11.32035403202665869 ) ) ;
#45040=CARTESIAN_POINT ( 'NONE',  ( 112.4967077545247633, -2.791137627527887410, -18.39754474579284249 ) ) ;
#45041=CARTESIAN_POINT ( 'NONE',  ( 111.2465515045248168, -6.936859964151250502, -18.39754474579286025 ) ) ;
#45042=CARTESIAN_POINT ( 'NONE',  ( 111.2465515045248168, -2.477300249445798297, -7.631215200338310467 ) ) ;
#45045=CARTESIAN_POINT ( 'NONE',  ( 105.9681140045248355, -10.62599879583958717, -11.00651665394454604 ) ) ;
#45048=CARTESIAN_POINT ( 'NONE',  ( 109.3713171295247832, -10.62599879583958540, -13.39321520033831447 ) ) ;
#45062=CARTESIAN_POINT ( 'NONE',  ( 116.8382249924907086, -1.095796847231273130, -17.04019780263804762 ) ) ;
#45063=CARTESIAN_POINT ( 'NONE',  ( 115.2748327545248657, -2.477300249445798297, -19.15521520033831138 ) ) ;
#45064=ORIENTED_EDGE ( 'NONE', *, *, #35159, .F. ) ;
#45067=DIRECTION ( 'NONE',  ( 0.000000000000000000, 0.000000000000000000, -1.000000000000000000 ) ) ;
#45072=CARTESIAN_POINT ( 'NONE',  ( 69.69189222814998175, -41.76310523276723785, -6.393215200338315363 ) ) ;
#45073=CARTESIAN_POINT ( 'NONE',  ( 115.4831921295247952, -9.868328341294093420, -13.39321520033831447 ) ) ;
#45078=B_SPLINE_CURVE_WITH_KNOTS ( 'NONE', 3,
 ( #28932, #11600, #25510, #22088, #4747, #18667, #43966, #13412, #20021, #24120, #26633, #40546, #19563, #38014, #9993, #26858, #3136, #41009, #34136, #33904, #12730, #2219, #9763, #33440, #16149, #30053, #23674, #10212, #27088, #37094, #9529, #23445, #27316, #9307 ),
 .UNSPECIFIED., .F., .F.,
 ( 4, 2, 2, 2, 2, 2, 1, 1, 2, 2, 2, 2, 1, 1, 2, 2, 2, 2, 4 ),
 ( 0.000000000000000000, 0.06249999999997646327, 0.09374999999996487532, 0.1249999999999532874, 0.1874999999999158173, 0.2187499999998893940, 0.2343749999998761824, 0.2421874999998695766, 0.2460937499998662736, 0.2499999999998629707, 0.3749999999998242517, 0.4374999999998063216, 0.4687499999997993272, 0.4843749999998045452, 0.4921874999997982725, 0.4999999999997919997, 0.6249999999998440137, 0.7499999999998959721, 1.000000000000000000 ),
 .UNSPECIFIED. ) ;
#45085=( BOUNDED_SURFACE ( )  B_SPLINE_SURFACE ( 1, 2, ( 
 ( #11280, #27941, #41851, #21082, #21535, #35653, #38616, #24728, #31565, #32009, #28610, #10611, #18116, #35422, #14696, #34747, #42519, #4427, #7393, #11509, #21311, #1007, #31340, #38399, #28379, #25188, #39086, #114, #42292, #17892, #14027, #7855, #14923, #28834, #11054, #42744, #25413, #34959, #3747, #334, #14247, #1891, #1233, #12638, #36102, #19459, #25852, #39758, #15593, #42959, #22877, #43190, #5542, #33122, #1449, #36771, #1670, #18566, #15819, #11954, #15145, #8528, #4644, #32680, #2115, #32458, #43631, #33342, #16045, #18791, #26306, #19008, #22430, #35873, #8082, #29951, #26534, #29052, #15370, #19239, #21984, #26078, #29274, #11726, #39543, #43866, #36323, #25640, #8304, #22653, #29718, #8979, #22206, #29496, #4873, #12405, #32894, #36549, #5092, #43410, #12177, #39982, #40214, #8747, #5323, #23578, #3038, #24025, #10122, #40904, #13086, #16278, #12863, #37694, #33571, #13759, #9658, #30180, #16734, #34038, #30630, #41366, #19919, #44098, #16960, #6467, #37222, #44546, #30854, #23337, #37914, #6691, #26763, #37460, #6233, #20155, #2576, #16506, #13310, #20603, #40672, #2807, #9424, #34478, #23806, #3257, #17182, #2347, #5996, #27217, #33805, #30405, #31072, #44327, #26984, #41135, #20377, #9894, #34263, #44777, #13536 ),
 ( #27444, #40444, #44999, #9206, #23115, #36992, #5762, #19683, #17839, #3484, #27668, #31736, #62, #41581, #24677, #38565, #42016, #20818, #24244, #10340, #17400, #6908, #3699, #506, #10781, #28112, #3920, #31289, #13975, #27888, #7341, #14417, #21036, #7125, #41802, #21260, #35140, #10560, #28327, #38137, #34697, #24457, #38349, #34909, #17619, #31512, #284, #14194, #28439, #14526, #20927, #18170, #14080, #39374, #35248, #41903, #42352, #11111, #25013, #21815, #390, #10668, #42571, #32067, #17723, #38906, #11334, #3797, #4484, #35708, #24571, #4025, #31846, #615, #28221, #42128, #7677, #32297, #7227, #21592, #35017, #1062, #4253, #18405, #28890, #27998, #38456, #35479, #21141, #31621, #14977, #14303, #10888, #835, #14754, #24787, #17947, #28667, #25245, #39143, #42802, #38679, #11563, #7908, #25470, #34801, #7445, #3585, #21365, #17496, #31395, #164, #25914, #39819, #15651, #43016, #22935, #43246, #5597, #33177, #1507, #36828, #1729, #18624, #15880, #12012, #15201, #8586, #4704, #32733, #29555, #43472, #9038, #15427, #29105, #29777, #19299, #4927, #12238, #43688, #36158, #19521, #33398, #11785, #22486, #19068, #32952, #29332, #36380, #26135, #2172, #39599, #40039, #22264, #16102, #36607, #30005, #43921, #1289, #25692, #8805 ) ),
 .UNSPECIFIED., .F., .F., .T. ) 
 B_SPLINE_SURFACE_WITH_KNOTS ( ( 2, 2 ),
 ( 3, 2, 2, 2, 2, 2, 2, 2, 2, 2, 2, 2, 2, 2, 2, 2, 2, 2, 2, 2, 2, 2, 2, 2, 2, 2, 2, 2, 2, 2, 2, 2, 2, 2, 2, 2, 2, 2, 2, 2, 2, 2, 2, 2, 2, 2, 2, 2, 2, 2, 2, 2, 2, 2, 2, 2, 2, 2, 2, 2, 2, 2, 2, 2, 2, 2, 2, 2, 2, 2, 2, 2, 2, 2, 2, 2, 2, 2, 2, 2, 3 ),
 ( 0.000000000000000000, 1.000000000000000000 ),
 ( 0.000000000000000000, 0.01250000000000000069, 0.02500000000000000139, 0.03749999999999999861, 0.05000000000000000278, 0.06250000000000000000, 0.07499999999999999722, 0.08749999999999999445, 0.1000000000000000056, 0.1125000000000000028, 0.1250000000000000000, 0.1375000000000000111, 0.1499999999999999944, 0.1625000000000000056, 0.1749999999999999889, 0.1875000000000000000, 0.2000000000000000111, 0.2124999999999999944, 0.2250000000000000056, 0.2374999999999999889, 0.2500000000000000000, 0.2625000000000000111, 0.2750000000000000222, 0.2874999999999999778, 0.2999999999999999889, 0.3125000000000000000, 0.3250000000000000111, 0.3375000000000000222, 0.3499999999999999778, 0.3624999999999999889, 0.3750000000000000000, 0.3875000000000000111, 0.4000000000000000222, 0.4124999999999999778, 0.4249999999999999889, 0.4375000000000000000, 0.4500000000000000111, 0.4625000000000000222, 0.4749999999999999778, 0.4874999999999999889, 0.5000000000000000000, 0.5124999999999999556, 0.5250000000000000222, 0.5374999999999999778, 0.5500000000000000444, 0.5625000000000000000, 0.5749999999999999556, 0.5875000000000000222, 0.5999999999999999778, 0.6125000000000000444, 0.6250000000000000000, 0.6374999999999999556, 0.6500000000000000222, 0.6624999999999999778, 0.6750000000000000444, 0.6875000000000000000, 0.6999999999999999556, 0.7125000000000000222, 0.7249999999999999778, 0.7375000000000000444, 0.7500000000000000000, 0.7624999999999999556, 0.7750000000000000222, 0.7874999999999999778, 0.8000000000000000444, 0.8125000000000000000, 0.8249999999999999556, 0.8375000000000000222, 0.8499999999999999778, 0.8625000000000000444, 0.8750000000000000000, 0.8874999999999999556, 0.9000000000000000222, 0.9124999999999999778, 0.9250000000000000444, 0.9375000000000000000, 0.9499999999999999556, 0.9625000000000000222, 0.9749999999999999778, 0.9875000000000000444, 1.000000000000000000 ),
 .UNSPECIFIED. ) 
 GEOMETRIC_REPRESENTATION_ITEM ( )  RATIONAL_B_SPLINE_SURFACE ( (
 ( 1.000000000000000000, 0.9238795325112869605, 1.000000000000000000, 0.9238795325112869605, 1.000000000000000000, 0.9238795325112869605, 1.000000000000000000, 0.9238795325112869605, 1.000000000000000000, 0.9238795325112869605, 1.000000000000000000, 0.9238795325112869605, 1.000000000000000000, 0.9238795325112869605, 1.000000000000000000, 0.9238795325112869605, 1.000000000000000000, 0.9238795325112869605, 1.000000000000000000, 0.9238795325112869605, 1.000000000000000000, 0.9238795325112869605, 1.000000000000000000, 0.9238795325112869605, 1.000000000000000000, 0.9238795325112869605, 1.000000000000000000, 0.9238795325112869605, 1.000000000000000000, 0.9238795325112869605, 1.000000000000000000, 0.9238795325112869605, 1.000000000000000000, 0.9238795325112869605, 1.000000000000000000, 0.9238795325112869605, 1.000000000000000000, 0.9238795325112869605, 1.000000000000000000, 0.9238795325112869605, 1.000000000000000000, 0.9238795325112869605, 1.000000000000000000, 0.9238795325112869605, 1.000000000000000000, 0.9238795325112869605, 1.000000000000000000, 0.9238795325112869605, 1.000000000000000000, 0.9238795325112869605, 1.000000000000000000, 0.9238795325112869605, 1.000000000000000000, 0.9238795325112869605, 1.000000000000000000, 0.9238795325112869605, 1.000000000000000000, 0.9238795325112869605, 1.000000000000000000, 0.9238795325112869605, 1.000000000000000000, 0.9238795325112869605, 1.000000000000000000, 0.9238795325112869605, 1.000000000000000000, 0.9238795325112869605, 1.000000000000000000, 0.9238795325112869605, 1.000000000000000000, 0.9238795325112869605, 1.000000000000000000, 0.9238795325112869605, 1.000000000000000000, 0.9238795325112869605, 1.000000000000000000, 0.9238795325112869605, 1.000000000000000000, 0.9238795325112869605, 1.000000000000000000, 0.9238795325112869605, 1.000000000000000000, 0.9238795325112869605, 1.000000000000000000, 0.9238795325112869605, 1.000000000000000000, 0.9238795325112869605, 1.000000000000000000, 0.9238795325112869605, 1.000000000000000000, 0.9238795325112869605, 1.000000000000000000, 0.9238795325112869605, 1.000000000000000000, 0.9238795325112869605, 1.000000000000000000, 0.9238795325112869605, 1.000000000000000000, 0.9238795325112869605, 1.000000000000000000, 0.9238795325112869605, 1.000000000000000000, 0.9238795325112869605, 1.000000000000000000, 0.9238795325112869605, 1.000000000000000000, 0.9238795325112869605, 1.000000000000000000, 0.9238795325112869605, 1.000000000000000000, 0.9238795325112869605, 1.000000000000000000, 0.9238795325112869605, 1.000000000000000000, 0.9238795325112869605, 1.000000000000000000, 0.9238795325112869605, 1.000000000000000000, 0.9238795325112869605, 1.000000000000000000, 0.9238795325112869605, 1.000000000000000000, 0.9238795325112869605, 1.000000000000000000, 0.9238795325112869605, 1.000000000000000000, 0.9238795325112869605, 1.000000000000000000, 0.9238795325112869605, 1.000000000000000000, 0.9238795325112869605, 1.000000000000000000, 0.9238795325112869605, 1.000000000000000000, 0.9238795325112869605, 1.000000000000000000, 0.9238795325112869605, 1.000000000000000000, 0.9238795325112869605, 1.000000000000000000, 0.9238795325112869605, 1.000000000000000000, 0.9238795325112869605, 1.000000000000000000, 0.9238795325112869605, 1.000000000000000000, 0.9238795325112869605, 1.000000000000000000, 0.9238795325112869605, 1.000000000000000000, 0.9238795325112869605, 1.000000000000000000, 0.9238795325112869605, 1.000000000000000000, 0.9238795325112869605, 1.000000000000000000, 0.9238795325112869605, 1.000000000000000000, 0.9238795325112869605, 1.000000000000000000, 0.9238795325112869605, 1.000000000000000000),
 ( 1.000000000000000000, 0.9238795325112869605, 1.000000000000000000, 0.9238795325112869605, 1.000000000000000000, 0.9238795325112869605, 1.000000000000000000, 0.9238795325112869605, 1.000000000000000000, 0.9238795325112869605, 1.000000000000000000, 0.9238795325112869605, 1.000000000000000000, 0.9238795325112869605, 1.000000000000000000, 0.9238795325112869605, 1.000000000000000000, 0.9238795325112869605, 1.000000000000000000, 0.9238795325112869605, 1.000000000000000000, 0.9238795325112869605, 1.000000000000000000, 0.9238795325112869605, 1.000000000000000000, 0.9238795325112869605, 1.000000000000000000, 0.9238795325112869605, 1.000000000000000000, 0.9238795325112869605, 1.000000000000000000, 0.9238795325112869605, 1.000000000000000000, 0.9238795325112869605, 1.000000000000000000, 0.9238795325112869605, 1.000000000000000000, 0.9238795325112869605, 1.000000000000000000, 0.9238795325112869605, 1.000000000000000000, 0.9238795325112869605, 1.000000000000000000, 0.9238795325112869605, 1.000000000000000000, 0.9238795325112869605, 1.000000000000000000, 0.9238795325112869605, 1.000000000000000000, 0.9238795325112869605, 1.000000000000000000, 0.9238795325112869605, 1.000000000000000000, 0.9238795325112869605, 1.000000000000000000, 0.9238795325112869605, 1.000000000000000000, 0.9238795325112869605, 1.000000000000000000, 0.9238795325112869605, 1.000000000000000000, 0.9238795325112869605, 1.000000000000000000, 0.9238795325112869605, 1.000000000000000000, 0.9238795325112869605, 1.000000000000000000, 0.9238795325112869605, 1.000000000000000000, 0.9238795325112869605, 1.000000000000000000, 0.9238795325112869605, 1.000000000000000000, 0.9238795325112869605, 1.000000000000000000, 0.9238795325112869605, 1.000000000000000000, 0.9238795325112869605, 1.000000000000000000, 0.9238795325112869605, 1.000000000000000000, 0.9238795325112869605, 1.000000000000000000, 0.9238795325112869605, 1.000000000000000000, 0.9238795325112869605, 1.000000000000000000, 0.9238795325112869605, 1.000000000000000000, 0.9238795325112869605, 1.000000000000000000, 0.9238795325112869605, 1.000000000000000000, 0.9238795325112869605, 1.000000000000000000, 0.9238795325112869605, 1.000000000000000000, 0.9238795325112869605, 1.000000000000000000, 0.9238795325112869605, 1.000000000000000000, 0.9238795325112869605, 1.000000000000000000, 0.9238795325112869605, 1.000000000000000000, 0.9238795325112869605, 1.000000000000000000, 0.9238795325112869605, 1.000000000000000000, 0.9238795325112869605, 1.000000000000000000, 0.9238795325112869605, 1.000000000000000000, 0.9238795325112869605, 1.000000000000000000, 0.9238795325112869605, 1.000000000000000000, 0.9238795325112869605, 1.000000000000000000, 0.9238795325112869605, 1.000000000000000000, 0.9238795325112869605, 1.000000000000000000, 0.9238795325112869605, 1.000000000000000000, 0.9238795325112869605, 1.000000000000000000, 0.9238795325112869605, 1.000000000000000000, 0.9238795325112869605, 1.000000000000000000, 0.9238795325112869605, 1.000000000000000000, 0.9238795325112869605, 1.000000000000000000, 0.9238795325112869605, 1.000000000000000000, 0.9238795325112869605, 1.000000000000000000, 0.9238795325112869605, 1.000000000000000000, 0.9238795325112869605, 1.000000000000000000, 0.9238795325112869605, 1.000000000000000000, 0.9238795325112869605, 1.000000000000000000, 0.9238795325112869605, 1.000000000000000000, 0.9238795325112869605, 1.000000000000000000, 0.9238795325112869605, 1.000000000000000000, 0.9238795325112869605, 1.000000000000000000, 0.9238795325112869605, 1.000000000000000000, 0.9238795325112869605, 1.000000000000000000, 0.9238795325112869605, 1.000000000000000000) ) ) 
 REPRESENTATION_ITEM ( '' )  SURFACE ( )  );
#45089=CARTESIAN_POINT ( 'NONE',  ( 110.2742077545248094, -7.250697342233347165, -7.631215200338321125 ) ) ;
#45090=CARTESIAN_POINT ( 'NONE',  ( 106.1070202545248407, 0.1403307496149616695, -11.32035403202665336 ) ) ;
#45091=CARTESIAN_POINT ( 'NONE',  ( 113.3995983795247895, -0.7896495226426338832, -9.318865927141430916 ) ) ;
#45096=CARTESIAN_POINT ( 'NONE',  ( 110.4131140045248287, 0.1403307496149616695, -15.46607636864997204 ) ) ;
#45100=LINE ( 'NONE', #13857, #11898 ) ;
#45109=VECTOR ( 'NONE', #42060, 1000.000000000000000 ) ;
#45112=EDGE_CURVE ( 'NONE', #36034, #16480, #2019, .T. ) ;
#45113=CARTESIAN_POINT ( 'NONE',  ( 107.1488171295247867, 0.1403307496149613920, -13.39321520033831447 ) ) ;
#45122=ORIENTED_EDGE ( 'NONE', *, *, #39925, .F. ) ;
#45123=CARTESIAN_POINT ( 'NONE',  ( 114.1635827545248389, -2.477300249445798297, -19.15521520033831138 ) ) ;
#45129=DIRECTION ( 'NONE',  ( 3.317300593186674996E-33, -1.668003342285379964E-16, 1.000000000000000000 ) ) ;
#45130=ADVANCED_FACE ( 'NONE', ( #23000 ), #24860, .T. ) ;
#45135=EDGE_CURVE ( 'NONE', #31317, #35799, #7510, .T. ) ;
#45139=EDGE_CURVE ( 'NONE', #6063, #38699, #23809, .T. ) ;
#45143=CARTESIAN_POINT ( 'NONE',  ( 105.6208483795248299, -0.7896495226426338832, -9.318865927141430916 ) ) ;
#45147=CARTESIAN_POINT ( 'NONE',  ( 113.3954021944299768, 0.6269505268395592079, -12.14321520033829849 ) ) ;
#45156=COLOUR_RGB('Dark Blue',0.08,0.2,0.34);
#45157=FILL_AREA_STYLE_COLOUR('',#45156);
#45158=FILL_AREA_STYLE('',(#45157));
#45159=SURFACE_STYLE_FILL_AREA(#45158);
#45160=SURFACE_SIDE_STYLE('',(#45159));
#45161=SURFACE_STYLE_USAGE(.BOTH.,#45160);
#45162=PRESENTATION_STYLE_ASSIGNMENT((#45161));
ENDSEC;
END-ISO-10303-21;
